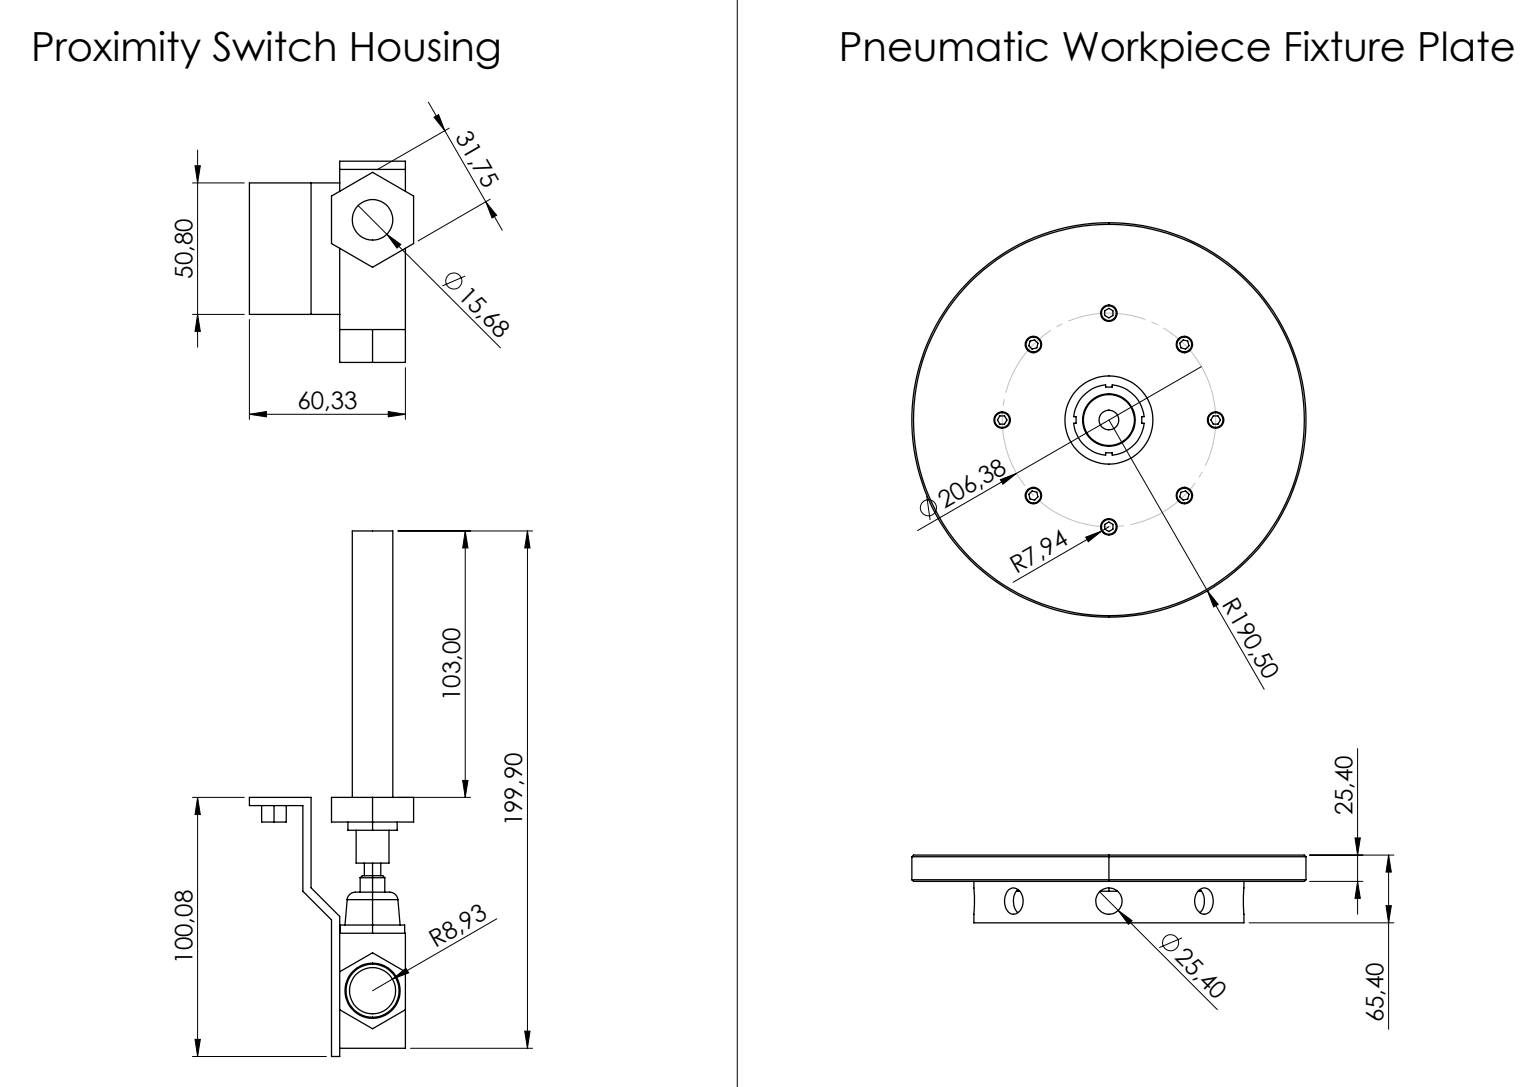
ISO-10303-21;
HEADER;
FILE_DESCRIPTION (('STEP AP214'),
    '1' );
FILE_NAME ('Pneumatic Workpiece Fixture Plate.step',
    '2026-10-07T11:37:37',
    ( '' ),
    ( '' ),
    'SwSTEP 2.0',
    'SolidWorks 2020',
    '' );
FILE_SCHEMA (( 'AUTOMOTIVE_DESIGN' ));
ENDSEC;

DATA;
#3=CARTESIAN_POINT ( 'NONE',  ( -7.205548786489490269E-13, 127.0000000000000000, 111.1250000000000000 ) ) ;
#11=CARTESIAN_POINT ( 'NONE',  ( 92.31685958143638970, 83.38015080693119785, -74.38497350661467067 ) ) ;
#32=DIRECTION ( 'NONE',  ( 0.2588190451025215166, 0.000000000000000000, -0.9659258262890680902 ) ) ;
#49=ORIENTED_EDGE ( 'NONE', *, *, #34842, .F. ) ;
#61=EDGE_LOOP ( 'NONE', ( #69387, #53740 ) ) ;
#64=ADVANCED_FACE ( 'NONE', ( #72976, #57557 ), #58012, .F. ) ;
#66=ADVANCED_FACE ( 'NONE', ( #65279 ), #44369, .F. ) ;
#91=CARTESIAN_POINT ( 'NONE',  ( -90.24991642302028083, 70.17656663518272353, 94.33976020835999066 ) ) ;
#105=CARTESIAN_POINT ( 'NONE',  ( -3.968750000000754508, 127.0000000000000000, 100.8961411191535973 ) ) ;
#110=CARTESIAN_POINT ( 'NONE',  ( -84.20430400022949868, 76.20343663217360586, -99.77245543246449699 ) ) ;
#111=CARTESIAN_POINT ( 'NONE',  ( -91.81710919847694186, 87.03046781249439334, -75.00112839233729289 ) ) ;
#127=CIRCLE ( 'NONE', #16099, 7.143750000000004263 ) ;
#165=PLANE ( 'NONE',  #8255 ) ;
#167=CARTESIAN_POINT ( 'NONE',  ( -103.1875000000000000, 127.0000000000000000, -1.080832317973422076E-12 ) ) ;
#168=DIRECTION ( 'NONE',  ( 0.000000000000000000, 1.000000000000000000, 0.000000000000000000 ) ) ;
#201=ORIENTED_EDGE ( 'NONE', *, *, #40061, .T. ) ;
#217=CARTESIAN_POINT ( 'NONE',  ( 9.720633968232110273E-16, 127.0000000000000000, -111.1250000000000000 ) ) ;
#218=FACE_OUTER_BOUND ( 'NONE', #6817, .T. ) ;
#237=VECTOR ( 'NONE', #41224, 1000.000000000000114 ) ;
#238=EDGE_CURVE ( 'NONE', #48773, #70137, #68413, .T. ) ;
#253=CARTESIAN_POINT ( 'NONE',  ( 129.9447564289581010, 80.89704698943971550, 12.61967231918858445 ) ) ;
#268=CYLINDRICAL_SURFACE ( 'NONE', #55688, 7.143750000000004263 ) ;
#316=CARTESIAN_POINT ( 'NONE',  ( 89.95943163722039060, 94.84315624882769669, 94.61941200740749025 ) ) ;
#327=AXIS2_PLACEMENT_3D ( 'NONE', #13933, #74815, #67998 ) ;
#328=VECTOR ( 'NONE', #6728, 1000.000000000000114 ) ;
#333=ORIENTED_EDGE ( 'NONE', *, *, #85560, .F. ) ;
#366=DIRECTION ( 'NONE',  ( 0.000000000000000000, 1.000000000000000000, 0.000000000000000000 ) ) ;
#370=ADVANCED_FACE ( 'NONE', ( #49293, #62029 ), #15244, .T. ) ;
#376=FACE_BOUND ( 'NONE', #32605, .T. ) ;
#387=ORIENTED_EDGE ( 'NONE', *, *, #40134, .F. ) ;
#391=CARTESIAN_POINT ( 'NONE',  ( -12.70000000000000107, 82.54999999999999716, 117.8738102209307641 ) ) ;
#428=CARTESIAN_POINT ( 'NONE',  ( -92.26493792250037984, 84.21376545118704371, 74.44936585838431142 ) ) ;
#431=ADVANCED_FACE ( 'NONE', ( #81897 ), #67340, .F. ) ;
#435=CARTESIAN_POINT ( 'NONE',  ( 85.00925061400988625, 69.93366089391891194, -82.64146475440696804 ) ) ;
#492=CARTESIAN_POINT ( 'NONE',  ( -75.10852726169378002, 77.68452076096561143, -91.72954497613109481 ) ) ;
#501=ORIENTED_EDGE ( 'NONE', *, *, #4272, .F. ) ;
#504=CARTESIAN_POINT ( 'NONE',  ( 85.31568053864954493, 74.16976894168004719, -98.82395782888116287 ) ) ;
#513=LINE ( 'NONE', #48640, #59500 ) ;
#514=CARTESIAN_POINT ( 'NONE',  ( 0.000000000000000000, 117.4749999999999943, -103.1875000000000000 ) ) ;
#520=FACE_OUTER_BOUND ( 'NONE', #29437, .T. ) ;
#547=ORIENTED_EDGE ( 'NONE', *, *, #56743, .F. ) ;
#575=CARTESIAN_POINT ( 'NONE',  ( -7.941868552260229762E-13, 127.0000000000000000, 107.7702177616926065 ) ) ;
#586=DIRECTION ( 'NONE',  ( -0.8660254037844381525, 0.000000000000000000, -0.5000000000000007772 ) ) ;
#607=CARTESIAN_POINT ( 'NONE',  ( -7.746062721843856025, 92.64813751154241572, 130.3278237768880672 ) ) ;
#621=CARTESIAN_POINT ( 'NONE',  ( 129.9528072873947053, 84.62817240485476589, 12.53569626682358695 ) ) ;
#634=CARTESIAN_POINT ( 'NONE',  ( -80.88709205069390862, 70.52090377575432001, 86.67734222162562219 ) ) ;
#657=CARTESIAN_POINT ( 'NONE',  ( -97.63858630140161665, 92.64237678566784950, -86.67213519546656642 ) ) ;
#673=ORIENTED_EDGE ( 'NONE', *, *, #65969, .T. ) ;
#678=CARTESIAN_POINT ( 'NONE',  ( 72.96458098368650269, 127.0000000000000000, 65.02708098368729850 ) ) ;
#698=ORIENTED_EDGE ( 'NONE', *, *, #71843, .F. ) ;
#711=CARTESIAN_POINT ( 'NONE',  ( 103.1875000000000000, 127.0000000000000000, -7.937499999999639400 ) ) ;
#717=CARTESIAN_POINT ( 'NONE',  ( 103.1875000000000000, 117.4749999999999943, 7.937500000000360600 ) ) ;
#740=ORIENTED_EDGE ( 'NONE', *, *, #36493, .T. ) ;
#755=ADVANCED_FACE ( 'NONE', ( #10935 ), #56167, .T. ) ;
#762=CARTESIAN_POINT ( 'NONE',  ( 85.30153658290296903, 90.93932679090998761, 98.83759631548571178 ) ) ;
#765=CYLINDRICAL_SURFACE ( 'NONE', #44229, 34.13125000000000142 ) ;
#769=EDGE_CURVE ( 'NONE', #62133, #32868, #1079, .T. ) ;
#785=ORIENTED_EDGE ( 'NONE', *, *, #8187, .F. ) ;
#789=CARTESIAN_POINT ( 'NONE',  ( 1.145694247088684285E-22, 95.25000000000000000, 118.5560000000000116 ) ) ;
#827=FACE_OUTER_BOUND ( 'NONE', #18181, .T. ) ;
#841=CARTESIAN_POINT ( 'NONE',  ( 100.8594679592200833, 82.54999999999999716, 82.89895571708400723 ) ) ;
#847=EDGE_LOOP ( 'NONE', ( #47913, #48812, #20485, #2433, #41329, #27512, #86444, #59413, #54279, #89920 ) ) ;
#871=DIRECTION ( 'NONE',  ( 0.7071067811865461294, 0.000000000000000000, 0.7071067811865489050 ) ) ;
#875=PLANE ( 'NONE',  #44348 ) ;
#880=CARTESIAN_POINT ( 'NONE',  ( -79.76397050720386517, 93.94641470820118911, 87.71185091857950056 ) ) ;
#883=ADVANCED_FACE ( 'NONE', ( #13270 ), #75941, .F. ) ;
#886=CARTESIAN_POINT ( 'NONE',  ( -118.0434137139726118, 88.91291927174616205, 11.02232302911455264 ) ) ;
#889=CARTESIAN_POINT ( 'NONE',  ( 74.70173812346097009, 79.26437155269050550, -92.06079644778149884 ) ) ;
#892=DIRECTION ( 'NONE',  ( -3.491483361109385222E-15, 0.000000000000000000, 1.000000000000000000 ) ) ;
#901=CARTESIAN_POINT ( 'NONE',  ( -3.968750000000770051, 127.0000000000000000, 105.4788588808462038 ) ) ;
#905=CARTESIAN_POINT ( 'NONE',  ( 76.80574412431069220, 90.93089219781636245, -90.31319802837579402 ) ) ;
#937=DIRECTION ( 'NONE',  ( 0.000000000000000000, 0.000000000000000000, 1.000000000000000000 ) ) ;
#945=CARTESIAN_POINT ( 'NONE',  ( -76.79083731950203173, 74.16215221268210200, -90.32738470895317562 ) ) ;
#951=CARTESIAN_POINT ( 'NONE',  ( 0.000000000000000000, 111.1250000000000000, 0.000000000000000000 ) ) ;
#954=ORIENTED_EDGE ( 'NONE', *, *, #47098, .T. ) ;
#957=CARTESIAN_POINT ( 'NONE',  ( 87.44698480207823366, 71.76234181793741129, -96.94335780202294472 ) ) ;
#968=CIRCLE ( 'NONE', #16988, 7.143750000000004263 ) ;
#972=CARTESIAN_POINT ( 'NONE',  ( 97.46300000000010755, 82.54999999999999716, -12.69999999999898144 ) ) ;
#985=CARTESIAN_POINT ( 'NONE',  ( -93.49502539975199511, 69.93364840292896645, 91.12742965731035838 ) ) ;
#996=CYLINDRICAL_SURFACE ( 'NONE', #75479, 7.143749999999999822 ) ;
#1018=B_SPLINE_CURVE_WITH_KNOTS ( 'NONE', 3,
 ( #43540, #14059, #62654, #428, #76288, #35382, #57168, #8604, #77636, #56725, #28117, #43086, #41741, #71282, #64450, #70369, #55805, #83560, #36302, #48997, #42634, #21786, #63552, #64010, #70829, #1788, #14519, #22685, #36751, #29485, #35836, #880, #2231, #56264, #29040, #21326, #84471, #50355, #29941, #1338, #42197, #69928, #8145, #84011, #77195, #22234, #69478, #78094, #57625 ),
 .UNSPECIFIED., .F., .F.,
 ( 4, 2, 2, 2, 2, 2, 2, 2, 2, 2, 2, 2, 2, 2, 2, 1, 2, 2, 2, 2, 2, 2, 2, 2, 4 ),
 ( 0.01987186023414422645, 0.02111356671950567407, 0.02235527320486711822, 0.02483868617559002040, 0.02608039266095149578, 0.02732209914631297809, 0.02980551211703592190, 0.03228892508775886572, 0.03353063157312033415, 0.03477233805848178871, 0.03725575102920469783, 0.03849745751456615239, 0.03973916399992760695, 0.04222257697065050913, 0.04346428345601198451, 0.04470598994137346682, 0.04594769642673494914, 0.04718940291209643145, 0.04967281588281940996, 0.05091452236818086452, 0.05215622885354231908, 0.05463964182426526983, 0.05588134830962676602, 0.05712305479498826222, 0.05960646776571128236 ),
 .UNSPECIFIED. ) ;
#1028=ORIENTED_EDGE ( 'NONE', *, *, #76526, .F. ) ;
#1034=ORIENTED_EDGE ( 'NONE', *, *, #40096, .F. ) ;
#1036=DIRECTION ( 'NONE',  ( 0.2588190451025180749, 0.000000000000000000, -0.9659258262890690894 ) ) ;
#1042=VECTOR ( 'NONE', #24862, 1000.000000000000000 ) ;
#1053=ORIENTED_EDGE ( 'NONE', *, *, #85400, .T. ) ;
#1056=DIRECTION ( 'NONE',  ( 0.000000000000000000, -1.000000000000000000, 0.000000000000000000 ) ) ;
#1063=CARTESIAN_POINT ( 'NONE',  ( 12.53573128184445551, 84.62794568765841063, -117.8914214560859932 ) ) ;
#1064=CARTESIAN_POINT ( 'NONE',  ( -12.70000000000000107, 82.54999999999999716, 129.9368274816650910 ) ) ;
#1065=CARTESIAN_POINT ( 'NONE',  ( -3.174999999999644995, 104.3431970271541616, -33.98325472291465132 ) ) ;
#1079=CIRCLE ( 'NONE', #5432, 7.143750000000001599 ) ;
#1082=DIRECTION ( 'NONE',  ( 0.000000000000000000, 1.000000000000000000, 0.000000000000000000 ) ) ;
#1094=CARTESIAN_POINT ( 'NONE',  ( -85.00925061400930360, 69.93366089391888352, 82.64146475440757911 ) ) ;
#1104=CARTESIAN_POINT ( 'NONE',  ( -76.20505178924449297, 127.0000000000000000, 76.20505178924310030 ) ) ;
#1118=CARTESIAN_POINT ( 'NONE',  ( -96.94208673522986430, 93.33885111288434189, -87.44839512528828607 ) ) ;
#1130=ORIENTED_EDGE ( 'NONE', *, *, #23416, .T. ) ;
#1158=LINE ( 'NONE', #36120, #6583 ) ;
#1159=PLANE ( 'NONE',  #88725 ) ;
#1165=AXIS2_PLACEMENT_3D ( 'NONE', #18310, #30611, #59188 ) ;
#1168=EDGE_CURVE ( 'NONE', #65321, #37445, #68012, .T. ) ;
#1178=DIRECTION ( 'NONE',  ( -0.000000000000000000, 1.000000000000000000, 0.000000000000000000 ) ) ;
#1181=DIRECTION ( 'NONE',  ( 0.000000000000000000, -1.000000000000000000, 0.000000000000000000 ) ) ;
#1201=EDGE_LOOP ( 'NONE', ( #30232, #45202 ) ) ;
#1213=EDGE_CURVE ( 'NONE', #59215, #59751, #18967, .T. ) ;
#1220=ORIENTED_EDGE ( 'NONE', *, *, #26232, .F. ) ;
#1222=CARTESIAN_POINT ( 'NONE',  ( 0.000000000000000000, 101.5999999999999943, 0.000000000000000000 ) ) ;
#1225=CARTESIAN_POINT ( 'NONE',  ( 97.63858630140103401, 92.64237678566784950, 86.67213519546724854 ) ) ;
#1241=VERTEX_POINT ( 'NONE', #61630 ) ;
#1245=EDGE_LOOP ( 'NONE', ( #56958, #54258, #46238, #1220 ) ) ;
#1251=ORIENTED_EDGE ( 'NONE', *, *, #68598, .T. ) ;
#1254=ORIENTED_EDGE ( 'NONE', *, *, #34297, .F. ) ;
#1326=DIRECTION ( 'NONE',  ( -0.7071067811865487940, 0.000000000000000000, 0.7071067811865463515 ) ) ;
#1327=EDGE_CURVE ( 'NONE', #9843, #1981, #60064, .T. ) ;
#1332=FACE_BOUND ( 'NONE', #25903, .T. ) ;
#1335=AXIS2_PLACEMENT_3D ( 'NONE', #83746, #42825, #63746 ) ;
#1338=CARTESIAN_POINT ( 'NONE',  ( -76.20774946062844890, 89.94786999841842601, 90.81826664112044512 ) ) ;
#1341=CARTESIAN_POINT ( 'NONE',  ( -117.8827734314469069, 84.21498941703525531, 12.61757617297219802 ) ) ;
#1344=CARTESIAN_POINT ( 'NONE',  ( 81.46681417397508085, 70.27900073646854651, -86.13269706310863683 ) ) ;
#1381=EDGE_LOOP ( 'NONE', ( #14389, #45601, #45690, #35665 ) ) ;
#1414=EDGE_CURVE ( 'NONE', #50785, #8401, #18401, .T. ) ;
#1416=CARTESIAN_POINT ( 'NONE',  ( 93.49502539975264881, 69.93364840292898066, -91.12742965730970468 ) ) ;
#1417=CARTESIAN_POINT ( 'NONE',  ( 0.000000000000000000, 61.59999999999999432, 130.5560000000000116 ) ) ;
#1434=ORIENTED_EDGE ( 'NONE', *, *, #81091, .F. ) ;
#1452=CARTESIAN_POINT ( 'NONE',  ( 3.175000000000355094, 111.1250000000000000, -33.98325472291460159 ) ) ;
#1466=CARTESIAN_POINT ( 'NONE',  ( -83.54193218351851158, 95.25015226514365452, -84.12159398442685188 ) ) ;
#1488=ORIENTED_EDGE ( 'NONE', *, *, #52165, .T. ) ;
#1494=EDGE_CURVE ( 'NONE', #29444, #6827, #10263, .T. ) ;
#1499=CARTESIAN_POINT ( 'NONE',  ( -12.70000000000000107, 82.54999999999999716, 129.9368274816650910 ) ) ;
#1501=ORIENTED_EDGE ( 'NONE', *, *, #74747, .T. ) ;
#1519=CARTESIAN_POINT ( 'NONE',  ( 69.72411017813010403, 120.6499999999999915, -69.72411017812979139 ) ) ;
#1525=DIRECTION ( 'NONE',  ( -1.047445008332813989E-14, 0.000000000000000000, 1.000000000000000000 ) ) ;
#1566=CARTESIAN_POINT ( 'NONE',  ( -100.8961411191535973, 127.0000000000000000, 3.968749999998880451 ) ) ;
#1592=LINE ( 'NONE', #8403, #57970 ) ;
#1606=VECTOR ( 'NONE', #41005, 1000.000000000000114 ) ;
#1610=ADVANCED_FACE ( 'NONE', ( #39738 ), #81397, .T. ) ;
#1621=EDGE_CURVE ( 'NONE', #77970, #1241, #49387, .T. ) ;
#1635=CYLINDRICAL_SURFACE ( 'NONE', #36468, 12.70000000000000107 ) ;
#1657=DIRECTION ( 'NONE',  ( -0.7071067811865510144, 0.000000000000000000, 0.7071067811865441310 ) ) ;
#1659=ORIENTED_EDGE ( 'NONE', *, *, #58078, .F. ) ;
#1670=VERTEX_POINT ( 'NONE', #2002 ) ;
#1676=CARTESIAN_POINT ( 'NONE',  ( 98.60478223830740774, 127.0000000000000000, 3.859079674607175002E-13 ) ) ;
#1677=CARTESIAN_POINT ( 'NONE',  ( 82.89895571708159139, 82.96445444011520465, 100.8594679592221155 ) ) ;
#1683=LINE ( 'NONE', #15759, #75101 ) ;
#1685=CARTESIAN_POINT ( 'NONE',  ( 76.20505178924339873, 120.6499999999999915, 76.20505178924419454 ) ) ;
#1691=ORIENTED_EDGE ( 'NONE', *, *, #2750, .F. ) ;
#1702=ORIENTED_EDGE ( 'NONE', *, *, #76963, .T. ) ;
#1704=VERTEX_POINT ( 'NONE', #84243 ) ;
#1724=ORIENTED_EDGE ( 'NONE', *, *, #1621, .T. ) ;
#1725=DIRECTION ( 'NONE',  ( -3.491483361109380094E-15, 0.000000000000000000, 1.000000000000000000 ) ) ;
#1734=FACE_BOUND ( 'NONE', #62684, .T. ) ;
#1751=CARTESIAN_POINT ( 'NONE',  ( -7.205548786489490269E-13, 101.5999999999999943, 103.1875000000000000 ) ) ;
#1764=CARTESIAN_POINT ( 'NONE',  ( 90.65754775987920766, 74.81620433377381119, 76.39898589339244950 ) ) ;
#1765=PLANE ( 'NONE',  #84930 ) ;
#1766=ADVANCED_FACE ( 'NONE', ( #83332 ), #76511, .F. ) ;
#1782=ORIENTED_EDGE ( 'NONE', *, *, #57519, .F. ) ;
#1786=ORIENTED_EDGE ( 'NONE', *, *, #238, .F. ) ;
#1788=CARTESIAN_POINT ( 'NONE',  ( -83.24211534968669923, 95.24969287062863543, 84.42134122279109931 ) ) ;
#1794=VERTEX_POINT ( 'NONE', #76962 ) ;
#1813=CARTESIAN_POINT ( 'NONE',  ( 72.96458098368701428, 101.5999999999999943, -78.00648098368678518 ) ) ;
#1817=ORIENTED_EDGE ( 'NONE', *, *, #32049, .F. ) ;
#1828=AXIS2_PLACEMENT_3D ( 'NONE', #54145, #81016, #19216 ) ;
#1850=CARTESIAN_POINT ( 'NONE',  ( 72.96458098368701428, 117.4749999999999943, -65.02708098368670164 ) ) ;
#1856=CARTESIAN_POINT ( 'NONE',  ( -103.1875000000000000, 127.0000000000000000, -1.080832317973422076E-12 ) ) ;
#1872=FACE_BOUND ( 'NONE', #82136, .T. ) ;
#1887=ORIENTED_EDGE ( 'NONE', *, *, #8187, .T. ) ;
#1895=AXIS2_PLACEMENT_3D ( 'NONE', #16774, #79005, #44455 ) ;
#1915=ORIENTED_EDGE ( 'NONE', *, *, #61465, .T. ) ;
#1945=ORIENTED_EDGE ( 'NONE', *, *, #81206, .T. ) ;
#1946=EDGE_CURVE ( 'NONE', #1794, #35668, #24234, .T. ) ;
#1954=FACE_BOUND ( 'NONE', #72816, .T. ) ;
#1967=CARTESIAN_POINT ( 'NONE',  ( -10.78734560828563360, 89.26522093196130925, 130.1097824653510315 ) ) ;
#1981=VERTEX_POINT ( 'NONE', #16527 ) ;
#2002=CARTESIAN_POINT ( 'NONE',  ( 4.665904304751420031E-15, 92.07499999999998863, -38.10000000000000142 ) ) ;
#2015=CARTESIAN_POINT ( 'NONE',  ( 1.668880554893940493, 69.93234144696143062, 130.5479136978233896 ) ) ;
#2023=CIRCLE ( 'NONE', #41097, 38.10000000000000142 ) ;
#2033=CARTESIAN_POINT ( 'NONE',  ( -103.1875000000000000, 117.4749999999999943, -1.080832317973422076E-12 ) ) ;
#2043=EDGE_LOOP ( 'NONE', ( #68408, #37115, #73877, #16147 ) ) ;
#2059=CARTESIAN_POINT ( 'NONE',  ( -130.4793906290846621, 70.66229531820916065, -4.488385961153167791 ) ) ;
#2062=VERTEX_POINT ( 'NONE', #26903 ) ;
#2090=PLANE ( 'NONE',  #6152 ) ;
#2098=DIRECTION ( 'NONE',  ( 0.000000000000000000, 1.000000000000000000, 0.000000000000000000 ) ) ;
#2102=LINE ( 'NONE', #28917, #67367 ) ;
#2124=EDGE_CURVE ( 'NONE', #47880, #64107, #46324, .T. ) ;
#2161=FACE_BOUND ( 'NONE', #29161, .T. ) ;
#2166=ORIENTED_EDGE ( 'NONE', *, *, #69271, .T. ) ;
#2184=VECTOR ( 'NONE', #82406, 1000.000000000000114 ) ;
#2192=LINE ( 'NONE', #83973, #66848 ) ;
#2221=EDGE_CURVE ( 'NONE', #55274, #46818, #44913, .T. ) ;
#2231=CARTESIAN_POINT ( 'NONE',  ( -79.21949419058834962, 93.55466788070657458, 88.20392011030202184 ) ) ;
#2249=VECTOR ( 'NONE', #61719, 1000.000000000000000 ) ;
#2290=FACE_OUTER_BOUND ( 'NONE', #53030, .T. ) ;
#2305=CARTESIAN_POINT ( 'NONE',  ( 0.000000000000000000, 127.0000000000000000, 0.000000000000000000 ) ) ;
#2315=CARTESIAN_POINT ( 'NONE',  ( 0.000000000000000000, 117.4749999999999943, -98.14560000000000173 ) ) ;
#2330=LINE ( 'NONE', #23675, #16717 ) ;
#2338=ADVANCED_FACE ( 'NONE', ( #56834 ), #996, .T. ) ;
#2352=EDGE_CURVE ( 'NONE', #18286, #38056, #51216, .T. ) ;
#2354=DIRECTION ( 'NONE',  ( 0.000000000000000000, 1.000000000000000000, 0.000000000000000000 ) ) ;
#2365=ORIENTED_EDGE ( 'NONE', *, *, #71733, .T. ) ;
#2387=CARTESIAN_POINT ( 'NONE',  ( 76.20505178924389611, 120.6499999999999915, -76.20505178924359768 ) ) ;
#2389=ADVANCED_FACE ( 'NONE', ( #87244 ), #10927, .F. ) ;
#2396=VERTEX_POINT ( 'NONE', #53574 ) ;
#2424=CARTESIAN_POINT ( 'NONE',  ( 0.000000000000000000, 127.0000000000000000, 0.000000000000000000 ) ) ;
#2431=VERTEX_POINT ( 'NONE', #19529 ) ;
#2432=LINE ( 'NONE', #50105, #73729 ) ;
#2433=ORIENTED_EDGE ( 'NONE', *, *, #81943, .F. ) ;
#2442=EDGE_CURVE ( 'NONE', #6249, #50785, #59903, .T. ) ;
#2444=CARTESIAN_POINT ( 'NONE',  ( -7.199374239792870816E-13, 101.5999999999999943, 98.14560000000000173 ) ) ;
#2453=DIRECTION ( 'NONE',  ( 0.000000000000000000, 1.000000000000000000, 0.000000000000000000 ) ) ;
#2455=DIRECTION ( 'NONE',  ( 0.000000000000000000, -1.000000000000000000, 0.000000000000000000 ) ) ;
#2456=CARTESIAN_POINT ( 'NONE',  ( -72.96458098368600531, 127.0000000000000000, -67.92268098368781182 ) ) ;
#2486=ORIENTED_EDGE ( 'NONE', *, *, #31297, .F. ) ;
#2487=AXIS2_PLACEMENT_3D ( 'NONE', #78848, #86101, #15719 ) ;
#2507=CARTESIAN_POINT ( 'NONE',  ( -130.2871811975775813, 72.98383416765817344, 8.394281761909056172 ) ) ;
#2514=EDGE_CURVE ( 'NONE', #12810, #44525, #54917, .T. ) ;
#2544=VERTEX_POINT ( 'NONE', #49909 ) ;
#2552=CARTESIAN_POINT ( 'NONE',  ( -12.70000000000000107, 82.54999999999999716, -129.9368274816650910 ) ) ;
#2564=AXIS2_PLACEMENT_3D ( 'NONE', #83197, #46395, #47297 ) ;
#2589=CARTESIAN_POINT ( 'NONE',  ( -72.96458098368600531, 117.4749999999999943, -72.96458098368781009 ) ) ;
#2596=VECTOR ( 'NONE', #70871, 1000.000000000000114 ) ;
#2609=FACE_BOUND ( 'NONE', #21078, .T. ) ;
#2611=DIRECTION ( 'NONE',  ( 1.000000000000000000, 0.000000000000000000, 0.000000000000000000 ) ) ;
#2615=CARTESIAN_POINT ( 'NONE',  ( -7.205548786489490269E-13, 127.0000000000000000, 103.1875000000000000 ) ) ;
#2616=VERTEX_POINT ( 'NONE', #86241 ) ;
#2623=ADVANCED_FACE ( 'NONE', ( #24020 ), #36754, .T. ) ;
#2631=CARTESIAN_POINT ( 'NONE',  ( 74.15067561874209900, 120.6499999999999915, 68.53801554307469246 ) ) ;
#2664=CARTESIAN_POINT ( 'NONE',  ( 75.68572508987453773, 76.20320268897035021, 91.25368348339081592 ) ) ;
#2679=ADVANCED_FACE ( 'NONE', ( #53006 ), #52128, .F. ) ;
#2684=DIRECTION ( 'NONE',  ( 0.000000000000000000, 0.000000000000000000, -1.000000000000000000 ) ) ;
#2698=EDGE_CURVE ( 'NONE', #82109, #43994, #17645, .T. ) ;
#2725=LINE ( 'NONE', #42681, #24433 ) ;
#2743=ORIENTED_EDGE ( 'NONE', *, *, #61260, .F. ) ;
#2750=EDGE_CURVE ( 'NONE', #52484, #27146, #59495, .T. ) ;
#2766=CARTESIAN_POINT ( 'NONE',  ( 99.76704648670056486, 88.91113633199481114, -84.21071524772746386 ) ) ;
#2768=VECTOR ( 'NONE', #53000, 1000.000000000000000 ) ;
#2788=EDGE_LOOP ( 'NONE', ( #36538, #22888, #1028, #17291 ) ) ;
#2794=CARTESIAN_POINT ( 'NONE',  ( -96.94152442043684914, 93.33921197991993779, 87.44900557253197348 ) ) ;
#2798=DIRECTION ( 'NONE',  ( 0.000000000000000000, 1.000000000000000000, 0.000000000000000000 ) ) ;
#2812=ORIENTED_EDGE ( 'NONE', *, *, #86456, .T. ) ;
#2816=VERTEX_POINT ( 'NONE', #13071 ) ;
#2831=LINE ( 'NONE', #35997, #27075 ) ;
#2841=CARTESIAN_POINT ( 'NONE',  ( -2.883802008152356322, 70.17481864577712258, 130.5247784292598112 ) ) ;
#2846=ORIENTED_EDGE ( 'NONE', *, *, #21323, .F. ) ;
#2849=DIRECTION ( 'NONE',  ( 0.000000000000000000, 1.000000000000000000, 0.000000000000000000 ) ) ;
#2902=CARTESIAN_POINT ( 'NONE',  ( 118.1268077877470830, 74.81620433377382540, -10.08232578576091854 ) ) ;
#2905=DIRECTION ( 'NONE',  ( 0.000000000000000000, -0.7071067811865280328, -0.7071067811865670016 ) ) ;
#2948=CARTESIAN_POINT ( 'NONE',  ( -130.3273007233323142, 72.45841406287408404, 7.755409066832052112 ) ) ;
#2970=ORIENTED_EDGE ( 'NONE', *, *, #89696, .F. ) ;
#2988=CARTESIAN_POINT ( 'NONE',  ( -11.89044713366393680, 87.03112570152840988, -130.0135071244502853 ) ) ;
#2992=AXIS2_PLACEMENT_3D ( 'NONE', #72250, #50897, #44516 ) ;
#2999=EDGE_LOOP ( 'NONE', ( #63002, #56856, #5047, #17409, #54291, #77223, #34139, #34652, #30607, #29751, #12971, #71726, #7525, #26455, #29483, #22789 ) ) ;
#3002=CARTESIAN_POINT ( 'NONE',  ( 0.000000000000000000, 101.5999999999999943, -103.1875000000000000 ) ) ;
#3009=CARTESIAN_POINT ( 'NONE',  ( 74.38497350661437224, 83.38015080693121206, 92.31685958143667392 ) ) ;
#3012=CARTESIAN_POINT ( 'NONE',  ( 7.752238106858494682, 92.64409645872694909, 130.3274943305225122 ) ) ;
#3016=ADVANCED_FACE ( 'NONE', ( #3796, #52787 ), #80554, .F. ) ;
#3019=VECTOR ( 'NONE', #47360, 1000.000000000000000 ) ;
#3025=VECTOR ( 'NONE', #19725, 1000.000000000000000 ) ;
#3027=EDGE_LOOP ( 'NONE', ( #48707, #4492, #67828, #78131, #34277, #73610 ) ) ;
#3056=VERTEX_POINT ( 'NONE', #66910 ) ;
#3072=CIRCLE ( 'NONE', #33470, 42.54500000000000171 ) ;
#3098=CARTESIAN_POINT ( 'NONE',  ( -69.72411017813060141, 120.6499999999999915, 69.72411017812929401 ) ) ;
#3101=CARTESIAN_POINT ( 'NONE',  ( 89.13771950014249512, 72.45860812971086773, 78.16952835488777396 ) ) ;
#3118=ORIENTED_EDGE ( 'NONE', *, *, #26315, .F. ) ;
#3119=LINE ( 'NONE', #37644, #65548 ) ;
#3149=ORIENTED_EDGE ( 'NONE', *, *, #11965, .F. ) ;
#3183=ORIENTED_EDGE ( 'NONE', *, *, #68690, .F. ) ;
#3189=EDGE_LOOP ( 'NONE', ( #71067, #73722, #49504, #27268 ) ) ;
#3208=CARTESIAN_POINT ( 'NONE',  ( 100.8465607796070742, 83.38002811471481834, -82.91466710319141953 ) ) ;
#3212=VECTOR ( 'NONE', #50264, 1000.000000000000000 ) ;
#3215=DIRECTION ( 'NONE',  ( 0.000000000000000000, 1.000000000000000000, 0.000000000000000000 ) ) ;
#3226=ORIENTED_EDGE ( 'NONE', *, *, #41674, .F. ) ;
#3236=CARTESIAN_POINT ( 'NONE',  ( -95.16331303980125256, 94.60320878023493663, 89.38347482486680917 ) ) ;
#3242=LINE ( 'NONE', #37310, #40634 ) ;
#3254=CARTESIAN_POINT ( 'NONE',  ( 0.000000000000000000, 124.5870000000000033, 0.000000000000000000 ) ) ;
#3286=CARTESIAN_POINT ( 'NONE',  ( -11.39831192919941927, 76.93384533283848725, 130.0576265831481635 ) ) ;
#3295=DIRECTION ( 'NONE',  ( -0.000000000000000000, 1.000000000000000000, -0.000000000000000000 ) ) ;
#3296=ORIENTED_EDGE ( 'NONE', *, *, #51682, .F. ) ;
#3325=CARTESIAN_POINT ( 'NONE',  ( 1.598849875094818280E-14, 101.5999999999999943, -130.5560000000000116 ) ) ;
#3327=CARTESIAN_POINT ( 'NONE',  ( 107.7702177616926065, 120.6499999999999915, 4.179089330879380409E-13 ) ) ;
#3345=CARTESIAN_POINT ( 'NONE',  ( 117.8738102209308920, 82.54999999999999716, -12.69999999999876827 ) ) ;
#3350=DIRECTION ( 'NONE',  ( -0.000000000000000000, 1.000000000000000000, 0.000000000000000000 ) ) ;
#3352=EDGE_CURVE ( 'NONE', #66793, #76220, #23706, .T. ) ;
#3355=ADVANCED_FACE ( 'NONE', ( #71408 ), #38206, .T. ) ;
#3360=VECTOR ( 'NONE', #83469, 1000.000000000000000 ) ;
#3366=VERTEX_POINT ( 'NONE', #59074 ) ;
#3390=CARTESIAN_POINT ( 'NONE',  ( -129.9778716492873230, 79.25971567868511158, -12.27341459163442039 ) ) ;
#3435=DIRECTION ( 'NONE',  ( 0.000000000000000000, 0.000000000000000000, 1.000000000000000000 ) ) ;
#3457=CARTESIAN_POINT ( 'NONE',  ( 1.653891986036727157, 95.16955141394545592, 130.5480982590283929 ) ) ;
#3469=ORIENTED_EDGE ( 'NONE', *, *, #88264, .F. ) ;
#3475=CARTESIAN_POINT ( 'NONE',  ( 68.53801554307449351, 120.6499999999999915, -74.15067561874229796 ) ) ;
#3532=DIRECTION ( 'NONE',  ( 0.000000000000000000, 1.000000000000000000, 0.000000000000000000 ) ) ;
#3549=CARTESIAN_POINT ( 'NONE',  ( 118.2605848834651425, 92.12496802699139664, 8.385272115322319308 ) ) ;
#3563=ORIENTED_EDGE ( 'NONE', *, *, #4315, .F. ) ;
#3565=EDGE_CURVE ( 'NONE', #43245, #5020, #52687, .T. ) ;
#3582=CARTESIAN_POINT ( 'NONE',  ( -3.174999999999644995, 124.5870000000000033, -33.98325472291465132 ) ) ;
#3584=ORIENTED_EDGE ( 'NONE', *, *, #49359, .F. ) ;
#3592=DIRECTION ( 'NONE',  ( 0.000000000000000000, -1.000000000000000000, 0.000000000000000000 ) ) ;
#3615=ORIENTED_EDGE ( 'NONE', *, *, #62505, .F. ) ;
#3617=ORIENTED_EDGE ( 'NONE', *, *, #17476, .F. ) ;
#3633=DIRECTION ( 'NONE',  ( 1.000000000000000000, 0.000000000000000000, 0.000000000000000000 ) ) ;
#3664=EDGE_CURVE ( 'NONE', #76633, #10599, #23030, .T. ) ;
#3673=CARTESIAN_POINT ( 'NONE',  ( -100.0213216842699779, 88.17609398443094904, 83.90854149456468747 ) ) ;
#3678=CARTESIAN_POINT ( 'NONE',  ( -74.15067561874160162, 120.6499999999999915, -68.53801554307528932 ) ) ;
#3680=EDGE_LOOP ( 'NONE', ( #75447, #6355, #76872, #82445 ) ) ;
#3688=CARTESIAN_POINT ( 'NONE',  ( 77.39114642429960611, 127.0000000000000000, -71.77848634863110533 ) ) ;
#3693=ORIENTED_EDGE ( 'NONE', *, *, #61802, .F. ) ;
#3715=DIRECTION ( 'NONE',  ( 0.000000000000000000, 1.000000000000000000, 0.000000000000000000 ) ) ;
#3726=ORIENTED_EDGE ( 'NONE', *, *, #57993, .F. ) ;
#3745=EDGE_CURVE ( 'NONE', #37737, #2431, #35401, .T. ) ;
#3758=ORIENTED_EDGE ( 'NONE', *, *, #77992, .T. ) ;
#3785=DIRECTION ( 'NONE',  ( 0.000000000000000000, 1.000000000000000000, 0.000000000000000000 ) ) ;
#3787=CARTESIAN_POINT ( 'NONE',  ( 117.9189190431816172, 79.26437155269050550, -12.27470785613960835 ) ) ;
#3796=FACE_BOUND ( 'NONE', #78200, .T. ) ;
#3804=FACE_OUTER_BOUND ( 'NONE', #54938, .T. ) ;
#3809=DIRECTION ( 'NONE',  ( 0.000000000000000000, 0.000000000000000000, -1.000000000000000000 ) ) ;
#3815=CARTESIAN_POINT ( 'NONE',  ( -74.15067561874160162, 120.6499999999999915, -68.53801554307528932 ) ) ;
#3876=CARTESIAN_POINT ( 'NONE',  ( -3.174999999999664979, 111.1250000000000000, -31.75000000000000000 ) ) ;
#3894=CARTESIAN_POINT ( 'NONE',  ( 0.000000000000000000, 117.4749999999999943, -110.3312500000000114 ) ) ;
#3898=CARTESIAN_POINT ( 'NONE',  ( 3.291704278000434414, 94.82304653311919651, 130.5151038487541939 ) ) ;
#3907=EDGE_CURVE ( 'NONE', #66196, #3366, #89475, .T. ) ;
#3920=PLANE ( 'NONE',  #88005 ) ;
#3921=VERTEX_POINT ( 'NONE', #72181 ) ;
#3934=ORIENTED_EDGE ( 'NONE', *, *, #14312, .F. ) ;
#3964=EDGE_CURVE ( 'NONE', #57201, #18286, #79002, .T. ) ;
#3968=VECTOR ( 'NONE', #26272, 1000.000000000000000 ) ;
#3985=LINE ( 'NONE', #85345, #68695 ) ;
#3990=VERTEX_POINT ( 'NONE', #30841 ) ;
#3997=CARTESIAN_POINT ( 'NONE',  ( 118.5451175586561874, 95.14807216649714405, 1.659552426424649729 ) ) ;
#4026=ORIENTED_EDGE ( 'NONE', *, *, #41664, .F. ) ;
#4032=CARTESIAN_POINT ( 'NONE',  ( -118.1268077877469977, 74.81620433377381119, 10.08232578576174099 ) ) ;
#4066=DIRECTION ( 'NONE',  ( 0.8660254037844379305, 0.000000000000000000, -0.5000000000000011102 ) ) ;
#4083=EDGE_CURVE ( 'NONE', #64107, #47880, #968, .T. ) ;
#4091=CARTESIAN_POINT ( 'NONE',  ( 0.000000000000000000, 127.0000000000000000, 42.54500000000000171 ) ) ;
#4095=ORIENTED_EDGE ( 'NONE', *, *, #9873, .F. ) ;
#4115=CARTESIAN_POINT ( 'NONE',  ( -85.52787878288653189, 91.23859726994542996, 98.64044413063014360 ) ) ;
#4125=DIRECTION ( 'NONE',  ( -0.7071067811865495711, 0.000000000000000000, 0.7071067811865455743 ) ) ;
#4126=EDGE_LOOP ( 'NONE', ( #54924, #32505 ) ) ;
#4150=DIRECTION ( 'NONE',  ( 0.000000000000000000, 0.000000000000000000, 1.000000000000000000 ) ) ;
#4172=CARTESIAN_POINT ( 'NONE',  ( -88.20503424218274802, 71.54629894495528220, -79.21825297796436871 ) ) ;
#4173=EDGE_CURVE ( 'NONE', #40480, #68811, #82455, .T. ) ;
#4205=ORIENTED_EDGE ( 'NONE', *, *, #88673, .F. ) ;
#4210=VERTEX_POINT ( 'NONE', #34406 ) ;
#4219=CARTESIAN_POINT ( 'NONE',  ( -84.91200770515607132, 74.81660785136577374, 99.17101862044627580 ) ) ;
#4230=CARTESIAN_POINT ( 'NONE',  ( 118.1704280561596931, 74.16215221268205937, 9.571784452934572585 ) ) ;
#4252=ORIENTED_EDGE ( 'NONE', *, *, #64976, .T. ) ;
#4255=CARTESIAN_POINT ( 'NONE',  ( -11.00664350276215941, 76.20047485311516766, 118.0441341279204721 ) ) ;
#4262=LINE ( 'NONE', #61007, #47994 ) ;
#4272=EDGE_CURVE ( 'NONE', #60191, #24962, #85893, .T. ) ;
#4279=CARTESIAN_POINT ( 'NONE',  ( -3.968750000000770051, 120.6499999999999915, 105.4788588808462038 ) ) ;
#4281=EDGE_LOOP ( 'NONE', ( #13317, #49329 ) ) ;
#4299=DIRECTION ( 'NONE',  ( 0.000000000000000000, 1.000000000000000000, 0.000000000000000000 ) ) ;
#4305=CARTESIAN_POINT ( 'NONE',  ( -72.96458098368751166, 127.0000000000000000, 65.82083098368619289 ) ) ;
#4315=EDGE_CURVE ( 'NONE', #32905, #16980, #30289, .T. ) ;
#4322=AXIS2_PLACEMENT_3D ( 'NONE', #59666, #74660, #20151 ) ;
#4324=ORIENTED_EDGE ( 'NONE', *, *, #66591, .T. ) ;
#4347=AXIS2_PLACEMENT_3D ( 'NONE', #81002, #52775, #26462 ) ;
#4363=ORIENTED_EDGE ( 'NONE', *, *, #78833, .F. ) ;
#4370=DIRECTION ( 'NONE',  ( -0.000000000000000000, 1.000000000000000000, -0.000000000000000000 ) ) ;
#4380=VERTEX_POINT ( 'NONE', #86599 ) ;
#4387=DIRECTION ( 'NONE',  ( 0.000000000000000000, 1.000000000000000000, 0.000000000000000000 ) ) ;
#4390=DIRECTION ( 'NONE',  ( 0.000000000000000000, 0.000000000000000000, 1.000000000000000000 ) ) ;
#4418=CARTESIAN_POINT ( 'NONE',  ( -74.15067561874160162, 127.0000000000000000, -68.53801554307528932 ) ) ;
#4426=CARTESIAN_POINT ( 'NONE',  ( 11.00078833628932173, 88.90974477516434149, -130.0918550420129236 ) ) ;
#4451=CARTESIAN_POINT ( 'NONE',  ( 118.0074504647926688, 88.17653575778740560, 11.39323553397083444 ) ) ;
#4492=ORIENTED_EDGE ( 'NONE', *, *, #62549, .T. ) ;
#4501=DIRECTION ( 'NONE',  ( 0.000000000000000000, -1.000000000000000000, 0.000000000000000000 ) ) ;
#4506=DIRECTION ( 'NONE',  ( 0.000000000000000000, -1.000000000000000000, 0.000000000000000000 ) ) ;
#4527=CARTESIAN_POINT ( 'NONE',  ( -129.9368274816650626, 82.96445444011519044, -12.70000000000045404 ) ) ;
#4534=EDGE_CURVE ( 'NONE', #66251, #28958, #10722, .T. ) ;
#4543=CARTESIAN_POINT ( 'NONE',  ( -7.205548786489490269E-13, 117.4749999999999943, 103.1875000000000000 ) ) ;
#4546=CARTESIAN_POINT ( 'NONE',  ( -9.275582543403935176, 73.86526018886296185, -118.1929554227103267 ) ) ;
#4559=AXIS2_PLACEMENT_3D ( 'NONE', #7540, #41585, #77475 ) ;
#4564=ORIENTED_EDGE ( 'NONE', *, *, #88178, .F. ) ;
#4569=CARTESIAN_POINT ( 'NONE',  ( -82.89895571708294142, 83.38918798244689867, 100.8594679592209502 ) ) ;
#4586=CONICAL_SURFACE ( 'NONE', #43737, 188.9759999999999991, 0.7853981633974758125 ) ;
#4597=CARTESIAN_POINT ( 'NONE',  ( -68.53801554307339927, 120.6499999999999915, -74.15067561874339219 ) ) ;
#4621=CARTESIAN_POINT ( 'NONE',  ( -92.32962665258507684, 82.54999999999999716, -74.36911441044765070 ) ) ;
#4623=EDGE_LOOP ( 'NONE', ( #58418, #31773 ) ) ;
#4638=CARTESIAN_POINT ( 'NONE',  ( -3.968750000000754508, 120.6499999999999915, 100.8961411191535973 ) ) ;
#4640=CARTESIAN_POINT ( 'NONE',  ( 72.96458098368701428, 117.4749999999999943, -72.96458098368670164 ) ) ;
#4650=EDGE_CURVE ( 'NONE', #68005, #70474, #37848, .T. ) ;
#4655=EDGE_CURVE ( 'NONE', #9197, #63483, #24655, .T. ) ;
#4666=DIRECTION ( 'NONE',  ( 0.000000000000000000, -1.000000000000000000, 0.000000000000000000 ) ) ;
#4682=CARTESIAN_POINT ( 'NONE',  ( 118.2371168503541838, 73.28361289573329884, 8.694557611693589649 ) ) ;
#4687=ORIENTED_EDGE ( 'NONE', *, *, #4920, .F. ) ;
#4691=CARTESIAN_POINT ( 'NONE',  ( -97.63922045723913357, 72.45841406287408404, -86.67141577317428869 ) ) ;
#4694=DIRECTION ( 'NONE',  ( 0.000000000000000000, 1.000000000000000000, 0.000000000000000000 ) ) ;
#4700=ORIENTED_EDGE ( 'NONE', *, *, #62567, .T. ) ;
#4701=VERTEX_POINT ( 'NONE', #59600 ) ;
#4722=CYLINDRICAL_SURFACE ( 'NONE', #51592, 7.937500000000000000 ) ;
#4748=CARTESIAN_POINT ( 'NONE',  ( 3.968750000000050182, 127.0000000000000000, -100.8961411191535973 ) ) ;
#4751=CARTESIAN_POINT ( 'NONE',  ( -12.27452259663393264, 85.83635631587365822, -117.9189384461415813 ) ) ;
#4792=CARTESIAN_POINT ( 'NONE',  ( -68.53801554307499089, 120.6499999999999915, 74.15067561874188584 ) ) ;
#4797=EDGE_CURVE ( 'NONE', #54712, #28958, #8678, .T. ) ;
#4832=DIRECTION ( 'NONE',  ( 0.000000000000000000, 1.000000000000000000, 0.000000000000000000 ) ) ;
#4864=CARTESIAN_POINT ( 'NONE',  ( 12.67977336836082891, 83.37982733273462088, -129.9388093972407603 ) ) ;
#4887=EDGE_CURVE ( 'NONE', #61102, #77844, #81944, .T. ) ;
#4897=VECTOR ( 'NONE', #26224, 1000.000000000000114 ) ;
#4920=EDGE_CURVE ( 'NONE', #40277, #9193, #18341, .T. ) ;
#4928=CARTESIAN_POINT ( 'NONE',  ( -117.9189190431815462, 79.26437155269051971, 12.27470785614043436 ) ) ;
#4949=DIRECTION ( 'NONE',  ( -0.8660254037844390407, 0.000000000000000000, -0.4999999999999995004 ) ) ;
#4964=DIRECTION ( 'NONE',  ( 0.000000000000000000, 1.000000000000000000, 0.000000000000000000 ) ) ;
#4970=CARTESIAN_POINT ( 'NONE',  ( -130.4924867222203773, 94.58014758961631685, 4.091264198876692681 ) ) ;
#4983=CARTESIAN_POINT ( 'NONE',  ( 94.61941200740719182, 94.84315624882772511, -89.95943163722073166 ) ) ;
#4985=CARTESIAN_POINT ( 'NONE',  ( 3.174999999999889688, 124.5870000000000033, 31.75000000000000000 ) ) ;
#5020=VERTEX_POINT ( 'NONE', #64068 ) ;
#5023=VERTEX_POINT ( 'NONE', #49513 ) ;
#5046=CARTESIAN_POINT ( 'NONE',  ( 103.1875000000000000, 117.4749999999999943, 3.602774393244745134E-13 ) ) ;
#5047=ORIENTED_EDGE ( 'NONE', *, *, #43636, .F. ) ;
#5048=CARTESIAN_POINT ( 'NONE',  ( 129.9368274816652331, 83.38918798244689867, -12.69999999999863505 ) ) ;
#5078=( LENGTH_UNIT ( ) NAMED_UNIT ( * ) SI_UNIT ( .MILLI., .METRE. ) );
#5100=CARTESIAN_POINT ( 'NONE',  ( 72.96458098368701428, 127.0000000000000000, -72.96458098368670164 ) ) ;
#5103=EDGE_CURVE ( 'NONE', #58908, #41468, #74447, .T. ) ;
#5123=CARTESIAN_POINT ( 'NONE',  ( 3.968749999999229949, 120.6499999999999915, 100.8961411191535973 ) ) ;
#5131=CARTESIAN_POINT ( 'NONE',  ( -88.24354053934787601, 71.14122173980733521, -96.22129751242513862 ) ) ;
#5145=ORIENTED_EDGE ( 'NONE', *, *, #29847, .T. ) ;
#5152=AXIS2_PLACEMENT_3D ( 'NONE', #84294, #43363, #15236 ) ;
#5164=DIRECTION ( 'NONE',  ( 0.000000000000000000, 1.000000000000000000, 0.000000000000000000 ) ) ;
#5210=AXIS2_PLACEMENT_3D ( 'NONE', #35376, #34934, #21779 ) ;
#5219=DIRECTION ( 'NONE',  ( 0.000000000000000000, 1.000000000000000000, 0.000000000000000000 ) ) ;
#5225=CARTESIAN_POINT ( 'NONE',  ( -75.67519899969657615, 76.18740257834568297, 91.26337341211453236 ) ) ;
#5228=VECTOR ( 'NONE', #47995, 1000.000000000000114 ) ;
#5282=CARTESIAN_POINT ( 'NONE',  ( 130.0566129357926570, 76.91670260214422683, -11.41267162807792168 ) ) ;
#5283=ADVANCED_FACE ( 'NONE', ( #1734, #21732, #77140, #376, #85316, #23089, #14917, #49854, #28517, #827 ), #14467, .F. ) ;
#5297=EDGE_CURVE ( 'NONE', #11982, #19831, #35333, .T. ) ;
#5321=CARTESIAN_POINT ( 'NONE',  ( 3.968749999999215294, 120.6499999999999915, 105.4788588808464027 ) ) ;
#5328=DIRECTION ( 'NONE',  ( 0.000000000000000000, 1.000000000000000000, 0.000000000000000000 ) ) ;
#5341=CARTESIAN_POINT ( 'NONE',  ( 74.15067561874269586, 120.6499999999999915, -68.53801554307419508 ) ) ;
#5343=LINE ( 'NONE', #47550, #70965 ) ;
#5347=CARTESIAN_POINT ( 'NONE',  ( 118.5559670995753407, 95.24969287062864964, -0.8338386114217244405 ) ) ;
#5357=DIRECTION ( 'NONE',  ( -0.7071067811865512365, 0.000000000000000000, 0.7071067811865436870 ) ) ;
#5376=CARTESIAN_POINT ( 'NONE',  ( -118.1931971052175783, 73.86197090048098346, 9.272510012971169502 ) ) ;
#5390=EDGE_LOOP ( 'NONE', ( #42426, #41819, #67161, #56127 ) ) ;
#5393=VECTOR ( 'NONE', #68884, 1000.000000000000000 ) ;
#5396=EDGE_LOOP ( 'NONE', ( #15482, #17028, #56494, #54162 ) ) ;
#5400=VECTOR ( 'NONE', #8620, 1000.000000000000000 ) ;
#5407=ADVANCED_FACE ( 'NONE', ( #30332 ), #17590, .F. ) ;
#5415=VERTEX_POINT ( 'NONE', #85760 ) ;
#5427=CARTESIAN_POINT ( 'NONE',  ( -130.2872239869710143, 92.11674985319542941, 8.393624206580916791 ) ) ;
#5432=AXIS2_PLACEMENT_3D ( 'NONE', #64573, #2354, #4125 ) ;
#5435=PLANE ( 'NONE',  #64452 ) ;
#5439=CARTESIAN_POINT ( 'NONE',  ( 84.19383299529407338, 88.91243380484084469, -99.78216974382846161 ) ) ;
#5443=CARTESIAN_POINT ( 'NONE',  ( -11.02404012120765842, 76.19011824550719325, -118.0432514857309911 ) ) ;
#5455=DIRECTION ( 'NONE',  ( 0.000000000000000000, 0.000000000000000000, 1.000000000000000000 ) ) ;
#5467=CARTESIAN_POINT ( 'NONE',  ( -118.3860192952351014, 93.55239623846829033, -6.356965277239823742 ) ) ;
#5473=CYLINDRICAL_SURFACE ( 'NONE', #89048, 34.13125000000000142 ) ;
#5490=VECTOR ( 'NONE', #88016, 1000.000000000000000 ) ;
#5507=CARTESIAN_POINT ( 'NONE',  ( 130.2064250969986006, 90.93081950567962224, -9.551273559373818500 ) ) ;
#5511=VERTEX_POINT ( 'NONE', #67072 ) ;
#5513=ORIENTED_EDGE ( 'NONE', *, *, #88264, .T. ) ;
#5519=CARTESIAN_POINT ( 'NONE',  ( -12.61757850223405519, 80.88535426119446470, -129.9449579601741505 ) ) ;
#5528=CARTESIAN_POINT ( 'NONE',  ( -92.27764637677461224, 80.88465057165898031, -74.43377912862176515 ) ) ;
#5537=FACE_OUTER_BOUND ( 'NONE', #47265, .T. ) ;
#5542=SURFACE_SIDE_STYLE ('',( #82302 ) ) ;
#5583=DIRECTION ( 'NONE',  ( -0.4999999999999990563, 0.000000000000000000, -0.8660254037844392627 ) ) ;
#5593=DIRECTION ( 'NONE',  ( 0.000000000000000000, 1.000000000000000000, 0.000000000000000000 ) ) ;
#5608=EDGE_CURVE ( 'NONE', #36627, #83684, #62582, .T. ) ;
#5617=PLANE ( 'NONE',  #42165 ) ;
#5642=DIRECTION ( 'NONE',  ( 1.000000000000000000, 0.000000000000000000, 0.000000000000000000 ) ) ;
#5653=CARTESIAN_POINT ( 'NONE',  ( -1.654053778667912145, 95.16954379564980115, -118.5472977239360830 ) ) ;
#5661=CARTESIAN_POINT ( 'NONE',  ( 68.53801554307449351, 120.6499999999999915, -74.15067561874229796 ) ) ;
#5682=DIRECTION ( 'NONE',  ( 0.000000000000000000, 0.000000000000000000, 1.000000000000000000 ) ) ;
#5695=CARTESIAN_POINT ( 'NONE',  ( 88.20392011030118340, 93.55466788070657458, 79.21949419058924491 ) ) ;
#5703=CARTESIAN_POINT ( 'NONE',  ( -89.38347482486648232, 94.60320878023493663, -95.16331303980157941 ) ) ;
#5710=EDGE_LOOP ( 'NONE', ( #59053, #79670, #15981, #57002, #87201, #51776 ) ) ;
#5755=DIRECTION ( 'NONE',  ( 0.000000000000000000, 0.000000000000000000, 1.000000000000000000 ) ) ;
#5776=ADVANCED_FACE ( 'NONE', ( #77036 ), #76582, .F. ) ;
#5777=ORIENTED_EDGE ( 'NONE', *, *, #45261, .T. ) ;
#5814=ADVANCED_FACE ( 'NONE', ( #14814 ), #1635, .F. ) ;
#5844=CARTESIAN_POINT ( 'NONE',  ( 0.8399620612054651270, 69.85000000000003695, -118.5560000000000400 ) ) ;
#5856=FACE_OUTER_BOUND ( 'NONE', #52161, .T. ) ;
#5867=EDGE_LOOP ( 'NONE', ( #37005, #35358 ) ) ;
#5879=CARTESIAN_POINT ( 'NONE',  ( -130.0566101429361368, 88.18319050751495070, 11.41270026320447428 ) ) ;
#5885=VERTEX_POINT ( 'NONE', #15707 ) ;
#5887=EDGE_LOOP ( 'NONE', ( #80313, #60469, #21818, #23580 ) ) ;
#5888=DIRECTION ( 'NONE',  ( 0.000000000000000000, 0.000000000000000000, -1.000000000000000000 ) ) ;
#5910=ORIENTED_EDGE ( 'NONE', *, *, #85334, .T. ) ;
#5913=B_SPLINE_CURVE_WITH_KNOTS ( 'NONE', 3,
 ( #36275, #69485, #54920, #7700, #889, #77201, #34947, #77645, #48553, #62659, #69034, #55816, #89483, #34499, #83126, #20885, #76294, #14065, #14972, #63559, #1344, #41749, #83566, #76743, #29046, #435, #56734, #84478, #27243, #21333, #22241, #15427, #43093, #6354, #82682, #48112, #75847, #41303, #49005, #14525, #78103, #72170, #37202, #52132, #65779, #71725, #23585, #9944 ),
 .UNSPECIFIED., .F., .F.,
 ( 4, 2, 2, 2, 2, 2, 2, 2, 2, 1, 2, 2, 2, 2, 2, 2, 2, 2, 2, 2, 2, 1, 2, 2, 4 ),
 ( 0.05960646776571126848, 0.06208927922045071740, 0.06333068494782044533, 0.06457209067519016632, 0.06705490212992966381, 0.06829630785729939868, 0.06953771358466911967, 0.07202052503940853390, 0.07326193076677825489, 0.07450333649414797588, 0.07574474222151769687, 0.07698614794888740398, 0.07946895940362684596, 0.08195177085836627406, 0.08319317658573600893, 0.08443458231310574380, 0.08691739376784522741, 0.08815879949521496228, 0.08940020522258468327, 0.09188301667732418077, 0.09312442240469391563, 0.09436582813206365050, 0.09560723385943339925, 0.09684863958680312024, 0.09933145104154256222 ),
 .UNSPECIFIED. ) ;
#5920=DIRECTION ( 'NONE',  ( 0.000000000000000000, 1.000000000000000000, 0.000000000000000000 ) ) ;
#5936=LINE ( 'NONE', #80446, #21491 ) ;
#5947=VERTEX_POINT ( 'NONE', #65182 ) ;
#5961=CARTESIAN_POINT ( 'NONE',  ( 130.0566101429361936, 88.18319050751496491, -11.41270026320357189 ) ) ;
#5966=ORIENTED_EDGE ( 'NONE', *, *, #15096, .F. ) ;
#5967=AXIS2_PLACEMENT_3D ( 'NONE', #54604, #28727, #82365 ) ;
#5978=CARTESIAN_POINT ( 'NONE',  ( -77.69145367648802392, 73.00424585431358082, -89.55259891852590215 ) ) ;
#6005=DIRECTION ( 'NONE',  ( 0.000000000000000000, 0.000000000000000000, 1.000000000000000000 ) ) ;
#6009=EDGE_CURVE ( 'NONE', #78871, #26653, #17480, .T. ) ;
#6010=DIRECTION ( 'NONE',  ( 0.000000000000000000, 1.000000000000000000, 0.000000000000000000 ) ) ;
#6025=CARTESIAN_POINT ( 'NONE',  ( -98.26026929335812099, 73.28356282573676594, 85.96437953530717380 ) ) ;
#6038=FACE_OUTER_BOUND ( 'NONE', #60661, .T. ) ;
#6059=LINE ( 'NONE', #33747, #39093 ) ;
#6070=CARTESIAN_POINT ( 'NONE',  ( 3.292096649336123892, 94.82294024675948663, 118.5109520256350208 ) ) ;
#6073=DIRECTION ( 'NONE',  ( 0.8660254037844390407, 0.000000000000000000, -0.4999999999999995004 ) ) ;
#6094=DIRECTION ( 'NONE',  ( -0.000000000000000000, 1.000000000000000000, 0.000000000000000000 ) ) ;
#6122=ORIENTED_EDGE ( 'NONE', *, *, #8150, .T. ) ;
#6144=CARTESIAN_POINT ( 'NONE',  ( 92.32962665258456525, 82.54999999999999716, 74.36911441044829019 ) ) ;
#6151=CARTESIAN_POINT ( 'NONE',  ( -92.02731164704657374, 95.25015599858943460, -92.60677566276801542 ) ) ;
#6152=AXIS2_PLACEMENT_3D ( 'NONE', #57490, #49768, #42502 ) ;
#6159=VERTEX_POINT ( 'NONE', #19270 ) ;
#6171=VERTEX_POINT ( 'NONE', #34673 ) ;
#6187=CARTESIAN_POINT ( 'NONE',  ( -129.9368274816651194, 81.71102547120852932, 12.69999999999954809 ) ) ;
#6207=CARTESIAN_POINT ( 'NONE',  ( -3.968750000000770051, 120.6499999999999915, 105.4788588808462038 ) ) ;
#6212=CARTESIAN_POINT ( 'NONE',  ( -3.174999999999664979, 111.1250000000000000, -31.75000000000000000 ) ) ;
#6221=ORIENTED_EDGE ( 'NONE', *, *, #60158, .T. ) ;
#6249=VERTEX_POINT ( 'NONE', #8328 ) ;
#6266=AXIS2_PLACEMENT_3D ( 'NONE', #40173, #80645, #5682 ) ;
#6268=ORIENTED_EDGE ( 'NONE', *, *, #25378, .T. ) ;
#6286=CIRCLE ( 'NONE', #41096, 7.143749999999999822 ) ;
#6287=DIRECTION ( 'NONE',  ( 0.000000000000000000, -1.000000000000000000, 0.000000000000000000 ) ) ;
#6312=CARTESIAN_POINT ( 'NONE',  ( -130.1664033068596495, 90.28418055714726620, 10.08203418473845936 ) ) ;
#6320=ORIENTED_EDGE ( 'NONE', *, *, #66389, .F. ) ;
#6323=DIRECTION ( 'NONE',  ( 0.000000000000000000, 0.000000000000000000, -1.000000000000000000 ) ) ;
#6336=DIRECTION ( 'NONE',  ( 0.5000000000000003331, 0.000000000000000000, 0.8660254037844383745 ) ) ;
#6354=CARTESIAN_POINT ( 'NONE',  ( 89.12695577293594340, 72.47328848629024378, -78.17938156622481927 ) ) ;
#6355=ORIENTED_EDGE ( 'NONE', *, *, #42854, .F. ) ;
#6357=DIRECTION ( 'NONE',  ( 0.000000000000000000, -1.000000000000000000, 0.000000000000000000 ) ) ;
#6369=CARTESIAN_POINT ( 'NONE',  ( 92.26493792250094828, 84.21376545118702950, -74.44936585838367193 ) ) ;
#6389=CARTESIAN_POINT ( 'NONE',  ( 129.9761744276714523, 85.85000629251470627, 12.29186252049211880 ) ) ;
#6407=CARTESIAN_POINT ( 'NONE',  ( -72.96458098368600531, 117.4749999999999943, -72.96458098368781009 ) ) ;
#6411=FACE_OUTER_BOUND ( 'NONE', #27480, .T. ) ;
#6431=CARTESIAN_POINT ( 'NONE',  ( 6.802569982901797644E-16, 69.84999999999999432, 118.5560000000000116 ) ) ;
#6435=DIRECTION ( 'NONE',  ( 1.000000000000000000, 0.000000000000000000, 3.491483361109385222E-15 ) ) ;
#6450=FACE_BOUND ( 'NONE', #21334, .T. ) ;
#6452=ADVANCED_FACE ( 'NONE', ( #26864 ), #18258, .F. ) ;
#6454=CARTESIAN_POINT ( 'NONE',  ( -99.63271100832207594, 75.84295037288958952, 84.36969927706194028 ) ) ;
#6457=EDGE_LOOP ( 'NONE', ( #63258, #10362, #21308, #58387, #67657, #6886 ) ) ;
#6472=CARTESIAN_POINT ( 'NONE',  ( -86.93292302958607820, 72.22361908171431821, -97.40459591070893453 ) ) ;
#6479=DIRECTION ( 'NONE',  ( 0.000000000000000000, 1.000000000000000000, 0.000000000000000000 ) ) ;
#6485=CARTESIAN_POINT ( 'NONE',  ( -105.4788588808464027, 120.6499999999999915, 3.968749999998844924 ) ) ;
#6489=ORIENTED_EDGE ( 'NONE', *, *, #13107, .F. ) ;
#6497=CARTESIAN_POINT ( 'NONE',  ( 11.02155491792549924, 88.91427639974089914, 118.0434862571550099 ) ) ;
#6499=ORIENTED_EDGE ( 'NONE', *, *, #69170, .F. ) ;
#6532=CARTESIAN_POINT ( 'NONE',  ( 8.387180980836969724, 92.12328101316224149, -118.2604483546762282 ) ) ;
#6537=CARTESIAN_POINT ( 'NONE',  ( -72.96458098368751166, 127.0000000000000000, 72.96458098368620426 ) ) ;
#6538=ORIENTED_EDGE ( 'NONE', *, *, #28055, .F. ) ;
#6556=DIRECTION ( 'NONE',  ( -0.7071067811865495711, 0.000000000000000000, 0.7071067811865455743 ) ) ;
#6560=CARTESIAN_POINT ( 'NONE',  ( -91.50401754987770175, 76.93600387762164416, 75.38287938185037262 ) ) ;
#6564=VERTEX_POINT ( 'NONE', #39590 ) ;
#6573=DIRECTION ( 'NONE',  ( 0.000000000000000000, 1.000000000000000000, 0.000000000000000000 ) ) ;
#6580=ORIENTED_EDGE ( 'NONE', *, *, #1414, .T. ) ;
#6583=VECTOR ( 'NONE', #50177, 1000.000000000000114 ) ;
#6597=DIRECTION ( 'NONE',  ( 0.000000000000000000, 1.000000000000000000, 0.000000000000000000 ) ) ;
#6606=ORIENTED_EDGE ( 'NONE', *, *, #42189, .F. ) ;
#6623=CARTESIAN_POINT ( 'NONE',  ( 130.3463096697861943, 72.22361908171431821, 7.404590904609912982 ) ) ;
#6625=EDGE_CURVE ( 'NONE', #3921, #12790, #63631, .T. ) ;
#6633=VECTOR ( 'NONE', #15534, 1000.000000000000000 ) ;
#6634=DIRECTION ( 'NONE',  ( 0.4999999999999998890, 0.000000000000000000, -0.8660254037844387076 ) ) ;
#6686=CARTESIAN_POINT ( 'NONE',  ( -68.53801554307339927, 120.6499999999999915, -74.15067561874339219 ) ) ;
#6691=AXIS2_PLACEMENT_3D ( 'NONE', #23368, #3350, #52343 ) ;
#6695=AXIS2_PLACEMENT_3D ( 'NONE', #26465, #54583, #39192 ) ;
#6703=CARTESIAN_POINT ( 'NONE',  ( 5.041900000000000048, 117.4749999999999943, -103.1875000000000000 ) ) ;
#6710=ORIENTED_EDGE ( 'NONE', *, *, #81812, .F. ) ;
#6711=CARTESIAN_POINT ( 'NONE',  ( -117.9083433361413285, 79.66725693986899159, -12.37555662352200336 ) ) ;
#6728=DIRECTION ( 'NONE',  ( 0.000000000000000000, -0.7071067811865315855, -0.7071067811865634489 ) ) ;
#6738=DIRECTION ( 'NONE',  ( 0.000000000000000000, 1.000000000000000000, 0.000000000000000000 ) ) ;
#6749=EDGE_CURVE ( 'NONE', #12034, #72171, #35917, .T. ) ;
#6752=CYLINDRICAL_SURFACE ( 'NONE', #25901, 5.041900000000000048 ) ;
#6755=CARTESIAN_POINT ( 'NONE',  ( 72.96458098368701428, 117.4749999999999943, -72.96458098368670164 ) ) ;
#6758=CARTESIAN_POINT ( 'NONE',  ( 85.96437953530612219, 73.28356282573676594, 98.26026929335903048 ) ) ;
#6759=CARTESIAN_POINT ( 'NONE',  ( -105.4788588808464027, 127.0000000000000000, 3.968749999998844924 ) ) ;
#6765=VERTEX_POINT ( 'NONE', #22307 ) ;
#6773=CARTESIAN_POINT ( 'NONE',  ( 0.000000000000000000, 127.0000000000000000, -103.1875000000000000 ) ) ;
#6793=VECTOR ( 'NONE', #21750, 1000.000000000000000 ) ;
#6816=CARTESIAN_POINT ( 'NONE',  ( 91.11128979799246963, 89.26692529358288652, -75.85717701425140547 ) ) ;
#6817=EDGE_LOOP ( 'NONE', ( #76793, #58348, #12878, #82892 ) ) ;
#6827=VERTEX_POINT ( 'NONE', #2315 ) ;
#6831=CARTESIAN_POINT ( 'NONE',  ( 3.968750000000000000, 120.6499999999999915, -105.4788588808464027 ) ) ;
#6842=ORIENTED_EDGE ( 'NONE', *, *, #73835, .F. ) ;
#6864=VECTOR ( 'NONE', #86102, 1000.000000000000000 ) ;
#6865=DIRECTION ( 'NONE',  ( -0.2588190451025206285, 0.000000000000000000, 0.9659258262890683122 ) ) ;
#6866=ORIENTED_EDGE ( 'NONE', *, *, #29322, .F. ) ;
#6869=CARTESIAN_POINT ( 'NONE',  ( 82.89895571708365196, 82.54999999999999716, -100.8594679592203818 ) ) ;
#6871=LINE ( 'NONE', #76814, #22376 ) ;
#6884=VECTOR ( 'NONE', #81579, 1000.000000000000000 ) ;
#6886=ORIENTED_EDGE ( 'NONE', *, *, #62105, .F. ) ;
#6888=DIRECTION ( 'NONE',  ( -0.4999999999999990008, 0.000000000000000000, 0.8660254037844392627 ) ) ;
#6893=FACE_OUTER_BOUND ( 'NONE', #5867, .T. ) ;
#6908=CARTESIAN_POINT ( 'NONE',  ( -103.1875000000000000, 127.0000000000000000, -1.080832317973422076E-12 ) ) ;
#6920=EDGE_CURVE ( 'NONE', #77431, #38484, #16830, .T. ) ;
#6921=CARTESIAN_POINT ( 'NONE',  ( -83.41622542100893156, 78.46444036551650925, -100.4321520267697707 ) ) ;
#6922=CARTESIAN_POINT ( 'NONE',  ( -84.42134122279082931, 95.24969287062862122, -83.24211534968698345 ) ) ;
#6933=ORIENTED_EDGE ( 'NONE', *, *, #83123, .T. ) ;
#6949=CARTESIAN_POINT ( 'NONE',  ( 4.868064396069526900, 94.30179516618007085, 118.4578665249601102 ) ) ;
#6976=CARTESIAN_POINT ( 'NONE',  ( 72.96458098368650269, 127.0000000000000000, 67.92268098368730023 ) ) ;
#6981=CARTESIAN_POINT ( 'NONE',  ( 0.8301440424157503495, 95.22976080284070122, -118.5538265829301565 ) ) ;
#6987=ORIENTED_EDGE ( 'NONE', *, *, #54071, .T. ) ;
#6995=CARTESIAN_POINT ( 'NONE',  ( 0.000000000000000000, 117.4749999999999943, -103.1875000000000000 ) ) ;
#7014=EDGE_LOOP ( 'NONE', ( #70795, #75809 ) ) ;
#7026=AXIS2_PLACEMENT_3D ( 'NONE', #40544, #5593, #33288 ) ;
#7047=ORIENTED_EDGE ( 'NONE', *, *, #70922, .F. ) ;
#7076=CARTESIAN_POINT ( 'NONE',  ( 130.4023353925299489, 71.53177522571071734, 6.370020420676822503 ) ) ;
#7088=CARTESIAN_POINT ( 'NONE',  ( 3.968749999999229949, 120.6499999999999915, 100.8961411191535973 ) ) ;
#7096=DIRECTION ( 'NONE',  ( 0.000000000000000000, 0.000000000000000000, -1.000000000000000000 ) ) ;
#7102=EDGE_CURVE ( 'NONE', #76987, #81147, #71142, .T. ) ;
#7105=CYLINDRICAL_SURFACE ( 'NONE', #65491, 5.041900000000001825 ) ;
#7116=EDGE_LOOP ( 'NONE', ( #68504, #70383 ) ) ;
#7133=EDGE_LOOP ( 'NONE', ( #59269, #52202, #83808, #54745 ) ) ;
#7137=CARTESIAN_POINT ( 'NONE',  ( 94.33669211993637305, 94.92443974548203300, 90.25311968877711877 ) ) ;
#7141=DIRECTION ( 'NONE',  ( 0.000000000000000000, 1.000000000000000000, 0.000000000000000000 ) ) ;
#7152=CIRCLE ( 'NONE', #76784, 7.143750000000001599 ) ;
#7166=DIRECTION ( 'NONE',  ( 0.000000000000000000, -1.000000000000000000, 0.000000000000000000 ) ) ;
#7172=VERTEX_POINT ( 'NONE', #59700 ) ;
#7173=CARTESIAN_POINT ( 'NONE',  ( -118.3034456680046702, 72.47328848629024378, -7.741103959107750399 ) ) ;
#7174=VERTEX_POINT ( 'NONE', #18378 ) ;
#7186=DIRECTION ( 'NONE',  ( 0.000000000000000000, 1.000000000000000000, 0.000000000000000000 ) ) ;
#7194=CARTESIAN_POINT ( 'NONE',  ( 72.96458098368650269, 127.0000000000000000, 72.96458098368729850 ) ) ;
#7205=AXIS2_PLACEMENT_3D ( 'NONE', #34611, #55477, #20554 ) ;
#7206=LINE ( 'NONE', #76237, #21831 ) ;
#7215=CARTESIAN_POINT ( 'NONE',  ( 98.06260288352331145, 72.98383416765820186, 86.19129576945198323 ) ) ;
#7228=CARTESIAN_POINT ( 'NONE',  ( 72.96458098368650269, 117.4749999999999943, 72.96458098368729850 ) ) ;
#7230=MECHANICAL_DESIGN_GEOMETRIC_PRESENTATION_REPRESENTATION('',(#50720),#63772);
#7251=EDGE_CURVE ( 'NONE', #79223, #55335, #11116, .T. ) ;
#7254=LINE ( 'NONE', #76737, #64077 ) ;
#7257=CARTESIAN_POINT ( 'NONE',  ( -117.9438598201574990, 86.63388195152280957, 12.03269986015488868 ) ) ;
#7277=CARTESIAN_POINT ( 'NONE',  ( 77.01901799881285626, 91.23868085022587593, -90.13147184857885463 ) ) ;
#7281=ORIENTED_EDGE ( 'NONE', *, *, #49359, .T. ) ;
#7293=CARTESIAN_POINT ( 'NONE',  ( 3.174999999999879918, 124.5870000000000033, 33.98325472291465132 ) ) ;
#7297=ORIENTED_EDGE ( 'NONE', *, *, #46817, .F. ) ;
#7307=DIRECTION ( 'NONE',  ( 0.000000000000000000, 1.000000000000000000, 0.000000000000000000 ) ) ;
#7315=CARTESIAN_POINT ( 'NONE',  ( -74.36911441044667015, 81.72118090664557144, -92.32962665258587265 ) ) ;
#7320=DIRECTION ( 'NONE',  ( -1.046082768126375896E-16, 0.000000000000000000, -1.000000000000000000 ) ) ;
#7334=LINE ( 'NONE', #69112, #28369 ) ;
#7337=EDGE_LOOP ( 'NONE', ( #10568, #6933 ) ) ;
#7346=ORIENTED_EDGE ( 'NONE', *, *, #52721, .T. ) ;
#7352=LINE ( 'NONE', #62302, #21037 ) ;
#7354=CARTESIAN_POINT ( 'NONE',  ( -88.25674559704555122, 71.15434825076368952, 96.20681132576139305 ) ) ;
#7356=EDGE_LOOP ( 'NONE', ( #11026, #89700, #66603, #77445, #33510, #74262 ) ) ;
#7365=CARTESIAN_POINT ( 'NONE',  ( 68.53801554307449351, 127.0000000000000000, -74.15067561874229796 ) ) ;
#7367=CARTESIAN_POINT ( 'NONE',  ( 1.166476076187854022E-15, 95.25000000000000000, -9.525000000000000355 ) ) ;
#7379=B_SPLINE_CURVE_WITH_KNOTS ( 'NONE', 3,
 ( #52273, #67731, #5519, #60913, #88641, #26397, #54070, #19578, #48602, #34091, #69081, #40471, #89078, #40911, #28174, #68188, #56318, #49508, #20039, #28633, #48161, #61795, #26836, #14116, #84065 ),
 .UNSPECIFIED., .F., .F.,
 ( 4, 2, 2, 2, 2, 2, 2, 2, 2, 1, 2, 2, 4 ),
 ( 0.05959919981814688211, 0.06208050401323544909, 0.06332115611077974993, 0.06456180820832406464, 0.06704311240341262468, 0.06828376450095689776, 0.06952441659850118472, 0.07200572079358977251, 0.07324637289113407335, 0.07448702498867838806, 0.07572767708622268890, 0.07696832918376700361, 0.07944963337885561916 ),
 .UNSPECIFIED. ) ;
#7386=FACE_BOUND ( 'NONE', #7494, .T. ) ;
#7411=DIRECTION ( 'NONE',  ( 0.000000000000000000, 1.000000000000000000, 0.000000000000000000 ) ) ;
#7419=CARTESIAN_POINT ( 'NONE',  ( -72.96458098368600531, 127.0000000000000000, -65.82083098368781293 ) ) ;
#7426=CARTESIAN_POINT ( 'NONE',  ( 6.715083999775234069, 93.33742752469728998, -118.3661748111209420 ) ) ;
#7429=CARTESIAN_POINT ( 'NONE',  ( -10.09777173618929602, 90.29655250510948861, 130.1657284840295006 ) ) ;
#7442=DIRECTION ( 'NONE',  ( -0.4999999999999998890, 0.000000000000000000, 0.8660254037844387076 ) ) ;
#7450=EDGE_LOOP ( 'NONE', ( #3584, #60194, #67290, #34318, #22309, #33034 ) ) ;
#7460=AXIS2_PLACEMENT_3D ( 'NONE', #80213, #88814, #19761 ) ;
#7479=EDGE_CURVE ( 'NONE', #75690, #32614, #68333, .T. ) ;
#7487=CARTESIAN_POINT ( 'NONE',  ( -100.8961411191535973, 120.6499999999999915, 3.968749999998880451 ) ) ;
#7490=DIRECTION ( 'NONE',  ( 0.000000000000000000, -1.000000000000000000, 0.000000000000000000 ) ) ;
#7494=EDGE_LOOP ( 'NONE', ( #6606, #75462 ) ) ;
#7496=ORIENTED_EDGE ( 'NONE', *, *, #29183, .T. ) ;
#7516=CARTESIAN_POINT ( 'NONE',  ( 8.748570571408901218E-16, 117.4749999999999943, -96.04375000000000284 ) ) ;
#7520=CARTESIAN_POINT ( 'NONE',  ( -98.60478223830740774, 127.0000000000000000, -1.074461880482445986E-12 ) ) ;
#7524=VECTOR ( 'NONE', #52776, 1000.000000000000000 ) ;
#7525=ORIENTED_EDGE ( 'NONE', *, *, #77993, .F. ) ;
#7529=AXIS2_PLACEMENT_3D ( 'NONE', #73060, #10835, #87158 ) ;
#7540=CARTESIAN_POINT ( 'NONE',  ( 0.000000000000000000, 92.07499999999998863, 0.000000000000000000 ) ) ;
#7541=CARTESIAN_POINT ( 'NONE',  ( -77.39114642430010349, 120.6499999999999915, 71.77848634863050847 ) ) ;
#7547=CARTESIAN_POINT ( 'NONE',  ( -7.199374239792870816E-13, 117.4749999999999943, 98.14560000000000173 ) ) ;
#7560=DIRECTION ( 'NONE',  ( 0.000000000000000000, 1.000000000000000000, 0.000000000000000000 ) ) ;
#7570=ORIENTED_EDGE ( 'NONE', *, *, #13107, .T. ) ;
#7576=AXIS2_PLACEMENT_3D ( 'NONE', #86311, #24088, #66746 ) ;
#7587=CARTESIAN_POINT ( 'NONE',  ( 100.8594679592200691, 83.38918798244691288, 82.89895571708403565 ) ) ;
#7596=DIRECTION ( 'NONE',  ( 0.000000000000000000, -1.000000000000000000, 0.000000000000000000 ) ) ;
#7601=DIRECTION ( 'NONE',  ( 0.000000000000000000, 1.000000000000000000, 0.000000000000000000 ) ) ;
#7623=CARTESIAN_POINT ( 'NONE',  ( 11.00664350276215941, 76.20047485311516766, -118.0441341279204721 ) ) ;
#7624=DIRECTION ( 'NONE',  ( 0.7071067811865460184, 0.000000000000000000, -0.7071067811865489050 ) ) ;
#7665=ORIENTED_EDGE ( 'NONE', *, *, #37483, .T. ) ;
#7675=CARTESIAN_POINT ( 'NONE',  ( -12.70000000000000107, 82.54999999999999716, 129.9368274816650910 ) ) ;
#7700=CARTESIAN_POINT ( 'NONE',  ( 74.62312585591649849, 79.66685870724424490, -92.12448541806578817 ) ) ;
#7704=ORIENTED_EDGE ( 'NONE', *, *, #53723, .T. ) ;
#7728=EDGE_LOOP ( 'NONE', ( #45921, #35994 ) ) ;
#7730=CARTESIAN_POINT ( 'NONE',  ( -31.75000000000000000, 111.1250000000000000, 3.174999999999779998 ) ) ;
#7755=VERTEX_POINT ( 'NONE', #12360 ) ;
#7760=CYLINDRICAL_SURFACE ( 'NONE', #66410, 34.13125000000000142 ) ;
#7765=DIRECTION ( 'NONE',  ( 0.000000000000000000, 0.000000000000000000, 1.000000000000000000 ) ) ;
#7784=VECTOR ( 'NONE', #72011, 1000.000000000000000 ) ;
#7818=CARTESIAN_POINT ( 'NONE',  ( -75.69222284415457125, 88.91144712388911842, -91.24829632406229507 ) ) ;
#7825=CARTESIAN_POINT ( 'NONE',  ( 72.96458098368701428, 127.0000000000000000, -72.96458098368670164 ) ) ;
#7827=ORIENTED_EDGE ( 'NONE', *, *, #14724, .F. ) ;
#7830=FACE_OUTER_BOUND ( 'NONE', #40384, .T. ) ;
#7863=AXIS2_PLACEMENT_3D ( 'NONE', #22880, #56008, #35582 ) ;
#7881=CARTESIAN_POINT ( 'NONE',  ( -3.968749999999935163, 120.6499999999999915, -100.8961411191535973 ) ) ;
#7892=CARTESIAN_POINT ( 'NONE',  ( -3.968750000000770051, 120.6499999999999915, 105.4788588808462038 ) ) ;
#7901=CARTESIAN_POINT ( 'NONE',  ( 105.4788588808464027, 120.6499999999999915, 3.968750000000405009 ) ) ;
#7902=CARTESIAN_POINT ( 'NONE',  ( -92.12462914090755817, 79.66725693986894896, 74.62294912200682973 ) ) ;
#7924=ORIENTED_EDGE ( 'NONE', *, *, #29692, .T. ) ;
#7931=AXIS2_PLACEMENT_3D ( 'NONE', #12359, #54551, #60947 ) ;
#7936=EDGE_LOOP ( 'NONE', ( #35636, #71289 ) ) ;
#7941=DIRECTION ( 'NONE',  ( 0.2588190451025189631, 0.000000000000000000, 0.9659258262890688673 ) ) ;
#7993=ORIENTED_EDGE ( 'NONE', *, *, #82925, .F. ) ;
#8030=CARTESIAN_POINT ( 'NONE',  ( 88.53717826876548713, 94.12569442554141119, 95.94886839522675359 ) ) ;
#8037=CARTESIAN_POINT ( 'NONE',  ( 103.1875000000000000, 127.0000000000000000, 7.937500000000360600 ) ) ;
#8046=ORIENTED_EDGE ( 'NONE', *, *, #70831, .T. ) ;
#8052=ADVANCED_FACE ( 'NONE', ( #1872, #55900 ), #48642, .T. ) ;
#8055=CARTESIAN_POINT ( 'NONE',  ( -12.70000000000000462, 82.96441223327236969, 117.8738102209307641 ) ) ;
#8071=CARTESIAN_POINT ( 'NONE',  ( 12.70000000000000284, 81.72078997525719046, -117.8738102209307641 ) ) ;
#8076=VERTEX_POINT ( 'NONE', #20530 ) ;
#8079=ORIENTED_EDGE ( 'NONE', *, *, #32049, .T. ) ;
#8087=AXIS2_PLACEMENT_3D ( 'NONE', #88225, #12353, #40044 ) ;
#8088=DIRECTION ( 'NONE',  ( 0.000000000000000000, 0.000000000000000000, 1.000000000000000000 ) ) ;
#8093=CARTESIAN_POINT ( 'NONE',  ( -72.96458098368751166, 127.0000000000000000, 80.90208098368620426 ) ) ;
#8097=EDGE_CURVE ( 'NONE', #78413, #69399, #75927, .T. ) ;
#8110=CARTESIAN_POINT ( 'NONE',  ( 94.33976020835903853, 70.17656663518266669, 90.24991642302124717 ) ) ;
#8121=FACE_OUTER_BOUND ( 'NONE', #86008, .T. ) ;
#8129=AXIS2_PLACEMENT_3D ( 'NONE', #24557, #79537, #58177 ) ;
#8142=VERTEX_POINT ( 'NONE', #31347 ) ;
#8145=CARTESIAN_POINT ( 'NONE',  ( -75.00112839233693762, 87.03046781249436492, 91.81710919847719765 ) ) ;
#8150=EDGE_CURVE ( 'NONE', #86064, #29444, #34973, .T. ) ;
#8167=CARTESIAN_POINT ( 'NONE',  ( -7.205548786489490269E-13, 127.0000000000000000, 103.1875000000000000 ) ) ;
#8170=CARTESIAN_POINT ( 'NONE',  ( 79.21949419058893227, 93.55466788070661721, -88.20392011030149604 ) ) ;
#8187=EDGE_CURVE ( 'NONE', #53265, #24560, #86328, .T. ) ;
#8237=CARTESIAN_POINT ( 'NONE',  ( 72.96458098368650269, 127.0000000000000000, 72.96458098368729850 ) ) ;
#8248=FACE_OUTER_BOUND ( 'NONE', #41714, .T. ) ;
#8255=AXIS2_PLACEMENT_3D ( 'NONE', #1065, #70560, #1525 ) ;
#8266=EDGE_CURVE ( 'NONE', #52316, #46913, #38608, .T. ) ;
#8271=ORIENTED_EDGE ( 'NONE', *, *, #37995, .T. ) ;
#8274=CARTESIAN_POINT ( 'NONE',  ( -80.89343850130802593, 94.60304557064716846, -86.67392531623340801 ) ) ;
#8309=VERTEX_POINT ( 'NONE', #32688 ) ;
#8312=AXIS2_PLACEMENT_3D ( 'NONE', #79989, #17741, #5455 ) ;
#8328=CARTESIAN_POINT ( 'NONE',  ( -117.8738102209307215, 82.54999999999999716, -12.70000000000041318 ) ) ;
#8331=CARTESIAN_POINT ( 'NONE',  ( -11.39408073823492806, 88.17482193101731980, 130.0579986637597187 ) ) ;
#8344=CARTESIAN_POINT ( 'NONE',  ( 100.8961411191535973, 120.6499999999999915, -3.968749999999580336 ) ) ;
#8365=ORIENTED_EDGE ( 'NONE', *, *, #83144, .T. ) ;
#8385=CARTESIAN_POINT ( 'NONE',  ( 12.61757850223405519, 80.88535426119446470, 129.9449579601741505 ) ) ;
#8386=CARTESIAN_POINT ( 'NONE',  ( -100.8594679592206802, 82.54999999999999716, -82.89895571708333932 ) ) ;
#8393=LINE ( 'NONE', #62887, #46515 ) ;
#8401=VERTEX_POINT ( 'NONE', #11810 ) ;
#8403=CARTESIAN_POINT ( 'NONE',  ( 4.163101094985349692E-14, 120.6499999999999915, -98.60478223830740774 ) ) ;
#8407=FACE_OUTER_BOUND ( 'NONE', #12138, .T. ) ;
#8427=CARTESIAN_POINT ( 'NONE',  ( -130.5477899301573927, 69.93364840292896645, -1.674143004589110140 ) ) ;
#8464=AXIS2_PLACEMENT_3D ( 'NONE', #28531, #82642, #49418 ) ;
#8465=EDGE_CURVE ( 'NONE', #8076, #83603, #69457, .T. ) ;
#8477=CIRCLE ( 'NONE', #38859, 190.5000000000000000 ) ;
#8488=CARTESIAN_POINT ( 'NONE',  ( 87.44900557253099294, 93.33921197991990937, 96.94152442043777285 ) ) ;
#8504=EDGE_LOOP ( 'NONE', ( #15770, #26334, #71639, #3615 ) ) ;
#8515=VECTOR ( 'NONE', #15056, 999.9999999999998863 ) ;
#8561=CARTESIAN_POINT ( 'NONE',  ( 97.63922045723853671, 72.45841406287408404, 86.67141577317495660 ) ) ;
#8585=CIRCLE ( 'NONE', #82644, 5.041900000000001825 ) ;
#8599=DIRECTION ( 'NONE',  ( 0.000000000000000000, 1.000000000000000000, 0.000000000000000000 ) ) ;
#8604=CARTESIAN_POINT ( 'NONE',  ( -91.61507027739536113, 87.79588542099537563, 75.24778849303649508 ) ) ;
#8608=CIRCLE ( 'NONE', #57875, 7.937500000000000000 ) ;
#8620=DIRECTION ( 'NONE',  ( 0.000000000000000000, 1.000000000000000000, 0.000000000000000000 ) ) ;
#8629=CARTESIAN_POINT ( 'NONE',  ( 85.28591416242399248, 95.08639429146514033, -82.35292268805471849 ) ) ;
#8635=ORIENTED_EDGE ( 'NONE', *, *, #50292, .F. ) ;
#8673=VECTOR ( 'NONE', #62687, 1000.000000000000000 ) ;
#8678=CIRCLE ( 'NONE', #4322, 5.041900000000000048 ) ;
#8685=AXIS2_PLACEMENT_3D ( 'NONE', #9429, #37140, #8088 ) ;
#8716=ADVANCED_FACE ( 'NONE', ( #36280 ), #1765, .F. ) ;
#8731=EDGE_CURVE ( 'NONE', #11327, #70447, #71262, .T. ) ;
#8733=CARTESIAN_POINT ( 'NONE',  ( -88.44471653959766400, 93.33860577356858812, -78.95047879920376488 ) ) ;
#8736=CARTESIAN_POINT ( 'NONE',  ( 103.1875000000000000, 117.4749999999999943, 3.602774393244745134E-13 ) ) ;
#8766=CARTESIAN_POINT ( 'NONE',  ( -7.399926448127667200, 72.22026871922481916, 130.3465752436562468 ) ) ;
#8773=EDGE_CURVE ( 'NONE', #4701, #24255, #13884, .T. ) ;
#8776=CARTESIAN_POINT ( 'NONE',  ( -103.1875000000000000, 127.0000000000000000, -1.080832317973422076E-12 ) ) ;
#8778=UNCERTAINTY_MEASURE_WITH_UNIT (LENGTH_MEASURE( 1.000000000000000082E-05 ), #5078, 'distance_accuracy_value', 'NONE');
#8787=EDGE_CURVE ( 'NONE', #64021, #49178, #15291, .T. ) ;
#8810=EDGE_CURVE ( 'NONE', #32576, #20813, #1158, .T. ) ;
#8814=VECTOR ( 'NONE', #9792, 1000.000000000000000 ) ;
#8815=CARTESIAN_POINT ( 'NONE',  ( 72.96458098368701428, 127.0000000000000000, -72.96458098368670164 ) ) ;
#8817=DIRECTION ( 'NONE',  ( 0.000000000000000000, -1.000000000000000000, 0.000000000000000000 ) ) ;
#8835=LINE ( 'NONE', #51038, #44903 ) ;
#8849=AXIS2_PLACEMENT_3D ( 'NONE', #6755, #48503, #55328 ) ;
#8856=AXIS2_PLACEMENT_3D ( 'NONE', #58442, #24828, #80256 ) ;
#8862=VECTOR ( 'NONE', #20825, 1000.000000000000000 ) ;
#8871=EDGE_CURVE ( 'NONE', #12810, #31262, #83835, .T. ) ;
#8885=CARTESIAN_POINT ( 'NONE',  ( -130.5560612649026666, 69.84937019662270075, 0.8297548318613829910 ) ) ;
#8904=CARTESIAN_POINT ( 'NONE',  ( 3.175000000000334666, 111.1250000000000000, -31.75000000000000000 ) ) ;
#8910=VERTEX_POINT ( 'NONE', #85635 ) ;
#8912=CARTESIAN_POINT ( 'NONE',  ( -103.1875000000000000, 127.0000000000000000, -7.143750000001079847 ) ) ;
#8921=LINE ( 'NONE', #83416, #33493 ) ;
#8957=DIRECTION ( 'NONE',  ( 0.000000000000000000, 1.000000000000000000, 0.000000000000000000 ) ) ;
#8971=ADVANCED_FACE ( 'NONE', ( #71989 ), #52385, .F. ) ;
#8986=FACE_BOUND ( 'NONE', #61, .T. ) ;
#8988=EDGE_LOOP ( 'NONE', ( #78923, #43522, #2486, #39731 ) ) ;
#8992=PLANE ( 'NONE',  #76544 ) ;
#9005=CARTESIAN_POINT ( 'NONE',  ( 8.748570571408911079E-16, 127.0000000000000000, -96.04375000000000284 ) ) ;
#9023=ORIENTED_EDGE ( 'NONE', *, *, #46375, .T. ) ;
#9024=ADVANCED_FACE ( 'NONE', ( #20648 ), #40171, .T. ) ;
#9031=CIRCLE ( 'NONE', #46727, 190.5000000000000000 ) ;
#9033=CARTESIAN_POINT ( 'NONE',  ( 86.13269706310835261, 70.27900073646853230, 81.46681417397539349 ) ) ;
#9052=FACE_OUTER_BOUND ( 'NONE', #86603, .T. ) ;
#9079=ORIENTED_EDGE ( 'NONE', *, *, #38806, .F. ) ;
#9080=ORIENTED_EDGE ( 'NONE', *, *, #79136, .T. ) ;
#9091=EDGE_LOOP ( 'NONE', ( #36094, #41540 ) ) ;
#9097=AXIS2_PLACEMENT_3D ( 'NONE', #41460, #14683, #70081 ) ;
#9102=CARTESIAN_POINT ( 'NONE',  ( -103.1875000000000000, 101.5999999999999943, 5.041899999998910253 ) ) ;
#9106=DIRECTION ( 'NONE',  ( 0.000000000000000000, 1.000000000000000000, 0.000000000000000000 ) ) ;
#9157=CARTESIAN_POINT ( 'NONE',  ( -94.61941200740652391, 94.84315624882771090, 89.95943163722139957 ) ) ;
#9158=AXIS2_PLACEMENT_3D ( 'NONE', #2387, #1036, #63260 ) ;
#9162=FACE_OUTER_BOUND ( 'NONE', #49253, .T. ) ;
#9173=DIRECTION ( 'NONE',  ( 0.000000000000000000, 1.000000000000000000, 0.000000000000000000 ) ) ;
#9183=EDGE_LOOP ( 'NONE', ( #68958, #35707, #79608, #71525 ) ) ;
#9193=VERTEX_POINT ( 'NONE', #41955 ) ;
#9197=VERTEX_POINT ( 'NONE', #7901 ) ;
#9240=VECTOR ( 'NONE', #71291, 1000.000000000000000 ) ;
#9275=DIRECTION ( 'NONE',  ( 0.5000000000000061062, 0.000000000000000000, -0.8660254037844351549 ) ) ;
#9290=LINE ( 'NONE', #28375, #11431 ) ;
#9291=ORIENTED_EDGE ( 'NONE', *, *, #74697, .T. ) ;
#9302=ORIENTED_EDGE ( 'NONE', *, *, #66389, .T. ) ;
#9317=CARTESIAN_POINT ( 'NONE',  ( -130.0004344034682617, 78.46444036551649504, -12.03207709110584211 ) ) ;
#9318=VERTEX_POINT ( 'NONE', #17841 ) ;
#9320=VERTEX_POINT ( 'NONE', #44192 ) ;
#9356=CARTESIAN_POINT ( 'NONE',  ( -7.752238106858478695, 92.64409645872694909, -130.3274943305225406 ) ) ;
#9359=FACE_OUTER_BOUND ( 'NONE', #17449, .T. ) ;
#9377=VECTOR ( 'NONE', #39588, 1000.000000000000000 ) ;
#9378=CARTESIAN_POINT ( 'NONE',  ( 77.39114642429899504, 120.6499999999999915, 71.77848634863160271 ) ) ;
#9380=CARTESIAN_POINT ( 'NONE',  ( 76.38857008572915674, 90.29828471680515634, 90.66710916952514765 ) ) ;
#9387=CARTESIAN_POINT ( 'NONE',  ( -72.96458098368751166, 117.4749999999999943, 72.96458098368620426 ) ) ;
#9423=CIRCLE ( 'NONE', #63098, 5.041900000000000048 ) ;
#9429=CARTESIAN_POINT ( 'NONE',  ( 0.000000000000000000, 92.07499999999998863, 0.000000000000000000 ) ) ;
#9434=DIRECTION ( 'NONE',  ( -0.000000000000000000, 1.000000000000000000, 0.000000000000000000 ) ) ;
#9436=VERTEX_POINT ( 'NONE', #40063 ) ;
#9440=DIRECTION ( 'NONE',  ( 0.000000000000000000, -1.000000000000000000, 0.000000000000000000 ) ) ;
#9484=AXIS2_PLACEMENT_3D ( 'NONE', #21438, #34602, #48660 ) ;
#9496=B_SPLINE_CURVE_WITH_KNOTS ( 'NONE', 3,
 ( #4621, #67281, #5528, #33221, #60460, #54080, #19585, #47277, #11433, #75003, #65934, #59115, #10975, #38677, #31868, #32306, #4172, #34555, #62714, #76347, #47726, #13671, #62262, #20046, #48609, #41803, #69539, #89087, #35447, #56329, #63163, #75463, #54972, #82739, #5978, #14583, #945, #68643, #54526, #14125, #20503, #492, #42258, #21391, #83623, #13232, #7315, #28182 ),
 .UNSPECIFIED., .F., .F.,
 ( 4, 2, 2, 2, 2, 2, 2, 2, 2, 1, 2, 2, 2, 2, 2, 2, 2, 2, 2, 2, 2, 1, 2, 2, 4 ),
 ( 0.05960646776571127542, 0.06208927922045080761, 0.06333068494782057023, 0.06457209067519034673, 0.06705490212992989973, 0.06829630785729966236, 0.06953771358466942498, 0.07202052503940886696, 0.07326193076677858795, 0.07450333649414830894, 0.07574474222151801606, 0.07698614794888773705, 0.07946895940362716515, 0.08195177085836659325, 0.08319317658573632812, 0.08443458231310606299, 0.08691739376784554660, 0.08815879949521529535, 0.08940020522258504410, 0.09188301667732448608, 0.09312442240469417931, 0.09436582813206385867, 0.09560723385943355190, 0.09684863958680324514, 0.09933145104154257610 ),
 .UNSPECIFIED. ) ;
#9512=ORIENTED_EDGE ( 'NONE', *, *, #5608, .F. ) ;
#9540=VECTOR ( 'NONE', #35415, 1000.000000000000000 ) ;
#9559=EDGE_CURVE ( 'NONE', #28103, #62184, #7352, .T. ) ;
#9571=CARTESIAN_POINT ( 'NONE',  ( 100.8961411191535973, 127.0000000000000000, -3.968749999999580336 ) ) ;
#9597=CARTESIAN_POINT ( 'NONE',  ( -89.37916159652597514, 94.58014758961630264, 95.16508291382922380 ) ) ;
#9601=DIRECTION ( 'NONE',  ( 0.000000000000000000, 1.000000000000000000, 0.000000000000000000 ) ) ;
#9615=AXIS2_PLACEMENT_3D ( 'NONE', #41148, #62942, #42047 ) ;
#9633=VERTEX_POINT ( 'NONE', #21434 ) ;
#9680=EDGE_CURVE ( 'NONE', #37237, #3921, #64113, .T. ) ;
#9694=EDGE_CURVE ( 'NONE', #19831, #72752, #38404, .T. ) ;
#9701=ADVANCED_FACE ( 'NONE', ( #8248 ), #35487, .T. ) ;
#9703=EDGE_CURVE ( 'NONE', #67094, #28641, #42295, .T. ) ;
#9714=DIRECTION ( 'NONE',  ( 0.000000000000000000, -1.000000000000000000, 0.000000000000000000 ) ) ;
#9719=VERTEX_POINT ( 'NONE', #73135 ) ;
#9749=CIRCLE ( 'NONE', #21355, 7.143750000000001599 ) ;
#9764=CIRCLE ( 'NONE', #44557, 42.54500000000000171 ) ;
#9792=DIRECTION ( 'NONE',  ( -0.4999999999999998890, 0.000000000000000000, 0.8660254037844387076 ) ) ;
#9803=CARTESIAN_POINT ( 'NONE',  ( -6.710386649963790084, 93.34051461951032991, -130.3838978039176482 ) ) ;
#9817=AXIS2_PLACEMENT_3D ( 'NONE', #42171, #43512, #77612 ) ;
#9818=VECTOR ( 'NONE', #47734, 1000.000000000000000 ) ;
#9821=DIRECTION ( 'NONE',  ( 0.000000000000000000, 1.000000000000000000, 0.000000000000000000 ) ) ;
#9833=CARTESIAN_POINT ( 'NONE',  ( 2.883471595053340053, 94.92538689125287021, 130.5247975405367811 ) ) ;
#9843=VERTEX_POINT ( 'NONE', #67675 ) ;
#9873=EDGE_CURVE ( 'NONE', #12790, #87834, #54010, .T. ) ;
#9895=ORIENTED_EDGE ( 'NONE', *, *, #22033, .F. ) ;
#9899=CARTESIAN_POINT ( 'NONE',  ( 0.000000000000000000, 61.59999999999999432, 130.5560000000000116 ) ) ;
#9913=DIRECTION ( 'NONE',  ( 0.000000000000000000, 0.000000000000000000, 1.000000000000000000 ) ) ;
#9919=CARTESIAN_POINT ( 'NONE',  ( 91.90737012895596081, 78.46643079253878739, 74.89042153202969132 ) ) ;
#9929=DIRECTION ( 'NONE',  ( 0.7071067811865398012, 0.000000000000000000, 0.7071067811865552333 ) ) ;
#9931=ADVANCED_FACE ( 'NONE', ( #18629 ), #26775, .F. ) ;
#9944=CARTESIAN_POINT ( 'NONE',  ( 92.32962665258612844, 82.54999999999999716, -74.36911441044637172 ) ) ;
#9964=CARTESIAN_POINT ( 'NONE',  ( -31.75000000000000000, 111.1250000000000000, 3.174999999999779998 ) ) ;
#9967=DIRECTION ( 'NONE',  ( 0.7071067811865460184, 0.000000000000000000, -0.7071067811865489050 ) ) ;
#9974=DIRECTION ( 'NONE',  ( 0.000000000000000000, 1.000000000000000000, 0.000000000000000000 ) ) ;
#9991=FACE_OUTER_BOUND ( 'NONE', #10922, .T. ) ;
#10047=CARTESIAN_POINT ( 'NONE',  ( 4.163101094985349692E-14, 120.6499999999999915, -98.60478223830740774 ) ) ;
#10052=ORIENTED_EDGE ( 'NONE', *, *, #47098, .F. ) ;
#10067=CARTESIAN_POINT ( 'NONE',  ( 103.1875000000000000, 127.0000000000000000, 7.143750000000359535 ) ) ;
#10084=CIRCLE ( 'NONE', #1335, 38.10000000000000142 ) ;
#10097=CARTESIAN_POINT ( 'NONE',  ( -4.084841600441663445, 70.51762400537137410, 130.4926920574403937 ) ) ;
#10105=AXIS2_PLACEMENT_3D ( 'NONE', #87358, #12851, #67336 ) ;
#10127=CIRCLE ( 'NONE', #31832, 5.041900000000001825 ) ;
#10133=ADVANCED_FACE ( 'NONE', ( #42530 ), #765, .T. ) ;
#10141=ORIENTED_EDGE ( 'NONE', *, *, #25552, .F. ) ;
#10157=CARTESIAN_POINT ( 'NONE',  ( 118.1931971052176777, 73.86197090048099767, -9.272510012970347049 ) ) ;
#10168=VECTOR ( 'NONE', #2798, 1000.000000000000000 ) ;
#10171=EDGE_CURVE ( 'NONE', #78871, #2616, #23025, .T. ) ;
#10188=VECTOR ( 'NONE', #47495, 999.9999999999998863 ) ;
#10190=ADVANCED_FACE ( 'NONE', ( #57960 ), #15308, .T. ) ;
#10199=DIRECTION ( 'NONE',  ( 0.000000000000000000, 1.000000000000000000, 0.000000000000000000 ) ) ;
#10202=CARTESIAN_POINT ( 'NONE',  ( -130.3836616406706526, 71.76234181793739708, 6.714949744938381038 ) ) ;
#10225=CARTESIAN_POINT ( 'NONE',  ( 72.96458098368701428, 101.5999999999999943, -72.96458098368670164 ) ) ;
#10227=EDGE_LOOP ( 'NONE', ( #53256, #34294 ) ) ;
#10243=EDGE_CURVE ( 'NONE', #2816, #67094, #73826, .T. ) ;
#10253=EDGE_CURVE ( 'NONE', #64446, #83766, #52015, .T. ) ;
#10263=LINE ( 'NONE', #37963, #52280 ) ;
#10286=CIRCLE ( 'NONE', #78531, 7.143750000000004263 ) ;
#10291=VECTOR ( 'NONE', #47250, 1000.000000000000000 ) ;
#10357=CARTESIAN_POINT ( 'NONE',  ( 74.43211355457049194, 80.89685143461890959, 92.27899210470947367 ) ) ;
#10362=ORIENTED_EDGE ( 'NONE', *, *, #51847, .F. ) ;
#10367=CARTESIAN_POINT ( 'NONE',  ( -72.96458098368600531, 127.0000000000000000, -72.96458098368781009 ) ) ;
#10385=DIRECTION ( 'NONE',  ( 0.000000000000000000, 1.000000000000000000, 0.000000000000000000 ) ) ;
#10394=CYLINDRICAL_SURFACE ( 'NONE', #37512, 7.143750000000004263 ) ;
#10456=CARTESIAN_POINT ( 'NONE',  ( -2.077912807000512618, 95.08573034283286063, 130.5400978111108259 ) ) ;
#10464=DIRECTION ( 'NONE',  ( 0.000000000000000000, 1.000000000000000000, 0.000000000000000000 ) ) ;
#10468=EDGE_CURVE ( 'NONE', #29480, #89346, #9764, .T. ) ;
#10488=CARTESIAN_POINT ( 'NONE',  ( -100.8594679592212344, 82.54999999999999716, 82.89895571708261457 ) ) ;
#10489=CARTESIAN_POINT ( 'NONE',  ( 72.96458098368701428, 127.0000000000000000, -72.96458098368670164 ) ) ;
#10528=ORIENTED_EDGE ( 'NONE', *, *, #37995, .F. ) ;
#10537=CARTESIAN_POINT ( 'NONE',  ( -12.70000000000000462, 81.72090770373000623, 129.9368274816651194 ) ) ;
#10567=CYLINDRICAL_SURFACE ( 'NONE', #14289, 7.937500000000000000 ) ;
#10568=ORIENTED_EDGE ( 'NONE', *, *, #78704, .T. ) ;
#10573=FACE_OUTER_BOUND ( 'NONE', #30474, .T. ) ;
#10575=DIRECTION ( 'NONE',  ( 0.8660254037844384856, 0.000000000000000000, -0.5000000000000003331 ) ) ;
#10592=CARTESIAN_POINT ( 'NONE',  ( 118.0058494126929816, 76.91656954603718077, -11.41259371393238098 ) ) ;
#10594=AXIS2_PLACEMENT_3D ( 'NONE', #30255, #85680, #65651 ) ;
#10599=VERTEX_POINT ( 'NONE', #77410 ) ;
#10607=ORIENTED_EDGE ( 'NONE', *, *, #13627, .F. ) ;
#10611=CARTESIAN_POINT ( 'NONE',  ( -4.481911866145203760, 70.65984535152513502, 118.4718773200152384 ) ) ;
#10627=EDGE_LOOP ( 'NONE', ( #85791, #64927, #18024, #74144 ) ) ;
#10630=CIRCLE ( 'NONE', #80298, 5.041900000000001825 ) ;
#10654=CARTESIAN_POINT ( 'NONE',  ( -97.46299999999992281, 82.54999999999999716, -12.70000000000034035 ) ) ;
#10704=CARTESIAN_POINT ( 'NONE',  ( 9.549815870737170087, 90.93248498521381862, 130.2065322450557119 ) ) ;
#10710=EDGE_CURVE ( 'NONE', #64009, #56554, #36964, .T. ) ;
#10713=ORIENTED_EDGE ( 'NONE', *, *, #42100, .F. ) ;
#10722=LINE ( 'NONE', #12079, #60272 ) ;
#10738=EDGE_LOOP ( 'NONE', ( #44986, #19954, #54006, #64514 ) ) ;
#10746=AXIS2_PLACEMENT_3D ( 'NONE', #25629, #18818, #53305 ) ;
#10755=CARTESIAN_POINT ( 'NONE',  ( 33.98325472291465132, 111.1250000000000000, -3.174999999999999822 ) ) ;
#10769=CARTESIAN_POINT ( 'NONE',  ( 84.20430400022883077, 76.20343663217362007, 99.77245543246509385 ) ) ;
#10775=CONICAL_SURFACE ( 'NONE', #77518, 24.63800000000000168, 0.7853981633974710386 ) ;
#10790=CARTESIAN_POINT ( 'NONE',  ( 77.69145367648738443, 73.00424585431355240, 89.55259891852641374 ) ) ;
#10799=EDGE_CURVE ( 'NONE', #81090, #79139, #89250, .T. ) ;
#10801=CARTESIAN_POINT ( 'NONE',  ( 117.8827734314469637, 84.21498941703524110, -12.61757617297137024 ) ) ;
#10809=ORIENTED_EDGE ( 'NONE', *, *, #43096, .F. ) ;
#10815=DIRECTION ( 'NONE',  ( 0.000000000000000000, -1.000000000000000000, 0.000000000000000000 ) ) ;
#10823=EDGE_CURVE ( 'NONE', #73627, #67094, #54581, .T. ) ;
#10828=ADVANCED_FACE ( 'NONE', ( #26464 ), #40079, .F. ) ;
#10835=DIRECTION ( 'NONE',  ( 1.000000000000000000, 0.000000000000000000, -3.406823656978775284E-15 ) ) ;
#10849=VECTOR ( 'NONE', #56822, 1000.000000000000000 ) ;
#10878=CARTESIAN_POINT ( 'NONE',  ( 4.163101094985349692E-14, 120.6499999999999915, -107.7702177616926065 ) ) ;
#10879=LINE ( 'NONE', #66276, #24662 ) ;
#10920=EDGE_LOOP ( 'NONE', ( #86351, #45913 ) ) ;
#10922=EDGE_LOOP ( 'NONE', ( #27485, #15450 ) ) ;
#10927=PLANE ( 'NONE',  #66769 ) ;
#10935=FACE_OUTER_BOUND ( 'NONE', #80727, .T. ) ;
#10965=VECTOR ( 'NONE', #17412, 1000.000000000000000 ) ;
#10974=VERTEX_POINT ( 'NONE', #42752 ) ;
#10975=CARTESIAN_POINT ( 'NONE',  ( -90.13186587200952715, 73.86197090048101188, -77.01855645442566356 ) ) ;
#11002=DIRECTION ( 'NONE',  ( 0.000000000000000000, 0.000000000000000000, 1.000000000000000000 ) ) ;
#11006=EDGE_LOOP ( 'NONE', ( #34465, #44985 ) ) ;
#11023=CARTESIAN_POINT ( 'NONE',  ( -83.15068351451286333, 79.66695435136418268, 100.6520717229721527 ) ) ;
#11026=ORIENTED_EDGE ( 'NONE', *, *, #63567, .F. ) ;
#11033=AXIS2_PLACEMENT_3D ( 'NONE', #48667, #83225, #89591 ) ;
#11040=CARTESIAN_POINT ( 'NONE',  ( 118.5214188546241161, 70.17671898886891313, 2.891923471344727492 ) ) ;
#11059=CARTESIAN_POINT ( 'NONE',  ( -10.79070278320184073, 75.83992121942911524, 118.0641357957730264 ) ) ;
#11073=FACE_OUTER_BOUND ( 'NONE', #82463, .T. ) ;
#11092=DIRECTION ( 'NONE',  ( 0.000000000000000000, -1.000000000000000000, 0.000000000000000000 ) ) ;
#11099=CARTESIAN_POINT ( 'NONE',  ( 77.39114642429899504, 120.6499999999999915, 71.77848634863160271 ) ) ;
#11103=LINE ( 'NONE', #4305, #16946 ) ;
#11105=CARTESIAN_POINT ( 'NONE',  ( 1.451892247740217613E-14, 95.25000000000000000, -118.5560000000000116 ) ) ;
#11116=LINE ( 'NONE', #65640, #8814 ) ;
#11118=CARTESIAN_POINT ( 'NONE',  ( 76.20505178924389611, 127.0000000000000000, -76.20505178924359768 ) ) ;
#11121=ORIENTED_EDGE ( 'NONE', *, *, #64702, .T. ) ;
#11146=CARTESIAN_POINT ( 'NONE',  ( 79.76258624986769519, 93.94553785444269067, 87.71311422381614875 ) ) ;
#11153=VECTOR ( 'NONE', #16238, 1000.000000000000000 ) ;
#11157=AXIS2_PLACEMENT_3D ( 'NONE', #75968, #60072, #27363 ) ;
#11175=ORIENTED_EDGE ( 'NONE', *, *, #50407, .F. ) ;
#11187=CARTESIAN_POINT ( 'NONE',  ( -72.96458098368751166, 127.0000000000000000, 72.96458098368620426 ) ) ;
#11196=B_SPLINE_CURVE_WITH_KNOTS ( 'NONE', 3,
 ( #58504, #45314, #81222, #52560, #67115, #24452, #38506, #74387, #4451, #65762, #52116, #66207, #53454, #3549, #81668, #74835, #46198, #38955, #60735, #60288, #45747, #26228, #3997, #53906, #31244, #5347, #58943, #86681, #24894, #19418, #18970, #59393, #47099, #12160, #79881, #59838, #73934, #38074, #25328, #18065, #11715, #80319, #17634, #73030, #87568, #39408, #10801, #39847, #31697 ),
 .UNSPECIFIED., .F., .F.,
 ( 4, 2, 2, 2, 2, 2, 2, 2, 2, 2, 2, 2, 2, 2, 2, 1, 2, 2, 2, 2, 2, 2, 2, 2, 4 ),
 ( 0.01987186023414422298, 0.02111356671950568101, 0.02235527320486713557, 0.02483868617559004816, 0.02608039266095152353, 0.02732209914631299891, 0.02980551211703595313, 0.03228892508775890735, 0.03353063157312036885, 0.03477233805848183035, 0.03725575102920476722, 0.03849745751456623566, 0.03973916399992770410, 0.04222257697065064097, 0.04346428345601210247, 0.04470598994137356397, 0.04594769642673503240, 0.04718940291209650084, 0.04967281588281945159, 0.05091452236818090615, 0.05215622885354237459, 0.05463964182426532534, 0.05588134830962680072, 0.05712305479498827609, 0.05960646776571126848 ),
 .UNSPECIFIED. ) ;
#11199=ADVANCED_FACE ( 'NONE', ( #31815, #59510 ), #87245, .T. ) ;
#11205=DIRECTION ( 'NONE',  ( 0.000000000000000000, -1.000000000000000000, 0.000000000000000000 ) ) ;
#11207=CARTESIAN_POINT ( 'NONE',  ( -3.968749999999935163, 127.0000000000000000, -100.8961411191535973 ) ) ;
#11232=VERTEX_POINT ( 'NONE', #11381 ) ;
#11236=DIRECTION ( 'NONE',  ( 0.000000000000000000, 1.000000000000000000, 0.000000000000000000 ) ) ;
#11241=LINE ( 'NONE', #38943, #77270 ) ;
#11274=ORIENTED_EDGE ( 'NONE', *, *, #34069, .T. ) ;
#11284=CIRCLE ( 'NONE', #54777, 88.90000000000000568 ) ;
#11286=CIRCLE ( 'NONE', #62065, 34.13125000000000142 ) ;
#11287=CARTESIAN_POINT ( 'NONE',  ( -118.5108917117887444, 70.27763793881261734, -3.294392537550126843 ) ) ;
#11291=VECTOR ( 'NONE', #54812, 1000.000000000000000 ) ;
#11321=ORIENTED_EDGE ( 'NONE', *, *, #89703, .T. ) ;
#11327=VERTEX_POINT ( 'NONE', #74950 ) ;
#11330=DIRECTION ( 'NONE',  ( -1.000000000000000000, 0.000000000000000000, -3.491483361109379305E-15 ) ) ;
#11334=CARTESIAN_POINT ( 'NONE',  ( -130.0420937742006515, 87.79544278253749212, -11.57361518220400676 ) ) ;
#11336=CIRCLE ( 'NONE', #15763, 5.041900000000001825 ) ;
#11353=CARTESIAN_POINT ( 'NONE',  ( -4.101352651117800896, 70.52330563318118095, -118.4857037620892726 ) ) ;
#11361=ADVANCED_FACE ( 'NONE', ( #32257 ), #19531, .F. ) ;
#11381=CARTESIAN_POINT ( 'NONE',  ( -72.96458098368751166, 101.5999999999999943, 78.00648098368618832 ) ) ;
#11413=ORIENTED_EDGE ( 'NONE', *, *, #27843, .T. ) ;
#11414=AXIS2_PLACEMENT_3D ( 'NONE', #56568, #62932, #83395 ) ;
#11431=VECTOR ( 'NONE', #56063, 1000.000000000000000 ) ;
#11432=ADVANCED_FACE ( 'NONE', ( #22689 ), #64015, .F. ) ;
#11433=CARTESIAN_POINT ( 'NONE',  ( -91.26337341211424814, 76.18740257834565455, -75.67519899969691721 ) ) ;
#11438=LINE ( 'NONE', #45478, #21441 ) ;
#11449=( NAMED_UNIT ( * ) PLANE_ANGLE_UNIT ( ) SI_UNIT ( $, .RADIAN. ) );
#11470=FACE_BOUND ( 'NONE', #76767, .T. ) ;
#11484=EDGE_CURVE ( 'NONE', #24458, #5511, #8477, .T. ) ;
#11504=CARTESIAN_POINT ( 'NONE',  ( -98.60478223830740774, 120.6499999999999915, -1.074461880482445986E-12 ) ) ;
#11508=CARTESIAN_POINT ( 'NONE',  ( -72.96458098368600531, 127.0000000000000000, -72.96458098368781009 ) ) ;
#11514=VECTOR ( 'NONE', #39679, 1000.000000000000000 ) ;
#11574=CARTESIAN_POINT ( 'NONE',  ( -10.08084112162953616, 90.28574336371696063, -118.1269349842563088 ) ) ;
#11613=CARTESIAN_POINT ( 'NONE',  ( 92.27768215249926698, 84.21498941703525531, 74.43373480440783396 ) ) ;
#11652=FACE_OUTER_BOUND ( 'NONE', #86235, .T. ) ;
#11661=ORIENTED_EDGE ( 'NONE', *, *, #40449, .F. ) ;
#11688=CARTESIAN_POINT ( 'NONE',  ( 6.714856022345344400, 93.33757043186105307, -130.3836582748265869 ) ) ;
#11711=DIRECTION ( 'NONE',  ( 0.2588190451025269012, 0.000000000000000000, -0.9659258262890665359 ) ) ;
#11715=CARTESIAN_POINT ( 'NONE',  ( 118.0434137139726829, 88.91291927174619047, -11.02232302911373196 ) ) ;
#11755=CYLINDRICAL_SURFACE ( 'NONE', #44711, 42.54500000000000171 ) ;
#11784=CARTESIAN_POINT ( 'NONE',  ( 103.1875000000000000, 117.4749999999999943, 3.602774393244745134E-13 ) ) ;
#11790=CARTESIAN_POINT ( 'NONE',  ( -130.3837941446097375, 93.33921197991992358, -6.712224447894871382 ) ) ;
#11809=CARTESIAN_POINT ( 'NONE',  ( -12.69999999999999929, 81.71107837960109066, -117.8738102209307499 ) ) ;
#11810=CARTESIAN_POINT ( 'NONE',  ( -129.9368274816651478, 82.54999999999999716, 12.69999999999954809 ) ) ;
#11817=EDGE_LOOP ( 'NONE', ( #27174, #2365, #77163, #58800 ) ) ;
#11831=DIRECTION ( 'NONE',  ( -0.5000000000000061062, 0.000000000000000000, 0.8660254037844351549 ) ) ;
#11837=ORIENTED_EDGE ( 'NONE', *, *, #65372, .F. ) ;
#11862=DIRECTION ( 'NONE',  ( 0.000000000000000000, 1.000000000000000000, 0.000000000000000000 ) ) ;
#11870=CARTESIAN_POINT ( 'NONE',  ( 130.5540562089606738, 95.23006786499114185, 0.8254869398584661067 ) ) ;
#11887=ADVANCED_FACE ( 'NONE', ( #56627 ), #76184, .F. ) ;
#11903=LINE ( 'NONE', #80960, #35481 ) ;
#11929=VECTOR ( 'NONE', #47454, 1000.000000000000000 ) ;
#11944=ADVANCED_FACE ( 'NONE', ( #62554 ), #20339, .F. ) ;
#11952=DIRECTION ( 'NONE',  ( -3.386875084296745512E-15, 0.000000000000000000, 1.000000000000000000 ) ) ;
#11957=CARTESIAN_POINT ( 'NONE',  ( -95.16685018566032284, 70.52074417248462623, -89.37727808479068869 ) ) ;
#11963=EDGE_LOOP ( 'NONE', ( #25263, #37882, #61119, #52904 ) ) ;
#11965=EDGE_CURVE ( 'NONE', #20160, #8910, #21231, .T. ) ;
#11982=VERTEX_POINT ( 'NONE', #43890 ) ;
#12018=CARTESIAN_POINT ( 'NONE',  ( -12.37521547983011416, 85.43365698736769787, -117.9083787315452412 ) ) ;
#12034=VERTEX_POINT ( 'NONE', #16212 ) ;
#12051=CARTESIAN_POINT ( 'NONE',  ( 7.399926448127667200, 72.22026871922481916, -130.3465752436562468 ) ) ;
#12052=EDGE_CURVE ( 'NONE', #18138, #10974, #65881, .T. ) ;
#12055=CARTESIAN_POINT ( 'NONE',  ( 83.54193218351797157, 95.25015226514366873, 84.12159398442744873 ) ) ;
#12074=ORIENTED_EDGE ( 'NONE', *, *, #67423, .F. ) ;
#12075=EDGE_LOOP ( 'NONE', ( #50675, #40179 ) ) ;
#12079=CARTESIAN_POINT ( 'NONE',  ( 103.1875000000000000, 127.0000000000000000, 5.041900000000359761 ) ) ;
#12097=CARTESIAN_POINT ( 'NONE',  ( 130.0003553321328411, 78.46683822717001533, -12.03293382262373612 ) ) ;
#12104=CARTESIAN_POINT ( 'NONE',  ( 0.000000000000000000, 82.54999999999999716, -97.46299999999996544 ) ) ;
#12122=ORIENTED_EDGE ( 'NONE', *, *, #88683, .F. ) ;
#12127=CARTESIAN_POINT ( 'NONE',  ( 2.077912807000529050, 95.08573034283288905, -130.5400978111108543 ) ) ;
#12135=APPLICATION_CONTEXT ( 'automotive_design' ) ;
#12138=EDGE_LOOP ( 'NONE', ( #53444, #41076, #47228, #65655 ) ) ;
#12140=DIRECTION ( 'NONE',  ( 0.000000000000000000, 0.000000000000000000, -1.000000000000000000 ) ) ;
#12160=CARTESIAN_POINT ( 'NONE',  ( 118.3662777621133131, 93.33860577356861654, -6.713439888429178382 ) ) ;
#12192=ORIENTED_EDGE ( 'NONE', *, *, #51682, .T. ) ;
#12205=VERTEX_POINT ( 'NONE', #67348 ) ;
#12236=CARTESIAN_POINT ( 'NONE',  ( -130.4354318373311514, 93.94566094357735153, -5.621620364686718219 ) ) ;
#12246=CARTESIAN_POINT ( 'NONE',  ( 72.96458098368701428, 127.0000000000000000, -67.92268098368680285 ) ) ;
#12261=ADVANCED_FACE ( 'NONE', ( #60992 ), #88720, .F. ) ;
#12265=CARTESIAN_POINT ( 'NONE',  ( -77.39114642430010349, 120.6499999999999915, 71.77848634863050847 ) ) ;
#12276=CARTESIAN_POINT ( 'NONE',  ( -118.2605848834651709, 92.12496802699141085, -8.385272115321491526 ) ) ;
#12282=VERTEX_POINT ( 'NONE', #77770 ) ;
#12317=ORIENTED_EDGE ( 'NONE', *, *, #13689, .F. ) ;
#12323=AXIS2_PLACEMENT_3D ( 'NONE', #6207, #33895, #35686 ) ;
#12338=LINE ( 'NONE', #38248, #66885 ) ;
#12346=( NAMED_UNIT ( * ) PLANE_ANGLE_UNIT ( ) SI_UNIT ( $, .RADIAN. ) );
#12353=DIRECTION ( 'NONE',  ( 0.000000000000000000, 1.000000000000000000, 0.000000000000000000 ) ) ;
#12359=CARTESIAN_POINT ( 'NONE',  ( 0.000000000000000000, 198.8420489685532004, 0.000000000000000000 ) ) ;
#12360=CARTESIAN_POINT ( 'NONE',  ( -105.4788588808462038, 120.6499999999999915, -3.968750000001139977 ) ) ;
#12362=AXIS2_PLACEMENT_3D ( 'NONE', #17378, #43278, #31437 ) ;
#12394=VERTEX_POINT ( 'NONE', #28251 ) ;
#12399=AXIS2_PLACEMENT_3D ( 'NONE', #70366, #8599, #36296 ) ;
#12421=VERTEX_POINT ( 'NONE', #84597 ) ;
#12422=VERTEX_POINT ( 'NONE', #69609 ) ;
#12456=EDGE_CURVE ( 'NONE', #59338, #79094, #65470, .T. ) ;
#12460=CARTESIAN_POINT ( 'NONE',  ( -71.77848634863190114, 127.0000000000000000, 77.39114642429879609 ) ) ;
#12469=DIRECTION ( 'NONE',  ( -0.9659258262890677571, 0.000000000000000000, 0.2588190451025230154 ) ) ;
#12480=ORIENTED_EDGE ( 'NONE', *, *, #88901, .F. ) ;
#12488=EDGE_CURVE ( 'NONE', #41468, #89588, #44111, .T. ) ;
#12490=DIRECTION ( 'NONE',  ( 0.000000000000000000, 1.000000000000000000, 0.000000000000000000 ) ) ;
#12494=VERTEX_POINT ( 'NONE', #10067 ) ;
#12501=CARTESIAN_POINT ( 'NONE',  ( 0.000000000000000000, 103.1240000000000236, 0.000000000000000000 ) ) ;
#12513=PLANE ( 'NONE',  #66401 ) ;
#12547=CARTESIAN_POINT ( 'NONE',  ( 130.2063869749195248, 74.16976894168006140, -9.551794474070780083 ) ) ;
#12555=CARTESIAN_POINT ( 'NONE',  ( 3.968750000000000000, 127.0000000000000000, -105.4788588808464027 ) ) ;
#12570=CARTESIAN_POINT ( 'NONE',  ( -3.175000000000120171, 104.3431970271541900, 33.98325472291460159 ) ) ;
#12581=CARTESIAN_POINT ( 'NONE',  ( 0.000000000000000000, 101.5999999999999943, 0.000000000000000000 ) ) ;
#12597=DIRECTION ( 'NONE',  ( -1.047445008332813989E-14, 0.000000000000000000, 1.000000000000000000 ) ) ;
#12601=ORIENTED_EDGE ( 'NONE', *, *, #4887, .T. ) ;
#12650=CARTESIAN_POINT ( 'NONE',  ( 3.286821707691937711, 70.27560252132435892, -118.5111027017741776 ) ) ;
#12655=VECTOR ( 'NONE', #37496, 1000.000000000000000 ) ;
#12679=EDGE_CURVE ( 'NONE', #75690, #9436, #48809, .T. ) ;
#12706=DIRECTION ( 'NONE',  ( 0.000000000000000000, 1.000000000000000000, 0.000000000000000000 ) ) ;
#12731=CARTESIAN_POINT ( 'NONE',  ( -118.4880192609368947, 94.60304557064718267, -4.087421425392933294 ) ) ;
#12737=CARTESIAN_POINT ( 'NONE',  ( 4.665904304751420031E-15, 95.25000000000000000, -38.10000000000000142 ) ) ;
#12749=AXIS2_PLACEMENT_3D ( 'NONE', #12104, #40242, #54747 ) ;
#12752=CARTESIAN_POINT ( 'NONE',  ( 92.32962665258611423, 82.96450994655477018, -74.36911441044638593 ) ) ;
#12753=VECTOR ( 'NONE', #82566, 1000.000000000000000 ) ;
#12769=CARTESIAN_POINT ( 'NONE',  ( 130.5169520046878802, 94.84315624882771090, 3.295103719955264410 ) ) ;
#12790=VERTEX_POINT ( 'NONE', #84788 ) ;
#12810=VERTEX_POINT ( 'NONE', #15738 ) ;
#12814=VECTOR ( 'NONE', #41519, 1000.000000000000000 ) ;
#12817=ORIENTED_EDGE ( 'NONE', *, *, #54071, .F. ) ;
#12829=ORIENTED_EDGE ( 'NONE', *, *, #28589, .T. ) ;
#12836=CARTESIAN_POINT ( 'NONE',  ( -100.4321520267694723, 78.46444036551649504, 83.41622542100928683 ) ) ;
#12849=DIRECTION ( 'NONE',  ( 0.000000000000000000, -1.000000000000000000, 0.000000000000000000 ) ) ;
#12851=DIRECTION ( 'NONE',  ( 0.000000000000000000, -1.000000000000000000, 0.000000000000000000 ) ) ;
#12865=ORIENTED_EDGE ( 'NONE', *, *, #57036, .T. ) ;
#12871=FACE_OUTER_BOUND ( 'NONE', #84976, .T. ) ;
#12878=ORIENTED_EDGE ( 'NONE', *, *, #10171, .F. ) ;
#12879=LINE ( 'NONE', #42338, #1606 ) ;
#12886=DIRECTION ( 'NONE',  ( 0.000000000000000000, -1.000000000000000000, 0.000000000000000000 ) ) ;
#12894=EDGE_CURVE ( 'NONE', #8142, #5023, #2102, .T. ) ;
#12907=LINE ( 'NONE', #89211, #2184 ) ;
#12929=AXIS2_PLACEMENT_3D ( 'NONE', #80757, #46195, #39841 ) ;
#12931=ORIENTED_EDGE ( 'NONE', *, *, #61487, .T. ) ;
#12957=CARTESIAN_POINT ( 'NONE',  ( 82.65057572782268380, 95.14807216649717247, 84.99753727674189463 ) ) ;
#12964=CARTESIAN_POINT ( 'NONE',  ( -83.76986456925402535, 87.79544278253753475, -100.1374281256143774 ) ) ;
#12971=ORIENTED_EDGE ( 'NONE', *, *, #41562, .F. ) ;
#12993=CIRCLE ( 'NONE', #24592, 188.9759999999999991 ) ;
#13029=CARTESIAN_POINT ( 'NONE',  ( -33.98325472291460159, 104.3431970271541900, -3.175000000000234746 ) ) ;
#13064=DIRECTION ( 'NONE',  ( 0.000000000000000000, 0.000000000000000000, -1.000000000000000000 ) ) ;
#13071=CARTESIAN_POINT ( 'NONE',  ( -100.8961411191535973, 120.6499999999999915, -3.968750000001104894 ) ) ;
#13092=CARTESIAN_POINT ( 'NONE',  ( 0.000000000000000000, 92.07499999999998863, 38.10000000000000142 ) ) ;
#13093=ORIENTED_EDGE ( 'NONE', *, *, #16668, .F. ) ;
#13094=CARTESIAN_POINT ( 'NONE',  ( -118.0068565116053492, 76.93600387762168680, -11.39936611905761765 ) ) ;
#13098=EDGE_CURVE ( 'NONE', #36775, #1670, #54379, .T. ) ;
#13107=EDGE_CURVE ( 'NONE', #41269, #52484, #16961, .T. ) ;
#13111=CIRCLE ( 'NONE', #34875, 7.937500000000000000 ) ;
#13150=CARTESIAN_POINT ( 'NONE',  ( 88.25806911646408537, 93.94653598907717651, -96.20559720633534084 ) ) ;
#13154=CARTESIAN_POINT ( 'NONE',  ( -12.37563412544579045, 79.66819247178165142, -117.9083347083516173 ) ) ;
#13164=AXIS2_PLACEMENT_3D ( 'NONE', #12501, #46545, #40183 ) ;
#13183=ADVANCED_FACE ( 'NONE', ( #88695, #46863, #31461, #74155 ), #26007, .T. ) ;
#13202=ORIENTED_EDGE ( 'NONE', *, *, #7479, .T. ) ;
#13210=VECTOR ( 'NONE', #62515, 1000.000000000000000 ) ;
#13215=VERTEX_POINT ( 'NONE', #80992 ) ;
#13232=CARTESIAN_POINT ( 'NONE',  ( -74.43211355457115985, 80.89685143461889538, -92.27899210470897629 ) ) ;
#13233=ORIENTED_EDGE ( 'NONE', *, *, #32084, .F. ) ;
#13242=DIRECTION ( 'NONE',  ( -0.9659258262890683122, 0.000000000000000000, -0.2588190451025206285 ) ) ;
#13266=EDGE_LOOP ( 'NONE', ( #57137, #5513, #77517, #65801 ) ) ;
#13270=FACE_OUTER_BOUND ( 'NONE', #11963, .T. ) ;
#13293=DIRECTION ( 'NONE',  ( 1.000000000000000000, 0.000000000000000000, 3.386875084296745512E-15 ) ) ;
#13297=EDGE_CURVE ( 'NONE', #38056, #18286, #41263, .T. ) ;
#13298=CARTESIAN_POINT ( 'NONE',  ( -89.95878776288222411, 70.27756284692561906, -94.61736061587636470 ) ) ;
#13302=VECTOR ( 'NONE', #41048, 1000.000000000000114 ) ;
#13317=ORIENTED_EDGE ( 'NONE', *, *, #23098, .F. ) ;
#13320=EDGE_LOOP ( 'NONE', ( #89844, #38638, #7047, #74510 ) ) ;
#13338=ADVANCED_FACE ( 'NONE', ( #20984 ), #35489, .F. ) ;
#13343=ORIENTED_EDGE ( 'NONE', *, *, #80925, .F. ) ;
#13361=CARTESIAN_POINT ( 'NONE',  ( -74.15067561874160162, 120.6499999999999915, -68.53801554307528932 ) ) ;
#13384=CARTESIAN_POINT ( 'NONE',  ( -91.90683392111071726, 78.46407912418315789, 74.89107914305792235 ) ) ;
#13420=ORIENTED_EDGE ( 'NONE', *, *, #74747, .F. ) ;
#13442=CARTESIAN_POINT ( 'NONE',  ( 130.4667014434020587, 70.80031561532533146, -4.873084245995139341 ) ) ;
#13467=CARTESIAN_POINT ( 'NONE',  ( 0.000000000000000000, 127.0000000000000000, -103.1875000000000000 ) ) ;
#13501=CARTESIAN_POINT ( 'NONE',  ( -68.53801554307499089, 127.0000000000000000, 74.15067561874188584 ) ) ;
#13536=FACE_OUTER_BOUND ( 'NONE', #56481, .T. ) ;
#13547=ORIENTED_EDGE ( 'NONE', *, *, #62194, .T. ) ;
#13571=CARTESIAN_POINT ( 'NONE',  ( 95.16685018565972598, 70.52074417248462623, 89.37727808479131397 ) ) ;
#13585=CARTESIAN_POINT ( 'NONE',  ( 89.37916159652658621, 94.58014758961626001, -95.16508291382855589 ) ) ;
#13587=ADVANCED_FACE ( 'NONE', ( #60399 ), #29853, .T. ) ;
#13590=CARTESIAN_POINT ( 'NONE',  ( 92.32962665258456525, 82.54999999999999716, 74.36911441044829019 ) ) ;
#13594=VECTOR ( 'NONE', #56979, 1000.000000000000000 ) ;
#13613=CIRCLE ( 'NONE', #51331, 7.143750000000004263 ) ;
#13617=FACE_OUTER_BOUND ( 'NONE', #16548, .T. ) ;
#13627=EDGE_CURVE ( 'NONE', #44525, #64446, #65876, .T. ) ;
#13628=CARTESIAN_POINT ( 'NONE',  ( -117.8738102209307925, 82.54999999999999716, 12.69999999999959073 ) ) ;
#13633=EDGE_CURVE ( 'NONE', #84986, #66271, #66077, .T. ) ;
#13644=ORIENTED_EDGE ( 'NONE', *, *, #8097, .T. ) ;
#13646=ORIENTED_EDGE ( 'NONE', *, *, #50507, .F. ) ;
#13671=CARTESIAN_POINT ( 'NONE',  ( -85.85227416678151258, 70.17658267799284033, -81.76234319299396702 ) ) ;
#13673=DIRECTION ( 'NONE',  ( 0.000000000000000000, 0.000000000000000000, -1.000000000000000000 ) ) ;
#13678=CYLINDRICAL_SURFACE ( 'NONE', #14713, 12.70000000000000107 ) ;
#13684=CARTESIAN_POINT ( 'NONE',  ( 98.83784439188674753, 74.16222525595216553, -85.30119219530038777 ) ) ;
#13689=EDGE_CURVE ( 'NONE', #77431, #13215, #47213, .T. ) ;
#13692=CARTESIAN_POINT ( 'NONE',  ( 5.627926923415666138, 71.15750911566317427, 118.4229113093306438 ) ) ;
#13698=CARTESIAN_POINT ( 'NONE',  ( 103.1875000000000000, 127.0000000000000000, 7.937500000000360600 ) ) ;
#13719=CARTESIAN_POINT ( 'NONE',  ( -98.83784439188610804, 74.16222525595216553, 85.30119219530108410 ) ) ;
#13735=EDGE_LOOP ( 'NONE', ( #88204, #30000 ) ) ;
#13738=CARTESIAN_POINT ( 'NONE',  ( -99.78212687779739554, 76.18750001922978754, -84.19388261208001722 ) ) ;
#13739=CARTESIAN_POINT ( 'NONE',  ( -74.49778344313841671, 84.62843115047675724, -92.22587532767836649 ) ) ;
#13746=DIRECTION ( 'NONE',  ( 0.000000000000000000, 0.000000000000000000, 1.000000000000000000 ) ) ;
#13776=DIRECTION ( 'NONE',  ( 1.000000000000000000, 0.000000000000000000, 0.000000000000000000 ) ) ;
#13809=DIRECTION ( 'NONE',  ( 0.000000000000000000, 0.000000000000000000, -1.000000000000000000 ) ) ;
#13811=VECTOR ( 'NONE', #87286, 1000.000000000000000 ) ;
#13825=CARTESIAN_POINT ( 'NONE',  ( -89.12695577293538918, 72.47328848629025799, 78.17938156622544454 ) ) ;
#13841=DIRECTION ( 'NONE',  ( 0.000000000000000000, 1.000000000000000000, 0.000000000000000000 ) ) ;
#13850=CARTESIAN_POINT ( 'NONE',  ( -87.71306776503853087, 93.55256755804782642, -96.70275196374447546 ) ) ;
#13856=AXIS2_PLACEMENT_3D ( 'NONE', #6537, #168, #82864 ) ;
#13859=VERTEX_POINT ( 'NONE', #3894 ) ;
#13872=EDGE_CURVE ( 'NONE', #1794, #14083, #54445, .T. ) ;
#13884=LINE ( 'NONE', #15691, #82014 ) ;
#13904=ADVANCED_FACE ( 'NONE', ( #52455 ), #43536, .F. ) ;
#13909=CARTESIAN_POINT ( 'NONE',  ( -7.205548786489490269E-13, 117.4749999999999943, 103.1875000000000000 ) ) ;
#13931=ADVANCED_FACE ( 'NONE', ( #1332, #57163 ), #875, .F. ) ;
#13933=CARTESIAN_POINT ( 'NONE',  ( 0.000000000000000000, 127.0000000000000000, -103.1875000000000000 ) ) ;
#13938=LINE ( 'NONE', #41617, #27252 ) ;
#13963=DIRECTION ( 'NONE',  ( 0.000000000000000000, 1.000000000000000000, 0.000000000000000000 ) ) ;
#13971=FACE_BOUND ( 'NONE', #43662, .T. ) ;
#13979=CARTESIAN_POINT ( 'NONE',  ( -117.8825533107840329, 80.89685143461892380, -12.61964884581497692 ) ) ;
#13995=VECTOR ( 'NONE', #50834, 1000.000000000000000 ) ;
#13997=DIRECTION ( 'NONE',  ( 0.000000000000000000, 0.000000000000000000, -1.000000000000000000 ) ) ;
#14011=DIRECTION ( 'NONE',  ( 0.000000000000000000, 0.000000000000000000, -1.000000000000000000 ) ) ;
#14014=ORIENTED_EDGE ( 'NONE', *, *, #29820, .T. ) ;
#14025=VECTOR ( 'NONE', #28705, 999.9999999999998863 ) ;
#14053=CYLINDRICAL_SURFACE ( 'NONE', #16826, 190.5000000000000000 ) ;
#14059=CARTESIAN_POINT ( 'NONE',  ( -92.32962665258561685, 82.96450994655479860, 74.36911441044702542 ) ) ;
#14065=CARTESIAN_POINT ( 'NONE',  ( 79.76251016565943530, 71.15456258041353976, -87.71317827224403629 ) ) ;
#14066=ORIENTED_EDGE ( 'NONE', *, *, #38915, .T. ) ;
#14077=DIRECTION ( 'NONE',  ( 0.000000000000000000, 0.000000000000000000, 1.000000000000000000 ) ) ;
#14082=CARTESIAN_POINT ( 'NONE',  ( 74.62309654709210349, 85.43299024555683729, -92.12450916458674044 ) ) ;
#14083=VERTEX_POINT ( 'NONE', #19316 ) ;
#14116=CARTESIAN_POINT ( 'NONE',  ( -0.8390482630167189759, 69.85000000000000853, -130.5560000000000400 ) ) ;
#14125=CARTESIAN_POINT ( 'NONE',  ( -75.68572508987513459, 76.20320268897033600, -91.25368348339026170 ) ) ;
#14127=VERTEX_POINT ( 'NONE', #25673 ) ;
#14138=CARTESIAN_POINT ( 'NONE',  ( 97.62852612868790914, 72.47310549519059464, -86.68128281353502018 ) ) ;
#14147=CARTESIAN_POINT ( 'NONE',  ( 11.41378189430731993, 76.91903266065129685, 118.0057337156638653 ) ) ;
#14158=ORIENTED_EDGE ( 'NONE', *, *, #25443, .F. ) ;
#14181=DIRECTION ( 'NONE',  ( 0.2588190451025229599, 0.000000000000000000, 0.9659258262890676461 ) ) ;
#14187=ORIENTED_EDGE ( 'NONE', *, *, #55005, .T. ) ;
#14189=CARTESIAN_POINT ( 'NONE',  ( -74.44936585838399878, 84.21376545118704371, -92.26493792250069248 ) ) ;
#14196=DIRECTION ( 'NONE',  ( 0.000000000000000000, 1.000000000000000000, 0.000000000000000000 ) ) ;
#14210=VECTOR ( 'NONE', #46712, 1000.000000000000000 ) ;
#14227=CARTESIAN_POINT ( 'NONE',  ( -68.53801554307339927, 120.6499999999999915, -74.15067561874339219 ) ) ;
#14234=LINE ( 'NONE', #69642, #75362 ) ;
#14255=EDGE_CURVE ( 'NONE', #76109, #24458, #22021, .T. ) ;
#14262=EDGE_CURVE ( 'NONE', #52873, #75590, #36536, .T. ) ;
#14282=CARTESIAN_POINT ( 'NONE',  ( -89.55259891852560372, 73.00424585431356661, 77.69145367648832234 ) ) ;
#14289=AXIS2_PLACEMENT_3D ( 'NONE', #5100, #73692, #46408 ) ;
#14306=CARTESIAN_POINT ( 'NONE',  ( 8.398107354775891764, 72.98722500879387098, 130.2869324835649536 ) ) ;
#14307=CARTESIAN_POINT ( 'NONE',  ( -98.64044413062988781, 91.23859726994547259, -85.52787878288694401 ) ) ;
#14312=EDGE_CURVE ( 'NONE', #24458, #77970, #43774, .T. ) ;
#14343=DIRECTION ( 'NONE',  ( 0.000000000000000000, 0.000000000000000000, -1.000000000000000000 ) ) ;
#14346=CARTESIAN_POINT ( 'NONE',  ( 130.5246120830809957, 70.17656663518269511, -2.891956274606212407 ) ) ;
#14380=ADVANCED_FACE ( 'NONE', ( #24678, #79666 ), #30603, .T. ) ;
#14389=ORIENTED_EDGE ( 'NONE', *, *, #12488, .T. ) ;
#14408=CARTESIAN_POINT ( 'NONE',  ( 99.17062120112595380, 90.28418055714728041, 84.91247172076124627 ) ) ;
#14416=CYLINDRICAL_SURFACE ( 'NONE', #30176, 7.143750000000004263 ) ;
#14431=EDGE_LOOP ( 'NONE', ( #80269, #20958 ) ) ;
#14440=CARTESIAN_POINT ( 'NONE',  ( -117.9723322394570886, 77.68452076096554038, -11.75283433610015393 ) ) ;
#14467=PLANE ( 'NONE',  #50913 ) ;
#14476=DIRECTION ( 'NONE',  ( 0.000000000000000000, 1.000000000000000000, 0.000000000000000000 ) ) ;
#14517=EDGE_LOOP ( 'NONE', ( #23403, #54023, #12865, #48013, #61076, #42978 ) ) ;
#14519=CARTESIAN_POINT ( 'NONE',  ( -82.65294504194682190, 95.16897323824359489, 84.99816483510906551 ) ) ;
#14525=CARTESIAN_POINT ( 'NONE',  ( 91.25368348339054592, 76.20320268897036442, -75.68572508987483616 ) ) ;
#14528=PLANE ( 'NONE',  #49871 ) ;
#14531=EDGE_LOOP ( 'NONE', ( #36126, #84180 ) ) ;
#14543=CARTESIAN_POINT ( 'NONE',  ( 76.39920031718088467, 90.28416741362499920, -90.65736737572389359 ) ) ;
#14550=VERTEX_POINT ( 'NONE', #66900 ) ;
#14557=DIRECTION ( 'NONE',  ( -0.9659258262890697555, 0.000000000000000000, 0.2588190451025154659 ) ) ;
#14583=CARTESIAN_POINT ( 'NONE',  ( -77.45828646618646474, 73.28361289573329884, -89.75424775947691103 ) ) ;
#14584=ORIENTED_EDGE ( 'NONE', *, *, #5103, .F. ) ;
#14625=CARTESIAN_POINT ( 'NONE',  ( -89.37727808479034763, 70.52074417248462623, 95.16685018566064969 ) ) ;
#14665=CIRCLE ( 'NONE', #36588, 7.937500000000000000 ) ;
#14671=AXIS2_PLACEMENT_3D ( 'NONE', #40378, #39923, #53981 ) ;
#14683=DIRECTION ( 'NONE',  ( 0.000000000000000000, 1.000000000000000000, 0.000000000000000000 ) ) ;
#14685=LINE ( 'NONE', #62809, #31897 ) ;
#14691=EDGE_LOOP ( 'NONE', ( #28356, #4205 ) ) ;
#14701=CARTESIAN_POINT ( 'NONE',  ( 2.078103260390294693, 95.08570091005915970, -118.5384849238115947 ) ) ;
#14713=AXIS2_PLACEMENT_3D ( 'NONE', #42267, #48616, #20512 ) ;
#14724=EDGE_CURVE ( 'NONE', #7172, #40430, #63224, .T. ) ;
#14735=CARTESIAN_POINT ( 'NONE',  ( -87.72765544449595154, 71.14137858619484689, 79.74945239053533896 ) ) ;
#14742=EDGE_CURVE ( 'NONE', #35450, #37737, #55935, .T. ) ;
#14801=CIRCLE ( 'NONE', #51020, 9.525000000000000355 ) ;
#14814=FACE_OUTER_BOUND ( 'NONE', #8504, .T. ) ;
#14815=PLANE ( 'NONE',  #46740 ) ;
#14817=CARTESIAN_POINT ( 'NONE',  ( 1.166476076187854022E-15, 92.07499999999998863, -9.525000000000000355 ) ) ;
#14859=CARTESIAN_POINT ( 'NONE',  ( -69.72411017812909506, 127.0000000000000000, -69.72411017813089984 ) ) ;
#14861=CARTESIAN_POINT ( 'NONE',  ( 100.8594679592200833, 82.54999999999999716, 82.89895571708400723 ) ) ;
#14862=LINE ( 'NONE', #63440, #84320 ) ;
#14878=VERTEX_POINT ( 'NONE', #72285 ) ;
#14884=CARTESIAN_POINT ( 'NONE',  ( -10.78716141056406208, 89.26551436951578467, 118.0644550036098224 ) ) ;
#14897=LINE ( 'NONE', #15344, #11153 ) ;
#14899=DIRECTION ( 'NONE',  ( 0.000000000000000000, 0.000000000000000000, 1.000000000000000000 ) ) ;
#14911=CARTESIAN_POINT ( 'NONE',  ( 117.8738102209308920, 82.54999999999999716, -12.69999999999876827 ) ) ;
#14917=FACE_BOUND ( 'NONE', #64909, .T. ) ;
#14942=CARTESIAN_POINT ( 'NONE',  ( -74.15067561874319324, 127.0000000000000000, 68.53801554307369770 ) ) ;
#14948=CYLINDRICAL_SURFACE ( 'NONE', #19597, 7.937500000000000000 ) ;
#14963=VERTEX_POINT ( 'NONE', #12737 ) ;
#14972=CARTESIAN_POINT ( 'NONE',  ( 80.31601416995117404, 70.80054593973557076, -87.20837843453648475 ) ) ;
#14988=CARTESIAN_POINT ( 'NONE',  ( 87.71311422381590717, 93.94553785444269067, -79.76258624986799362 ) ) ;
#14991=DIRECTION ( 'NONE',  ( 0.7071067811865389130, 0.000000000000000000, 0.7071067811865561215 ) ) ;
#15021=EDGE_LOOP ( 'NONE', ( #71099, #38880 ) ) ;
#15042=ADVANCED_FACE ( 'NONE', ( #26356 ), #5473, .T. ) ;
#15056=DIRECTION ( 'NONE',  ( 0.4999999999999986122, 0.000000000000000000, 0.8660254037844394848 ) ) ;
#15062=DIRECTION ( 'NONE',  ( 0.000000000000000000, 1.000000000000000000, 0.000000000000000000 ) ) ;
#15081=CARTESIAN_POINT ( 'NONE',  ( -107.7702177616926065, 127.0000000000000000, -1.170464777364108012E-12 ) ) ;
#15096=EDGE_CURVE ( 'NONE', #23774, #15841, #26665, .T. ) ;
#15130=DIRECTION ( 'NONE',  ( 1.000000000000000000, 0.000000000000000000, 0.000000000000000000 ) ) ;
#15131=AXIS2_PLACEMENT_3D ( 'NONE', #69828, #7601, #34848 ) ;
#15135=AXIS2_PLACEMENT_3D ( 'NONE', #2424, #16944, #44623 ) ;
#15140=LINE ( 'NONE', #77818, #30288 ) ;
#15144=CARTESIAN_POINT ( 'NONE',  ( 1.663885868249273425, 95.14749804389164467, -118.5450564992233780 ) ) ;
#15164=ADVANCED_FACE ( 'NONE', ( #76746 ), #14528, .F. ) ;
#15177=ORIENTED_EDGE ( 'NONE', *, *, #45132, .T. ) ;
#15178=ORIENTED_EDGE ( 'NONE', *, *, #84720, .F. ) ;
#15192=ORIENTED_EDGE ( 'NONE', *, *, #43096, .T. ) ;
#15194=CARTESIAN_POINT ( 'NONE',  ( 9.720633968232110273E-16, 117.4749999999999943, -111.1250000000000000 ) ) ;
#15208=ORIENTED_EDGE ( 'NONE', *, *, #31641, .T. ) ;
#15209=VECTOR ( 'NONE', #55992, 1000.000000000000114 ) ;
#15212=ORIENTED_EDGE ( 'NONE', *, *, #58715, .F. ) ;
#15224=DIRECTION ( 'NONE',  ( 0.8660254037844390407, 0.000000000000000000, -0.4999999999999995004 ) ) ;
#15236=DIRECTION ( 'NONE',  ( 0.000000000000000000, 0.000000000000000000, 1.000000000000000000 ) ) ;
#15244=PLANE ( 'NONE',  #54728 ) ;
#15270=PLANE ( 'NONE',  #2487 ) ;
#15276=ORIENTED_EDGE ( 'NONE', *, *, #30535, .F. ) ;
#15284=EDGE_CURVE ( 'NONE', #29629, #33210, #84731, .T. ) ;
#15291=CIRCLE ( 'NONE', #5152, 34.13125000000000142 ) ;
#15306=CARTESIAN_POINT ( 'NONE',  ( 95.69832483115182242, 94.30053025434482095, 88.80956239834469557 ) ) ;
#15308=CYLINDRICAL_SURFACE ( 'NONE', #66471, 7.143750000000004263 ) ;
#15322=CARTESIAN_POINT ( 'NONE',  ( -7.301849239715819957E-13, 127.0000000000000000, 98.60478223830740774 ) ) ;
#15336=EDGE_CURVE ( 'NONE', #79139, #29190, #36310, .T. ) ;
#15344=CARTESIAN_POINT ( 'NONE',  ( 3.968750000000000000, 120.6499999999999915, -105.4788588808464027 ) ) ;
#15388=ORIENTED_EDGE ( 'NONE', *, *, #33916, .T. ) ;
#15411=PLANE ( 'NONE',  #74801 ) ;
#15413=FACE_OUTER_BOUND ( 'NONE', #23540, .T. ) ;
#15427=CARTESIAN_POINT ( 'NONE',  ( 88.21655330423281782, 71.53193882405247450, -79.20758933349323172 ) ) ;
#15443=CARTESIAN_POINT ( 'NONE',  ( 80.88915705228910724, 94.58006533271583294, -86.67541640318093243 ) ) ;
#15450=ORIENTED_EDGE ( 'NONE', *, *, #26345, .T. ) ;
#15453=VERTEX_POINT ( 'NONE', #89383 ) ;
#15458=CARTESIAN_POINT ( 'NONE',  ( -72.96458098368751166, 117.4749999999999943, 80.10833098368618721 ) ) ;
#15470=AXIS2_PLACEMENT_3D ( 'NONE', #28187, #7320, #64851 ) ;
#15482=ORIENTED_EDGE ( 'NONE', *, *, #31641, .F. ) ;
#15492=AXIS2_PLACEMENT_3D ( 'NONE', #24273, #31509, #18788 ) ;
#15497=CARTESIAN_POINT ( 'NONE',  ( 84.19388261208037250, 76.18750001922980175, -99.78212687779711132 ) ) ;
#15504=DIRECTION ( 'NONE',  ( -0.2588190451025281225, 0.000000000000000000, 0.9659258262890663138 ) ) ;
#15518=CARTESIAN_POINT ( 'NONE',  ( -100.8961411191535973, 127.0000000000000000, -3.968750000001104894 ) ) ;
#15528=CIRCLE ( 'NONE', #11157, 7.937500000000000000 ) ;
#15534=DIRECTION ( 'NONE',  ( 3.596091637922019804E-15, 0.000000000000000000, 1.000000000000000000 ) ) ;
#15542=CARTESIAN_POINT ( 'NONE',  ( -75.24778849303618244, 87.79588542099533299, -91.61507027739561693 ) ) ;
#15545=DIRECTION ( 'NONE',  ( 0.000000000000000000, 1.000000000000000000, 0.000000000000000000 ) ) ;
#15554=EDGE_CURVE ( 'NONE', #14550, #27150, #61241, .T. ) ;
#15574=FACE_OUTER_BOUND ( 'NONE', #2043, .T. ) ;
#15584=CIRCLE ( 'NONE', #53202, 7.937500000000000000 ) ;
#15596=DIRECTION ( 'NONE',  ( 0.7071067811865415775, 0.000000000000000000, 0.7071067811865535679 ) ) ;
#15601=CARTESIAN_POINT ( 'NONE',  ( -9.572882853229330635, 90.93765695308124464, 130.2059221945669947 ) ) ;
#15612=FACE_OUTER_BOUND ( 'NONE', #63369, .T. ) ;
#15614=EDGE_CURVE ( 'NONE', #61529, #35450, #85273, .T. ) ;
#15618=ORIENTED_EDGE ( 'NONE', *, *, #58609, .T. ) ;
#15654=VECTOR ( 'NONE', #67201, 1000.000000000000000 ) ;
#15671=DIRECTION ( 'NONE',  ( -1.047445008332813989E-14, 0.000000000000000000, 1.000000000000000000 ) ) ;
#15682=ORIENTED_EDGE ( 'NONE', *, *, #57440, .F. ) ;
#15691=CARTESIAN_POINT ( 'NONE',  ( 1.088711004441995877E-14, 92.07499999999998863, -88.90000000000000568 ) ) ;
#15693=ORIENTED_EDGE ( 'NONE', *, *, #62002, .T. ) ;
#15707=CARTESIAN_POINT ( 'NONE',  ( 72.96458098368650269, 117.4749999999999943, 65.82083098368730134 ) ) ;
#15719=DIRECTION ( 'NONE',  ( 0.000000000000000000, -1.000000000000000000, 0.000000000000000000 ) ) ;
#15724=DIRECTION ( 'NONE',  ( 0.000000000000000000, 1.000000000000000000, 0.000000000000000000 ) ) ;
#15738=CARTESIAN_POINT ( 'NONE',  ( -76.20505178924449297, 120.6499999999999915, 76.20505178924310030 ) ) ;
#15748=DIRECTION ( 'NONE',  ( 0.000000000000000000, -1.000000000000000000, 0.000000000000000000 ) ) ;
#15757=ORIENTED_EDGE ( 'NONE', *, *, #50914, .T. ) ;
#15759=CARTESIAN_POINT ( 'NONE',  ( 76.20505178924389611, 120.6499999999999915, -76.20505178924359768 ) ) ;
#15763=AXIS2_PLACEMENT_3D ( 'NONE', #61072, #12490, #53786 ) ;
#15766=ORIENTED_EDGE ( 'NONE', *, *, #3352, .T. ) ;
#15770=ORIENTED_EDGE ( 'NONE', *, *, #10799, .T. ) ;
#15784=ORIENTED_EDGE ( 'NONE', *, *, #18613, .T. ) ;
#15788=CARTESIAN_POINT ( 'NONE',  ( 12.27293249669208919, 79.25788962028573792, -117.9191036749242301 ) ) ;
#15795=FACE_BOUND ( 'NONE', #58103, .T. ) ;
#15800=ORIENTED_EDGE ( 'NONE', *, *, #76985, .T. ) ;
#15801=ORIENTED_EDGE ( 'NONE', *, *, #13633, .F. ) ;
#15814=CARTESIAN_POINT ( 'NONE',  ( 71.77848634863140376, 127.0000000000000000, -77.39114642429929347 ) ) ;
#15832=CARTESIAN_POINT ( 'NONE',  ( 0.000000000000000000, 117.4749999999999943, -103.1875000000000000 ) ) ;
#15834=DIRECTION ( 'NONE',  ( 0.000000000000000000, 1.000000000000000000, 0.000000000000000000 ) ) ;
#15839=DIRECTION ( 'NONE',  ( 0.000000000000000000, -1.000000000000000000, 0.000000000000000000 ) ) ;
#15841=VERTEX_POINT ( 'NONE', #56859 ) ;
#15862=DIRECTION ( 'NONE',  ( -1.047445008332813989E-14, 0.000000000000000000, 1.000000000000000000 ) ) ;
#15891=CARTESIAN_POINT ( 'NONE',  ( 74.15067561874269586, 120.6499999999999915, -68.53801554307419508 ) ) ;
#15942=ORIENTED_EDGE ( 'NONE', *, *, #70178, .F. ) ;
#15944=LINE ( 'NONE', #62733, #48881 ) ;
#15976=CARTESIAN_POINT ( 'NONE',  ( -90.25311968877612401, 94.92443974548203300, 94.33669211993731096 ) ) ;
#15981=ORIENTED_EDGE ( 'NONE', *, *, #18249, .T. ) ;
#16019=PLANE ( 'NONE',  #9158 ) ;
#16053=DIRECTION ( 'NONE',  ( 0.000000000000000000, 1.000000000000000000, 0.000000000000000000 ) ) ;
#16099=AXIS2_PLACEMENT_3D ( 'NONE', #18493, #3532, #17616 ) ;
#16108=EDGE_LOOP ( 'NONE', ( #23608, #37814, #18155, #18883 ) ) ;
#16140=CARTESIAN_POINT ( 'NONE',  ( -130.2867309503044453, 73.00415124681445889, -8.386992461123011111 ) ) ;
#16141=ORIENTED_EDGE ( 'NONE', *, *, #23023, .T. ) ;
#16143=VECTOR ( 'NONE', #71893, 1000.000000000000000 ) ;
#16144=CIRCLE ( 'NONE', #5967, 5.041900000000001825 ) ;
#16147=ORIENTED_EDGE ( 'NONE', *, *, #69483, .T. ) ;
#16199=CARTESIAN_POINT ( 'NONE',  ( 84.37439091330263352, 89.26666702275852572, 99.62873342662707898 ) ) ;
#16212=CARTESIAN_POINT ( 'NONE',  ( 9.331435647859348646E-23, 95.25000000000000000, 130.5560000000000116 ) ) ;
#16216=DIRECTION ( 'NONE',  ( 0.000000000000000000, 0.000000000000000000, -1.000000000000000000 ) ) ;
#16238=DIRECTION ( 'NONE',  ( 0.000000000000000000, 1.000000000000000000, 0.000000000000000000 ) ) ;
#16265=CARTESIAN_POINT ( 'NONE',  ( 100.8961411191535973, 120.6499999999999915, 3.968750000000400124 ) ) ;
#16268=CARTESIAN_POINT ( 'NONE',  ( -3.174999999999664979, 124.5870000000000033, -31.75000000000000000 ) ) ;
#16293=AXIS2_PLACEMENT_3D ( 'NONE', #69858, #7186, #89867 ) ;
#16324=DIRECTION ( 'NONE',  ( 0.000000000000000000, 0.000000000000000000, 1.000000000000000000 ) ) ;
#16354=PLANE ( 'NONE',  #17956 ) ;
#16374=EDGE_CURVE ( 'NONE', #84699, #64009, #19241, .T. ) ;
#16392=CARTESIAN_POINT ( 'NONE',  ( 100.4448767513723624, 86.64186789594792515, -83.40142812120552662 ) ) ;
#16452=ORIENTED_EDGE ( 'NONE', *, *, #30625, .T. ) ;
#16453=VECTOR ( 'NONE', #82598, 1000.000000000000114 ) ;
#16463=EDGE_CURVE ( 'NONE', #80081, #57023, #78581, .T. ) ;
#16474=AXIS2_PLACEMENT_3D ( 'NONE', #30665, #44274, #44723 ) ;
#16503=CARTESIAN_POINT ( 'NONE',  ( 74.36911441044604487, 82.54999999999999716, 92.32962665258637003 ) ) ;
#16527=CARTESIAN_POINT ( 'NONE',  ( 100.8594679592200833, 82.54999999999999716, 82.89895571708400723 ) ) ;
#16533=VERTEX_POINT ( 'NONE', #37220 ) ;
#16548=EDGE_LOOP ( 'NONE', ( #2970, #46441, #85163, #86715, #18199, #74772 ) ) ;
#16559=CARTESIAN_POINT ( 'NONE',  ( 105.4788588808462038, 120.6499999999999915, -3.968749999999580336 ) ) ;
#16565=VERTEX_POINT ( 'NONE', #32173 ) ;
#16573=EDGE_CURVE ( 'NONE', #50785, #6249, #27827, .T. ) ;
#16606=DIRECTION ( 'NONE',  ( 0.000000000000000000, -1.000000000000000000, 0.000000000000000000 ) ) ;
#16616=ORIENTED_EDGE ( 'NONE', *, *, #69735, .F. ) ;
#16650=CIRCLE ( 'NONE', #26814, 5.041900000000000048 ) ;
#16668=EDGE_CURVE ( 'NONE', #57023, #65340, #83043, .T. ) ;
#16672=EDGE_CURVE ( 'NONE', #84699, #54126, #41658, .T. ) ;
#16717=VECTOR ( 'NONE', #23240, 1000.000000000000000 ) ;
#16766=EDGE_CURVE ( 'NONE', #82989, #76109, #22236, .T. ) ;
#16769=CARTESIAN_POINT ( 'NONE',  ( 0.000000000000000000, 127.0000000000000000, -103.1875000000000000 ) ) ;
#16770=CARTESIAN_POINT ( 'NONE',  ( -77.89700433585372252, 82.54999999999999716, 59.93649209371516662 ) ) ;
#16774=CARTESIAN_POINT ( 'NONE',  ( 68.91674821478504498, 82.54999999999999716, -68.91674821478385127 ) ) ;
#16781=AXIS2_PLACEMENT_3D ( 'NONE', #4640, #19170, #18262 ) ;
#16783=CARTESIAN_POINT ( 'NONE',  ( 103.1875000000000000, 127.0000000000000000, 3.602774393244745134E-13 ) ) ;
#16792=PLANE ( 'NONE',  #71172 ) ;
#16826=AXIS2_PLACEMENT_3D ( 'NONE', #41735, #29032, #28111 ) ;
#16830=LINE ( 'NONE', #44510, #75647 ) ;
#16856=VERTEX_POINT ( 'NONE', #32463 ) ;
#16862=CARTESIAN_POINT ( 'NONE',  ( -87.44839512528793080, 93.33885111288432768, 96.94208673523014852 ) ) ;
#16863=DIRECTION ( 'NONE',  ( -0.000000000000000000, 1.000000000000000000, 0.000000000000000000 ) ) ;
#16867=DIRECTION ( 'NONE',  ( 0.000000000000000000, 0.000000000000000000, 1.000000000000000000 ) ) ;
#16875=CARTESIAN_POINT ( 'NONE',  ( -74.36911441044730964, 82.54999999999999716, 92.32962665258534685 ) ) ;
#16888=AXIS2_PLACEMENT_3D ( 'NONE', #62210, #21792, #35390 ) ;
#16893=CYLINDRICAL_SURFACE ( 'NONE', #31196, 118.5560000000000116 ) ;
#16903=EDGE_LOOP ( 'NONE', ( #17615, #19858, #43502, #81109 ) ) ;
#16925=ORIENTED_EDGE ( 'NONE', *, *, #29847, .F. ) ;
#16944=DIRECTION ( 'NONE',  ( 0.000000000000000000, -1.000000000000000000, 0.000000000000000000 ) ) ;
#16946=VECTOR ( 'NONE', #66515, 1000.000000000000000 ) ;
#16950=ORIENTED_EDGE ( 'NONE', *, *, #30512, .F. ) ;
#16956=FACE_OUTER_BOUND ( 'NONE', #3189, .T. ) ;
#16961=LINE ( 'NONE', #78314, #79076 ) ;
#16970=CARTESIAN_POINT ( 'NONE',  ( 100.8961411191535973, 120.6499999999999915, 3.968750000000400124 ) ) ;
#16974=CARTESIAN_POINT ( 'NONE',  ( 118.5559323284754782, 69.85063172184841562, 0.8489616598202707198 ) ) ;
#16980=VERTEX_POINT ( 'NONE', #56029 ) ;
#16988=AXIS2_PLACEMENT_3D ( 'NONE', #53481, #18539, #31724 ) ;
#16998=CARTESIAN_POINT ( 'NONE',  ( -5.635505087355097587, 71.13841253056517644, 118.4244851085658468 ) ) ;
#17020=CARTESIAN_POINT ( 'NONE',  ( 72.96458098368701428, 117.4749999999999943, -72.96458098368670164 ) ) ;
#17024=CARTESIAN_POINT ( 'NONE',  ( -130.5246035444015718, 70.17666187254643262, -2.891673250712901044 ) ) ;
#17028=ORIENTED_EDGE ( 'NONE', *, *, #47415, .T. ) ;
#17033=EDGE_LOOP ( 'NONE', ( #77103, #1915 ) ) ;
#17043=PLANE ( 'NONE',  #16474 ) ;
#17059=ORIENTED_EDGE ( 'NONE', *, *, #80815, .F. ) ;
#17065=CARTESIAN_POINT ( 'NONE',  ( -4.087661814003488381, 94.58137602904392338, -130.4926000606902505 ) ) ;
#17068=CARTESIAN_POINT ( 'NONE',  ( 0.000000000000000000, 61.59999999999999432, 0.000000000000000000 ) ) ;
#17077=AXIS2_PLACEMENT_3D ( 'NONE', #87659, #46291, #6323 ) ;
#17137=CIRCLE ( 'NONE', #25881, 7.937500000000000000 ) ;
#17143=DIRECTION ( 'NONE',  ( 0.000000000000000000, 1.000000000000000000, 0.000000000000000000 ) ) ;
#17149=DIRECTION ( 'NONE',  ( 0.000000000000000000, 0.000000000000000000, 1.000000000000000000 ) ) ;
#17153=CARTESIAN_POINT ( 'NONE',  ( 1.451892259197136103E-14, 101.5999999999999943, -118.5560000000000116 ) ) ;
#17160=DIRECTION ( 'NONE',  ( 0.000000000000000000, 1.000000000000000000, 0.000000000000000000 ) ) ;
#17164=CARTESIAN_POINT ( 'NONE',  ( 82.89895571708156297, 82.54999999999999716, 100.8594679592221155 ) ) ;
#17167=CARTESIAN_POINT ( 'NONE',  ( 100.6522392491104938, 79.66749569656609253, -83.15048135366419046 ) ) ;
#17180=CARTESIAN_POINT ( 'NONE',  ( 79.20758933349287645, 71.53193882405246029, 88.21655330423307362 ) ) ;
#17185=ORIENTED_EDGE ( 'NONE', *, *, #89626, .F. ) ;
#17189=EDGE_CURVE ( 'NONE', #36762, #81558, #89393, .T. ) ;
#17204=DIRECTION ( 'NONE',  ( 0.000000000000000000, -1.000000000000000000, 0.000000000000000000 ) ) ;
#17205=B_SPLINE_CURVE_WITH_KNOTS ( 'NONE', 3,
 ( #66745, #4527, #81743, #46732, #74461, #68543, #47627, #11334, #18593, #73557, #47175, #53530, #39033, #68095, #74011, #11790, #81302, #12236, #39486, #39924, #67643, #40821, #75359, #33122, #19045, #67187, #59912, #19492, #53982, #4970, #32668, #60363, #53076, #25863, #54426, #5427, #74909, #88988, #6312, #32215, #40379, #5879, #34004, #88550, #33565, #26747, #82190, #61705, #24967 ),
 .UNSPECIFIED., .F., .F.,
 ( 4, 2, 2, 2, 2, 2, 2, 2, 2, 2, 2, 2, 2, 2, 2, 1, 2, 2, 2, 2, 2, 2, 2, 2, 4 ),
 ( 0.01986933033599076401, 0.02111088875730814801, 0.02235244717862553548, 0.02483556402126030349, 0.02607712244257766668, 0.02731868086389502986, 0.02980179770652975971, 0.03228491454916448955, 0.03352647297048184927, 0.03476803139179920898, 0.03725114823443394924, 0.03849270665575131589, 0.03973426507706868949, 0.04221738191970342974, 0.04345894034102079639, 0.04470049876233816999, 0.04594205718365554358, 0.04718361560497291718, 0.04966673244760767825, 0.05090829086892507960, 0.05214984929024249483, 0.05463296613287728365, 0.05587452455419468500, 0.05711608297551208635, 0.05959919981814688905 ),
 .UNSPECIFIED. ) ;
#17242=LINE ( 'NONE', #19018, #25910 ) ;
#17250=EDGE_CURVE ( 'NONE', #41991, #79223, #75759, .T. ) ;
#17268=CARTESIAN_POINT ( 'NONE',  ( 72.96458098368650269, 127.0000000000000000, 80.10833098368729566 ) ) ;
#17280=EDGE_LOOP ( 'NONE', ( #37562, #66032 ) ) ;
#17289=CARTESIAN_POINT ( 'NONE',  ( -103.1875000000000000, 101.5999999999999943, -1.080832317973422076E-12 ) ) ;
#17291=ORIENTED_EDGE ( 'NONE', *, *, #85400, .F. ) ;
#17299=FACE_OUTER_BOUND ( 'NONE', #49097, .T. ) ;
#17338=DIRECTION ( 'NONE',  ( -0.000000000000000000, 1.000000000000000000, -0.000000000000000000 ) ) ;
#17351=CARTESIAN_POINT ( 'NONE',  ( 31.75000000000000000, 104.3431970271542042, 3.174999999999999822 ) ) ;
#17357=CARTESIAN_POINT ( 'NONE',  ( -12.27300924177314911, 79.25817979229439914, 129.9779100289732696 ) ) ;
#17359=DIRECTION ( 'NONE',  ( 0.000000000000000000, 1.000000000000000000, 0.000000000000000000 ) ) ;
#17378=CARTESIAN_POINT ( 'NONE',  ( -103.1875000000000000, 127.0000000000000000, -1.080832317973422076E-12 ) ) ;
#17379=AXIS2_PLACEMENT_3D ( 'NONE', #53317, #34241, #55110 ) ;
#17397=DIRECTION ( 'NONE',  ( 0.000000000000000000, -1.000000000000000000, 0.000000000000000000 ) ) ;
#17409=ORIENTED_EDGE ( 'NONE', *, *, #5608, .T. ) ;
#17412=DIRECTION ( 'NONE',  ( 0.000000000000000000, -1.000000000000000000, 0.000000000000000000 ) ) ;
#17418=CARTESIAN_POINT ( 'NONE',  ( 117.9439354154377924, 78.46407912418312947, 12.03195559056957187 ) ) ;
#17428=DIRECTION ( 'NONE',  ( -0.4999999999999990563, 0.000000000000000000, -0.8660254037844392627 ) ) ;
#17449=EDGE_LOOP ( 'NONE', ( #71921, #3563, #15276, #18992 ) ) ;
#17476=EDGE_CURVE ( 'NONE', #44525, #88514, #33302, .T. ) ;
#17480=LINE ( 'NONE', #11099, #68492 ) ;
#17504=ADVANCED_FACE ( 'NONE', ( #7830 ), #56413, .F. ) ;
#17512=CARTESIAN_POINT ( 'NONE',  ( -7.205548786489490269E-13, 117.4749999999999943, 103.1875000000000000 ) ) ;
#17532=CARTESIAN_POINT ( 'NONE',  ( 79.21650378603776232, 93.55239623846831876, 88.20661029664658770 ) ) ;
#17538=CARTESIAN_POINT ( 'NONE',  ( 4.087661814003508809, 94.58137602904389496, 130.4926000606901937 ) ) ;
#17540=EDGE_CURVE ( 'NONE', #11232, #41269, #16144, .T. ) ;
#17541=CARTESIAN_POINT ( 'NONE',  ( 0.000000000000000000, 125.4759999999999991, 0.000000000000000000 ) ) ;
#17575=EDGE_LOOP ( 'NONE', ( #24474, #55854, #89084, #38228 ) ) ;
#17576=ORIENTED_EDGE ( 'NONE', *, *, #10799, .F. ) ;
#17588=DIRECTION ( 'NONE',  ( 0.8660254037844392627, 0.000000000000000000, 0.4999999999999990563 ) ) ;
#17590=PLANE ( 'NONE',  #68370 ) ;
#17615=ORIENTED_EDGE ( 'NONE', *, *, #40574, .F. ) ;
#17616=DIRECTION ( 'NONE',  ( 0.000000000000000000, 0.000000000000000000, -1.000000000000000000 ) ) ;
#17622=CARTESIAN_POINT ( 'NONE',  ( 90.81844170390269255, 75.15251084995274766, 76.20754074253750332 ) ) ;
#17634=CARTESIAN_POINT ( 'NONE',  ( 117.9583070260533901, 87.03046781249440755, -11.89069406032356824 ) ) ;
#17645=LINE ( 'NONE', #24463, #31949 ) ;
#17731=CARTESIAN_POINT ( 'NONE',  ( 0.000000000000000000, 61.59999999999999432, 130.5560000000000116 ) ) ;
#17741=DIRECTION ( 'NONE',  ( 0.000000000000000000, -1.000000000000000000, 0.000000000000000000 ) ) ;
#17751=CARTESIAN_POINT ( 'NONE',  ( -98.83759631548484492, 90.93932679091001603, 85.30153658290403484 ) ) ;
#17784=EDGE_LOOP ( 'NONE', ( #25929, #58481, #51569, #80238, #15178, #88658 ) ) ;
#17790=DIRECTION ( 'NONE',  ( -0.7071067811865490160, 0.000000000000000000, 0.7071067811865461294 ) ) ;
#17809=EDGE_LOOP ( 'NONE', ( #25507, #53310, #62024, #63467 ) ) ;
#17841=CARTESIAN_POINT ( 'NONE',  ( 82.89895571708365196, 82.54999999999999716, -100.8594679592203818 ) ) ;
#17858=AXIS2_PLACEMENT_3D ( 'NONE', #60612, #88355, #19742 ) ;
#17898=CARTESIAN_POINT ( 'NONE',  ( 72.96458098368650269, 127.0000000000000000, 72.96458098368729850 ) ) ;
#17921=ADVANCED_FACE ( 'NONE', ( #75878 ), #33643, .F. ) ;
#17956=AXIS2_PLACEMENT_3D ( 'NONE', #55862, #71328, #84524 ) ;
#17958=CARTESIAN_POINT ( 'NONE',  ( 12.27300924177314911, 79.25817979229439914, -129.9779100289732696 ) ) ;
#17966=CARTESIAN_POINT ( 'NONE',  ( 12.03249045273852502, 86.63451674300237926, 130.0003965276981432 ) ) ;
#17981=FACE_OUTER_BOUND ( 'NONE', #58106, .T. ) ;
#17984=EDGE_CURVE ( 'NONE', #62096, #9843, #27724, .T. ) ;
#17991=ORIENTED_EDGE ( 'NONE', *, *, #1946, .F. ) ;
#18002=CYLINDRICAL_SURFACE ( 'NONE', #71232, 5.041900000000001825 ) ;
#18006=EDGE_LOOP ( 'NONE', ( #56020, #64269, #29766, #45568 ) ) ;
#18009=ORIENTED_EDGE ( 'NONE', *, *, #72361, .T. ) ;
#18020=DIRECTION ( 'NONE',  ( 0.000000000000000000, 1.000000000000000000, 0.000000000000000000 ) ) ;
#18024=ORIENTED_EDGE ( 'NONE', *, *, #41562, .T. ) ;
#18031=DIRECTION ( 'NONE',  ( 0.000000000000000000, -1.000000000000000000, 0.000000000000000000 ) ) ;
#18046=CIRCLE ( 'NONE', #29655, 5.041900000000001825 ) ;
#18048=ORIENTED_EDGE ( 'NONE', *, *, #20287, .T. ) ;
#18065=CARTESIAN_POINT ( 'NONE',  ( 118.1052286201201724, 89.94786999841838337, -10.33119577496741925 ) ) ;
#18071=LINE ( 'NONE', #80326, #59689 ) ;
#18100=CARTESIAN_POINT ( 'NONE',  ( -118.5472164932298256, 69.93120980984942037, 1.660430599529278295 ) ) ;
#18108=ORIENTED_EDGE ( 'NONE', *, *, #32821, .F. ) ;
#18120=CARTESIAN_POINT ( 'NONE',  ( 6.174546696621020337E-16, 101.5999999999999943, -108.2293999999999983 ) ) ;
#18128=CARTESIAN_POINT ( 'NONE',  ( 0.000000000000000000, 95.25000000000000000, 0.000000000000000000 ) ) ;
#18137=DIRECTION ( 'NONE',  ( 0.000000000000000000, 0.000000000000000000, -1.000000000000000000 ) ) ;
#18138=VERTEX_POINT ( 'NONE', #15458 ) ;
#18151=AXIS2_PLACEMENT_3D ( 'NONE', #87530, #25739, #24414 ) ;
#18155=ORIENTED_EDGE ( 'NONE', *, *, #37979, .T. ) ;
#18181=EDGE_LOOP ( 'NONE', ( #86446, #60153 ) ) ;
#18193=CYLINDRICAL_SURFACE ( 'NONE', #49319, 88.90000000000000568 ) ;
#18199=ORIENTED_EDGE ( 'NONE', *, *, #83252, .F. ) ;
#18236=CARTESIAN_POINT ( 'NONE',  ( 3.175000000000334666, 124.5870000000000033, -31.75000000000000000 ) ) ;
#18237=PLANE ( 'NONE',  #50102 ) ;
#18241=ORIENTED_EDGE ( 'NONE', *, *, #34718, .T. ) ;
#18249=EDGE_CURVE ( 'NONE', #61102, #83340, #21254, .T. ) ;
#18257=CARTESIAN_POINT ( 'NONE',  ( -69.72411017813060141, 120.6499999999999915, 69.72411017812929401 ) ) ;
#18258=PLANE ( 'NONE',  #88801 ) ;
#18262=DIRECTION ( 'NONE',  ( 0.000000000000000000, 0.000000000000000000, 1.000000000000000000 ) ) ;
#18272=FACE_OUTER_BOUND ( 'NONE', #58014, .T. ) ;
#18286=VERTEX_POINT ( 'NONE', #33532 ) ;
#18294=AXIS2_PLACEMENT_3D ( 'NONE', #62319, #43208, #20556 ) ;
#18298=CARTESIAN_POINT ( 'NONE',  ( 118.3867465934798560, 71.53193882405243187, 6.370299515175424254 ) ) ;
#18310=CARTESIAN_POINT ( 'NONE',  ( 5.041899999999280624, 117.4749999999999943, 103.1875000000000000 ) ) ;
#18332=CARTESIAN_POINT ( 'NONE',  ( 1.598849875094818280E-14, 61.59999999999999432, -130.5560000000000116 ) ) ;
#18341=LINE ( 'NONE', #4279, #62336 ) ;
#18367=CARTESIAN_POINT ( 'NONE',  ( -0.8293608286808433760, 95.25000000000002842, -118.5560000000000400 ) ) ;
#18378=CARTESIAN_POINT ( 'NONE',  ( 103.1875000000000000, 117.4749999999999943, -7.937499999999639400 ) ) ;
#18381=EDGE_CURVE ( 'NONE', #35298, #73407, #39451, .T. ) ;
#18391=CARTESIAN_POINT ( 'NONE',  ( -74.70173812346030218, 79.26437155269049128, 92.06079644778199622 ) ) ;
#18401=LINE ( 'NONE', #57958, #82816 ) ;
#18405=CARTESIAN_POINT ( 'NONE',  ( 86.13037352894073706, 94.82191660594808980, 81.46927207886326983 ) ) ;
#18408=EDGE_LOOP ( 'NONE', ( #3469, #61408, #43326, #25107 ) ) ;
#18416=DIRECTION ( 'NONE',  ( 0.000000000000000000, 0.000000000000000000, 1.000000000000000000 ) ) ;
#18450=CARTESIAN_POINT ( 'NONE',  ( 129.9449656991351105, 80.88456863959032717, -12.61750076990764313 ) ) ;
#18463=LINE ( 'NONE', #87968, #55052 ) ;
#18493=CARTESIAN_POINT ( 'NONE',  ( -72.96458098368751166, 117.4749999999999943, 72.96458098368620426 ) ) ;
#18503=AXIS2_PLACEMENT_3D ( 'NONE', #43924, #366, #28062 ) ;
#18509=FACE_OUTER_BOUND ( 'NONE', #7337, .T. ) ;
#18539=DIRECTION ( 'NONE',  ( 0.000000000000000000, 1.000000000000000000, 0.000000000000000000 ) ) ;
#18551=ORIENTED_EDGE ( 'NONE', *, *, #80815, .T. ) ;
#18593=CARTESIAN_POINT ( 'NONE',  ( -130.0580535164678508, 88.17609398443093482, -11.39345613590910666 ) ) ;
#18605=EDGE_LOOP ( 'NONE', ( #21370, #89509, #4564, #14187 ) ) ;
#18607=ORIENTED_EDGE ( 'NONE', *, *, #22118, .T. ) ;
#18609=CARTESIAN_POINT ( 'NONE',  ( 82.89895571708365196, 83.38918798244688446, -100.8594679592203676 ) ) ;
#18613=EDGE_CURVE ( 'NONE', #13215, #63081, #58877, .T. ) ;
#18615=CARTESIAN_POINT ( 'NONE',  ( -3.306873253463332496, 70.28105300984509540, -118.5105382607468130 ) ) ;
#18629=FACE_OUTER_BOUND ( 'NONE', #40672, .T. ) ;
#18640=CARTESIAN_POINT ( 'NONE',  ( -117.9423201497065321, 86.64222086580515736, -12.05142355921143960 ) ) ;
#18655=DIRECTION ( 'NONE',  ( 0.000000000000000000, 1.000000000000000000, 0.000000000000000000 ) ) ;
#18708=ADVANCED_FACE ( 'NONE', ( #74323 ), #88406, .F. ) ;
#18725=DIRECTION ( 'NONE',  ( -0.000000000000000000, 1.000000000000000000, 0.000000000000000000 ) ) ;
#18734=CARTESIAN_POINT ( 'NONE',  ( 78.00648098368699834, 117.4749999999999943, -72.96458098368670164 ) ) ;
#18759=CARTESIAN_POINT ( 'NONE',  ( -100.3415888741737376, 78.07027470200928576, -83.52520760052931337 ) ) ;
#18766=DIRECTION ( 'NONE',  ( 0.000000000000000000, 0.000000000000000000, -1.000000000000000000 ) ) ;
#18788=DIRECTION ( 'NONE',  ( 1.000000000000000000, 0.000000000000000000, 0.000000000000000000 ) ) ;
#18789=ORIENTED_EDGE ( 'NONE', *, *, #44854, .F. ) ;
#18818=DIRECTION ( 'NONE',  ( 0.000000000000000000, 1.000000000000000000, 0.000000000000000000 ) ) ;
#18831=CARTESIAN_POINT ( 'NONE',  ( 3.174999999999879918, 111.1250000000000000, 33.98325472291465132 ) ) ;
#18845=CARTESIAN_POINT ( 'NONE',  ( -77.39114642430010349, 127.0000000000000000, 71.77848634863050847 ) ) ;
#18862=CARTESIAN_POINT ( 'NONE',  ( 6.364581335559162056, 71.52860519235655090, -130.4026037055029690 ) ) ;
#18865=CARTESIAN_POINT ( 'NONE',  ( 91.26325766987402233, 88.91291927174620469, 75.67533895324436344 ) ) ;
#18872=CARTESIAN_POINT ( 'NONE',  ( -85.30153658290372221, 90.93932679091004445, -98.83759631548520019 ) ) ;
#18883=ORIENTED_EDGE ( 'NONE', *, *, #32975, .T. ) ;
#18967=LINE ( 'NONE', #13501, #12753 ) ;
#18970=CARTESIAN_POINT ( 'NONE',  ( 118.4577320646419594, 94.30044247306076954, -4.871303722668521630 ) ) ;
#18975=ORIENTED_EDGE ( 'NONE', *, *, #34612, .T. ) ;
#18977=VECTOR ( 'NONE', #65349, 1000.000000000000000 ) ;
#18992=ORIENTED_EDGE ( 'NONE', *, *, #12894, .T. ) ;
#19005=CARTESIAN_POINT ( 'NONE',  ( -117.8827794761417493, 80.88465057165902294, 12.61751953376163549 ) ) ;
#19018=CARTESIAN_POINT ( 'NONE',  ( -7.941868552260229762E-13, 120.6499999999999915, 107.7702177616926065 ) ) ;
#19043=UNCERTAINTY_MEASURE_WITH_UNIT (LENGTH_MEASURE( 1.000000000000000082E-05 ), #73666, 'distance_accuracy_value', 'NONE');
#19045=CARTESIAN_POINT ( 'NONE',  ( -130.5560151749589295, 95.25015599858942039, -0.4097429349699925338 ) ) ;
#19059=CARTESIAN_POINT ( 'NONE',  ( 91.72735010416676005, 95.24968527363472504, -92.90667244829690219 ) ) ;
#19083=CARTESIAN_POINT ( 'NONE',  ( -118.0645351272586936, 89.26692529358285810, -10.78628659036711035 ) ) ;
#19096=CARTESIAN_POINT ( 'NONE',  ( 31.75000000000000000, 111.1250000000000000, -3.174999999999999822 ) ) ;
#19104=CARTESIAN_POINT ( 'NONE',  ( 89.55214429302422730, 92.12496802699136822, -77.69357874334680503 ) ) ;
#19109=EDGE_CURVE ( 'NONE', #4210, #89451, #72799, .T. ) ;
#19125=CARTESIAN_POINT ( 'NONE',  ( 130.2877996231769941, 92.12504059357186748, 8.385216644675763220 ) ) ;
#19142=CIRCLE ( 'NONE', #69918, 130.5560000000000116 ) ;
#19166=EDGE_CURVE ( 'NONE', #4210, #3366, #70429, .T. ) ;
#19170=DIRECTION ( 'NONE',  ( 0.000000000000000000, -1.000000000000000000, 0.000000000000000000 ) ) ;
#19204=AXIS2_PLACEMENT_3D ( 'NONE', #59354, #87083, #46158 ) ;
#19206=DIRECTION ( 'NONE',  ( 0.000000000000000000, 0.000000000000000000, 1.000000000000000000 ) ) ;
#19213=CARTESIAN_POINT ( 'NONE',  ( -85.96437953530681852, 73.28356282573680858, -98.26026929335846205 ) ) ;
#19216=DIRECTION ( 'NONE',  ( 0.000000000000000000, 0.000000000000000000, 1.000000000000000000 ) ) ;
#19225=EDGE_CURVE ( 'NONE', #50035, #22899, #8608, .T. ) ;
#19241=CIRCLE ( 'NONE', #61305, 5.041900000000001825 ) ;
#19265=DIRECTION ( 'NONE',  ( 0.000000000000000000, 0.000000000000000000, 1.000000000000000000 ) ) ;
#19267=LINE ( 'NONE', #6976, #35476 ) ;
#19270=CARTESIAN_POINT ( 'NONE',  ( 129.9368274816652331, 82.54999999999999716, -12.69999999999864038 ) ) ;
#19279=EDGE_LOOP ( 'NONE', ( #7297, #1817, #13644, #7665 ) ) ;
#19305=ORIENTED_EDGE ( 'NONE', *, *, #52274, .T. ) ;
#19313=CARTESIAN_POINT ( 'NONE',  ( 11.39831192919941927, 76.93384533283848725, -130.0576265831481635 ) ) ;
#19316=CARTESIAN_POINT ( 'NONE',  ( -103.1875000000000000, 117.4749999999999943, 7.937499999998919087 ) ) ;
#19321=DIRECTION ( 'NONE',  ( 1.000000000000000000, 0.000000000000000000, 0.000000000000000000 ) ) ;
#19337=VERTEX_POINT ( 'NONE', #9102 ) ;
#19361=CARTESIAN_POINT ( 'NONE',  ( 130.1663562161751884, 74.81660785136577374, -10.08264331121358381 ) ) ;
#19418=CARTESIAN_POINT ( 'NONE',  ( 118.4860461769942361, 94.58006533271583294, -4.091503224719446941 ) ) ;
#19492=CARTESIAN_POINT ( 'NONE',  ( -130.5247076678899134, 94.92443974548204721, 2.887521757540267409 ) ) ;
#19496=VERTEX_POINT ( 'NONE', #53510 ) ;
#19502=CARTESIAN_POINT ( 'NONE',  ( 1.451892259197136103E-14, 61.59999999999999432, -118.5560000000000116 ) ) ;
#19503=CARTESIAN_POINT ( 'NONE',  ( 96.94152442043744600, 93.33921197991993779, -87.44900557253130557 ) ) ;
#19508=CARTESIAN_POINT ( 'NONE',  ( -6.360060842339565923, 71.54945291875249325, -118.3858484385471286 ) ) ;
#19513=AXIS2_PLACEMENT_3D ( 'NONE', #66738, #87197, #18137 ) ;
#19520=CARTESIAN_POINT ( 'NONE',  ( 98.60478223830740774, 120.6499999999999915, 3.859079674607175002E-13 ) ) ;
#19521=DIRECTION ( 'NONE',  ( 0.000000000000000000, 1.000000000000000000, 0.000000000000000000 ) ) ;
#19529=CARTESIAN_POINT ( 'NONE',  ( -7.940696711283829426E-13, 127.0000000000000000, 107.7702177616926065 ) ) ;
#19531=PLANE ( 'NONE',  #75184 ) ;
#19555=VECTOR ( 'NONE', #77927, 999.9999999999998863 ) ;
#19568=CARTESIAN_POINT ( 'NONE',  ( 130.1658227983197662, 90.29814575435203494, 10.09656535537147803 ) ) ;
#19569=FACE_OUTER_BOUND ( 'NONE', #5390, .T. ) ;
#19572=MECHANICAL_DESIGN_GEOMETRIC_PRESENTATION_REPRESENTATION('',(#25336),#29699);
#19575=ORIENTED_EDGE ( 'NONE', *, *, #81409, .T. ) ;
#19578=CARTESIAN_POINT ( 'NONE',  ( -11.41387019979801387, 76.91918732108555901, -130.0565070412864372 ) ) ;
#19585=CARTESIAN_POINT ( 'NONE',  ( -91.81719692706842295, 78.06989712577870932, -75.00102098090771108 ) ) ;
#19589=B_SPLINE_CURVE_WITH_KNOTS ( 'NONE', 3,
 ( #86582, #52891, #3457, #9833, #3898, #17538, #37539, #59738, #58410, #65238, #3012, #72932, #31595, #10704, #67016, #24353, #46101, #73832, #80220, #17966, #45215, #38411, #59297, #30714, #45650 ),
 .UNSPECIFIED., .F., .F.,
 ( 4, 2, 2, 1, 2, 2, 2, 2, 2, 2, 2, 2, 4 ),
 ( 0.03972946622853323895, 0.04221318292723492960, 0.04345504127658578186, 0.04469689962593662719, 0.04593875797528747251, 0.04718061632463831784, 0.04966433302334004318, 0.05090619137269088851, 0.05214804972204173383, 0.05463176642074343836, 0.05587362477009429063, 0.05711548311944514289, 0.05959919981814688211 ),
 .UNSPECIFIED. ) ;
#19594=AXIS2_PLACEMENT_3D ( 'NONE', #53221, #19632, #87783 ) ;
#19597=AXIS2_PLACEMENT_3D ( 'NONE', #6773, #41722, #63531 ) ;
#19632=DIRECTION ( 'NONE',  ( -0.000000000000000000, 1.000000000000000000, -0.000000000000000000 ) ) ;
#19635=ORIENTED_EDGE ( 'NONE', *, *, #37807, .T. ) ;
#19645=DIRECTION ( 'NONE',  ( -0.000000000000000000, -1.000000000000000000, -0.000000000000000000 ) ) ;
#19653=CARTESIAN_POINT ( 'NONE',  ( -98.06260288352387988, 72.98383416765814502, -86.19129576945131532 ) ) ;
#19656=DIRECTION ( 'NONE',  ( 0.000000000000000000, 0.000000000000000000, 1.000000000000000000 ) ) ;
#19701=DIRECTION ( 'NONE',  ( 0.000000000000000000, 1.000000000000000000, 0.000000000000000000 ) ) ;
#19712=DIRECTION ( 'NONE',  ( 1.000000000000000000, 0.000000000000000000, 6.982966722218760189E-15 ) ) ;
#19722=B_SPLINE_CURVE_WITH_KNOTS ( 'NONE', 3,
 ( #68731, #82827, #27833, #54617, #6070, #61448, #6949, #61012, #34650, #76890, #54169, #42341, #47813, #68290, #55512, #48705, #6497, #21482, #82377, #70072, #81929, #75553, #69628, #49157, #34197 ),
 .UNSPECIFIED., .F., .F.,
 ( 4, 2, 2, 1, 2, 2, 2, 2, 2, 2, 2, 2, 4 ),
 ( 0.03973448063954120035, 0.04221847903031247795, 0.04346047822569811675, 0.04470247742108374861, 0.04594447661646938741, 0.04718647581185502621, 0.04967047420262627605, 0.05091247339801188709, 0.05215447259339749814, 0.05463847098416872022, 0.05588047017955435208, 0.05712246937493997700, 0.05960646776571127542 ),
 .UNSPECIFIED. ) ;
#19725=DIRECTION ( 'NONE',  ( 0.7071067811865536790, 0.000000000000000000, -0.7071067811865414665 ) ) ;
#19729=AXIS2_PLACEMENT_3D ( 'NONE', #49898, #1326, #871 ) ;
#19742=DIRECTION ( 'NONE',  ( 0.000000000000000000, 0.000000000000000000, 1.000000000000000000 ) ) ;
#19758=CIRCLE ( 'NONE', #58892, 7.143750000000001599 ) ;
#19761=DIRECTION ( 'NONE',  ( 0.000000000000000000, 0.000000000000000000, -1.000000000000000000 ) ) ;
#19763=CARTESIAN_POINT ( 'NONE',  ( 90.13147184857858463, 91.23868085022587593, 77.01901799881319732 ) ) ;
#19808=DIRECTION ( 'NONE',  ( 0.000000000000000000, -1.000000000000000000, 0.000000000000000000 ) ) ;
#19812=VECTOR ( 'NONE', #26056, 1000.000000000000000 ) ;
#19831=VERTEX_POINT ( 'NONE', #84856 ) ;
#19845=ADVANCED_FACE ( 'NONE', ( #22624 ), #36696, .F. ) ;
#19849=CARTESIAN_POINT ( 'NONE',  ( 5.210259806972410633E-15, 111.1250000000000000, -42.54500000000000171 ) ) ;
#19858=ORIENTED_EDGE ( 'NONE', *, *, #43562, .T. ) ;
#19870=DIRECTION ( 'NONE',  ( 0.7071067811865533459, 0.000000000000000000, -0.7071067811865416886 ) ) ;
#19899=CARTESIAN_POINT ( 'NONE',  ( -118.1704280561597358, 74.16215221268205937, -9.571784452933755460 ) ) ;
#19922=DIRECTION ( 'NONE',  ( 0.000000000000000000, 0.000000000000000000, 1.000000000000000000 ) ) ;
#19950=ORIENTED_EDGE ( 'NONE', *, *, #16672, .T. ) ;
#19954=ORIENTED_EDGE ( 'NONE', *, *, #41078, .F. ) ;
#19955=EDGE_CURVE ( 'NONE', #16565, #83000, #18463, .T. ) ;
#19958=ORIENTED_EDGE ( 'NONE', *, *, #46799, .T. ) ;
#19959=FACE_OUTER_BOUND ( 'NONE', #50813, .T. ) ;
#19960=CARTESIAN_POINT ( 'NONE',  ( 86.19179098795335392, 92.11674985319540099, -98.06216817836228472 ) ) ;
#19989=CARTESIAN_POINT ( 'NONE',  ( -118.4407179355509356, 94.12556101775334128, -5.241146580996161930 ) ) ;
#19993=DIRECTION ( 'NONE',  ( -0.000000000000000000, -0.000000000000000000, 1.000000000000000000 ) ) ;
#19995=CARTESIAN_POINT ( 'NONE',  ( 0.000000000000000000, 101.5999999999999943, 0.000000000000000000 ) ) ;
#20023=DIRECTION ( 'NONE',  ( 3.491483361109380094E-15, 0.000000000000000000, -1.000000000000000000 ) ) ;
#20028=CARTESIAN_POINT ( 'NONE',  ( 130.3837601098275059, 93.33885111288434189, -6.713053715882820960 ) ) ;
#20039=CARTESIAN_POINT ( 'NONE',  ( -4.879617406430184268, 70.80304812169737261, -130.4664555583633501 ) ) ;
#20046=CARTESIAN_POINT ( 'NONE',  ( -84.41866557162670404, 69.84937538953985836, -83.24493215373384203 ) ) ;
#20098=ORIENTED_EDGE ( 'NONE', *, *, #64665, .F. ) ;
#20105=CARTESIAN_POINT ( 'NONE',  ( 0.000000000000000000, 101.5999999999999943, 0.000000000000000000 ) ) ;
#20112=VECTOR ( 'NONE', #17588, 999.9999999999998863 ) ;
#20151=DIRECTION ( 'NONE',  ( 0.000000000000000000, 0.000000000000000000, 1.000000000000000000 ) ) ;
#20160=VERTEX_POINT ( 'NONE', #7088 ) ;
#20171=CARTESIAN_POINT ( 'NONE',  ( 11.00058663074870324, 88.91008943578141555, -118.0447001808843766 ) ) ;
#20188=FACE_OUTER_BOUND ( 'NONE', #75179, .T. ) ;
#20189=VECTOR ( 'NONE', #69812, 1000.000000000000227 ) ;
#20204=CARTESIAN_POINT ( 'NONE',  ( -86.94609723791337785, 70.66242608954387094, 80.59807192910960794 ) ) ;
#20210=EDGE_LOOP ( 'NONE', ( #6499, #58419, #3758, #47021 ) ) ;
#20218=CARTESIAN_POINT ( 'NONE',  ( 85.84941893669208923, 94.92435932957491218, 81.76533775135520443 ) ) ;
#20225=CARTESIAN_POINT ( 'NONE',  ( -93.48397507443814902, 95.16896684734908263, -91.13883569058478429 ) ) ;
#20228=VECTOR ( 'NONE', #68808, 1000.000000000000000 ) ;
#20240=ORIENTED_EDGE ( 'NONE', *, *, #50407, .T. ) ;
#20249=ORIENTED_EDGE ( 'NONE', *, *, #4650, .F. ) ;
#20254=EDGE_CURVE ( 'NONE', #63483, #21337, #89770, .T. ) ;
#20287=EDGE_CURVE ( 'NONE', #79701, #47173, #27589, .T. ) ;
#20288=DIRECTION ( 'NONE',  ( 0.000000000000000000, 0.000000000000000000, 1.000000000000000000 ) ) ;
#20294=DIRECTION ( 'NONE',  ( 0.000000000000000000, 1.000000000000000000, 0.000000000000000000 ) ) ;
#20310=FACE_OUTER_BOUND ( 'NONE', #22832, .T. ) ;
#20325=PLANE ( 'NONE',  #12929 ) ;
#20339=CYLINDRICAL_SURFACE ( 'NONE', #15131, 7.937500000000000000 ) ;
#20354=CARTESIAN_POINT ( 'NONE',  ( -72.96458098368600531, 127.0000000000000000, -78.00648098368779415 ) ) ;
#20356=ORIENTED_EDGE ( 'NONE', *, *, #77000, .T. ) ;
#20375=AXIS2_PLACEMENT_3D ( 'NONE', #1856, #78172, #84082 ) ;
#20401=FACE_OUTER_BOUND ( 'NONE', #52084, .T. ) ;
#20402=CARTESIAN_POINT ( 'NONE',  ( 89.37861919290365620, 70.52006616879377532, 95.16559702356724415 ) ) ;
#20411=CARTESIAN_POINT ( 'NONE',  ( -78.57724105935571401, 120.6499999999999915, 67.35192090801800191 ) ) ;
#20412=CARTESIAN_POINT ( 'NONE',  ( 93.48344774443344818, 95.14808745951977187, -91.13664476550651727 ) ) ;
#20416=FACE_OUTER_BOUND ( 'NONE', #1245, .T. ) ;
#20420=EDGE_LOOP ( 'NONE', ( #7496, #73416, #27926, #55671 ) ) ;
#20425=DIRECTION ( 'NONE',  ( -0.4999999999999998890, 0.000000000000000000, -0.8660254037844387076 ) ) ;
#20436=LINE ( 'NONE', #59177, #7524 ) ;
#20457=B_SPLINE_CURVE_WITH_KNOTS ( 'NONE', 3,
 ( #37535, #57962, #3009, #71615, #45644, #38851, #73375, #58405, #72501, #85698, #37088, #9380, #65666, #86578, #52017, #64788, #17532, #11146, #23473, #32477, #67907, #53350, #12957, #33833, #12055, #54242, #68363, #20218, #18405, #33385, #87465, #82008, #5695, #39305, #81120, #81566, #19763, #89260, #59732, #88372, #18865, #61088, #47442, #52886, #25224, #75175, #11613, #80659, #6144 ),
 .UNSPECIFIED., .F., .F.,
 ( 4, 2, 2, 2, 2, 2, 2, 2, 2, 2, 2, 2, 2, 2, 2, 1, 2, 2, 2, 2, 2, 2, 2, 2, 4 ),
 ( 0.01987186023414423339, 0.02111356671950569489, 0.02235527320486715638, 0.02483868617559007591, 0.02608039266095154782, 0.02732209914631301972, 0.02980551211703596354, 0.03228892508775890735, 0.03353063157312035497, 0.03477233805848180259, 0.03725575102920469783, 0.03849745751456616627, 0.03973916399992762083, 0.04222257697065059934, 0.04346428345601208165, 0.04470598994137357785, 0.04594769642673506016, 0.04718940291209654941, 0.04967281588281953486, 0.05091452236818098942, 0.05215622885354243010, 0.05463964182426538085, 0.05588134830962686317, 0.05712305479498833161, 0.05960646776571133787 ),
 .UNSPECIFIED. ) ;
#20473=DIRECTION ( 'NONE',  ( -0.000000000000000000, 1.000000000000000000, 0.000000000000000000 ) ) ;
#20481=CARTESIAN_POINT ( 'NONE',  ( 130.1664033068597064, 90.28418055714726620, -10.08203418473755164 ) ) ;
#20485=ORIENTED_EDGE ( 'NONE', *, *, #58303, .F. ) ;
#20490=ORIENTED_EDGE ( 'NONE', *, *, #30631, .T. ) ;
#20503=CARTESIAN_POINT ( 'NONE',  ( -75.38287938185001735, 76.93600387762164416, -91.50401754987797176 ) ) ;
#20512=DIRECTION ( 'NONE',  ( 1.000000000000000000, 0.000000000000000000, 0.000000000000000000 ) ) ;
#20517=CARTESIAN_POINT ( 'NONE',  ( 97.40459591070923295, 72.22361908171431821, -86.93292302958576556 ) ) ;
#20524=CARTESIAN_POINT ( 'NONE',  ( 8.398302923777746898, 72.98741371662136146, 118.2596197875572415 ) ) ;
#20530=CARTESIAN_POINT ( 'NONE',  ( -31.75000000000000000, 111.1250000000000000, -3.175000000000219647 ) ) ;
#20539=DIRECTION ( 'NONE',  ( 0.7071067811865490160, 0.000000000000000000, 0.7071067811865461294 ) ) ;
#20554=DIRECTION ( 'NONE',  ( 0.000000000000000000, 0.000000000000000000, 1.000000000000000000 ) ) ;
#20556=DIRECTION ( 'NONE',  ( 0.000000000000000000, 0.000000000000000000, 1.000000000000000000 ) ) ;
#20588=ORIENTED_EDGE ( 'NONE', *, *, #14255, .F. ) ;
#20593=EDGE_CURVE ( 'NONE', #81558, #83603, #76012, .T. ) ;
#20637=LINE ( 'NONE', #48303, #89704 ) ;
#20646=CARTESIAN_POINT ( 'NONE',  ( -68.53801554307339927, 127.0000000000000000, -74.15067561874339219 ) ) ;
#20648=FACE_OUTER_BOUND ( 'NONE', #11817, .T. ) ;
#20707=CARTESIAN_POINT ( 'NONE',  ( 130.5246035444014581, 70.17666187254641841, 2.891673250713812759 ) ) ;
#20726=LINE ( 'NONE', #76129, #72404 ) ;
#20743=ORIENTED_EDGE ( 'NONE', *, *, #56491, .F. ) ;
#20753=ORIENTED_EDGE ( 'NONE', *, *, #84722, .T. ) ;
#20764=CARTESIAN_POINT ( 'NONE',  ( 0.000000000000000000, 101.5999999999999943, 0.000000000000000000 ) ) ;
#20791=DIRECTION ( 'NONE',  ( 0.000000000000000000, 1.000000000000000000, 0.000000000000000000 ) ) ;
#20794=ORIENTED_EDGE ( 'NONE', *, *, #1327, .F. ) ;
#20804=CARTESIAN_POINT ( 'NONE',  ( 9.568977433314790559, 74.15890990428199814, -118.1706578929490377 ) ) ;
#20813=VERTEX_POINT ( 'NONE', #29958 ) ;
#20818=FACE_OUTER_BOUND ( 'NONE', #37628, .T. ) ;
#20825=DIRECTION ( 'NONE',  ( 0.000000000000000000, 1.000000000000000000, 0.000000000000000000 ) ) ;
#20828=EDGE_LOOP ( 'NONE', ( #82522, #34178, #62990, #21024 ) ) ;
#20832=EDGE_LOOP ( 'NONE', ( #19575, #27056, #48449, #8046 ) ) ;
#20882=CIRCLE ( 'NONE', #36836, 5.041900000000001825 ) ;
#20885=CARTESIAN_POINT ( 'NONE',  ( 78.94931995840801164, 71.76236341257997253, -88.44575049335516326 ) ) ;
#20902=CARTESIAN_POINT ( 'NONE',  ( 75.00112839233754869, 87.03046781249436492, -91.81710919847664343 ) ) ;
#20914=DIRECTION ( 'NONE',  ( 0.000000000000000000, 1.000000000000000000, 0.000000000000000000 ) ) ;
#20925=DIRECTION ( 'NONE',  ( 0.7071067811865389130, 0.000000000000000000, 0.7071067811865561215 ) ) ;
#20958=ORIENTED_EDGE ( 'NONE', *, *, #39616, .T. ) ;
#20967=AXIS2_PLACEMENT_3D ( 'NONE', #59679, #86084, #72005 ) ;
#20982=DIRECTION ( 'NONE',  ( 0.000000000000000000, -1.000000000000000000, 0.000000000000000000 ) ) ;
#20984=FACE_OUTER_BOUND ( 'NONE', #55248, .T. ) ;
#20990=CYLINDRICAL_SURFACE ( 'NONE', #11033, 7.937500000000000000 ) ;
#21004=CARTESIAN_POINT ( 'NONE',  ( -90.81826664112017511, 89.94786999841838337, -76.20774946062876154 ) ) ;
#21016=DIRECTION ( 'NONE',  ( -6.878358445406130340E-15, 0.000000000000000000, 1.000000000000000000 ) ) ;
#21024=ORIENTED_EDGE ( 'NONE', *, *, #4534, .F. ) ;
#21026=VECTOR ( 'NONE', #45008, 1000.000000000000000 ) ;
#21037=VECTOR ( 'NONE', #76836, 1000.000000000000000 ) ;
#21078=EDGE_LOOP ( 'NONE', ( #63838, #10809 ) ) ;
#21091=CARTESIAN_POINT ( 'NONE',  ( -91.11526841082567785, 75.84278307195157254, 75.85240403722379199 ) ) ;
#21125=ORIENTED_EDGE ( 'NONE', *, *, #70831, .F. ) ;
#21132=VECTOR ( 'NONE', #57382, 1000.000000000000000 ) ;
#21151=DIRECTION ( 'NONE',  ( 0.7071067811865560104, 0.000000000000000000, -0.7071067811865391350 ) ) ;
#21156=CARTESIAN_POINT ( 'NONE',  ( -130.1663562161751599, 74.81660785136578795, 10.08264331121449153 ) ) ;
#21164=VECTOR ( 'NONE', #5920, 1000.000000000000000 ) ;
#21187=CARTESIAN_POINT ( 'NONE',  ( -31.75000000000000000, 111.1250000000000000, -3.175000000000219647 ) ) ;
#21188=DIRECTION ( 'NONE',  ( 0.000000000000000000, -1.000000000000000000, 0.000000000000000000 ) ) ;
#21190=CARTESIAN_POINT ( 'NONE',  ( 77.39114642429960611, 120.6499999999999915, -71.77848634863110533 ) ) ;
#21217=CARTESIAN_POINT ( 'NONE',  ( -72.96458098368600531, 101.5999999999999943, -78.00648098368779415 ) ) ;
#21218=ADVANCED_FACE ( 'NONE', ( #87832 ), #5617, .F. ) ;
#21220=EDGE_CURVE ( 'NONE', #50419, #21337, #4262, .T. ) ;
#21231=LINE ( 'NONE', #48902, #58615 ) ;
#21251=EDGE_LOOP ( 'NONE', ( #333, #32516, #1053, #37883 ) ) ;
#21254=LINE ( 'NONE', #83480, #237 ) ;
#21261=EDGE_LOOP ( 'NONE', ( #17991, #9895, #22157, #22934 ) ) ;
#21288=CARTESIAN_POINT ( 'NONE',  ( 92.90380151374968420, 69.84937019662268654, 91.73035097708832097 ) ) ;
#21304=CARTESIAN_POINT ( 'NONE',  ( 92.06079644778121462, 79.26437155269051971, 74.70173812346128273 ) ) ;
#21308=ORIENTED_EDGE ( 'NONE', *, *, #63417, .F. ) ;
#21323=EDGE_CURVE ( 'NONE', #14083, #41448, #69625, .T. ) ;
#21326=CARTESIAN_POINT ( 'NONE',  ( -77.68727430814968216, 92.11680164986013608, 89.55756476669517951 ) ) ;
#21330=CARTESIAN_POINT ( 'NONE',  ( -118.4232890149586552, 93.94641470820113227, 5.620000134943238024 ) ) ;
#21333=CARTESIAN_POINT ( 'NONE',  ( 86.94609723791393208, 70.66242608954389937, -80.59807192910901108 ) ) ;
#21334=EDGE_LOOP ( 'NONE', ( #61897, #87495, #17185, #84543, #36399, #86501 ) ) ;
#21337=VERTEX_POINT ( 'NONE', #62349 ) ;
#21339=ORIENTED_EDGE ( 'NONE', *, *, #54480, .T. ) ;
#21349=CARTESIAN_POINT ( 'NONE',  ( 77.68727430815029322, 92.11680164986012187, -89.55756476669462529 ) ) ;
#21351=CARTESIAN_POINT ( 'NONE',  ( 77.89700433585288408, 82.54999999999999716, 59.93649209371626085 ) ) ;
#21355=AXIS2_PLACEMENT_3D ( 'NONE', #67429, #5219, #6556 ) ;
#21370=ORIENTED_EDGE ( 'NONE', *, *, #14742, .T. ) ;
#21374=CYLINDRICAL_SURFACE ( 'NONE', #40369, 12.69999999999999574 ) ;
#21391=CARTESIAN_POINT ( 'NONE',  ( -74.70281015415449133, 79.25941250729455589, -92.05992619857326531 ) ) ;
#21397=CARTESIAN_POINT ( 'NONE',  ( 3.110602869834275287E-15, 124.9679999999999893, 25.39999999999999858 ) ) ;
#21401=EDGE_CURVE ( 'NONE', #75109, #12810, #12879, .T. ) ;
#21432=DIRECTION ( 'NONE',  ( 0.000000000000000000, -1.000000000000000000, 0.000000000000000000 ) ) ;
#21434=CARTESIAN_POINT ( 'NONE',  ( -103.1875000000000000, 117.4749999999999943, 5.041899999998910253 ) ) ;
#21438=CARTESIAN_POINT ( 'NONE',  ( 74.15067561874209900, 120.6499999999999915, 68.53801554307469246 ) ) ;
#21441=VECTOR ( 'NONE', #17359, 1000.000000000000000 ) ;
#21458=CARTESIAN_POINT ( 'NONE',  ( -83.90387289223363609, 76.93632333215536789, -100.0252357601324462 ) ) ;
#21459=CARTESIAN_POINT ( 'NONE',  ( -77.69357874334708924, 92.12496802699139664, -89.55214429302399992 ) ) ;
#21463=AXIS2_PLACEMENT_3D ( 'NONE', #5661, #12469, #41937 ) ;
#21476=AXIS2_PLACEMENT_3D ( 'NONE', #27183, #6738, #83067 ) ;
#21482=CARTESIAN_POINT ( 'NONE',  ( 11.41184330286787940, 88.18497404666861428, 118.0059224074909849 ) ) ;
#21491=VECTOR ( 'NONE', #46334, 1000.000000000000114 ) ;
#21496=CIRCLE ( 'NONE', #30183, 5.041900000000001825 ) ;
#21537=DIRECTION ( 'NONE',  ( 0.000000000000000000, 1.000000000000000000, 0.000000000000000000 ) ) ;
#21557=LINE ( 'NONE', #1104, #39948 ) ;
#21572=CARTESIAN_POINT ( 'NONE',  ( 3.306647731859349904, 70.28099577563533273, 130.5147235605103617 ) ) ;
#21585=FACE_OUTER_BOUND ( 'NONE', #20832, .T. ) ;
#21610=CARTESIAN_POINT ( 'NONE',  ( -76.20505178924449297, 120.6499999999999915, 76.20505178924310030 ) ) ;
#21658=CARTESIAN_POINT ( 'NONE',  ( -7.205548786489490269E-13, 127.0000000000000000, 103.1875000000000000 ) ) ;
#21674=CARTESIAN_POINT ( 'NONE',  ( 98.06216817836198629, 92.11674985319542941, 86.19179098795370919 ) ) ;
#21679=DIRECTION ( 'NONE',  ( 0.7071067811865540120, 0.000000000000000000, -0.7071067811865410224 ) ) ;
#21698=CARTESIAN_POINT ( 'NONE',  ( -5.244287019405542871, 94.12413552026930574, 118.4405785268131410 ) ) ;
#21721=AXIS2_PLACEMENT_3D ( 'NONE', #56839, #9601, #16867 ) ;
#21732=FACE_BOUND ( 'NONE', #48592, .T. ) ;
#21749=CARTESIAN_POINT ( 'NONE',  ( 100.0338904447220898, 76.91670260214424104, 83.89393544538398828 ) ) ;
#21750=DIRECTION ( 'NONE',  ( 1.000000000000000000, 0.000000000000000000, 8.465970413060558704E-17 ) ) ;
#21779=DIRECTION ( 'NONE',  ( -3.278217592397115468E-15, 0.000000000000000000, 1.000000000000000000 ) ) ;
#21786=CARTESIAN_POINT ( 'NONE',  ( -85.28591416242345247, 95.08639429146514033, 82.35292268805530114 ) ) ;
#21792=DIRECTION ( 'NONE',  ( 0.000000000000000000, 0.000000000000000000, -1.000000000000000000 ) ) ;
#21810=CARTESIAN_POINT ( 'NONE',  ( 87.45628510944675327, 94.12556101775332706, -80.04418453221570928 ) ) ;
#21818=ORIENTED_EDGE ( 'NONE', *, *, #42477, .F. ) ;
#21826=EDGE_CURVE ( 'NONE', #26828, #26653, #82273, .T. ) ;
#21831=VECTOR ( 'NONE', #14011, 1000.000000000000000 ) ;
#21846=DIRECTION ( 'NONE',  ( 0.000000000000000000, 0.000000000000000000, 1.000000000000000000 ) ) ;
#21874=DIRECTION ( 'NONE',  ( -0.000000000000000000, 1.000000000000000000, 0.000000000000000000 ) ) ;
#21882=ORIENTED_EDGE ( 'NONE', *, *, #2698, .T. ) ;
#21886=CARTESIAN_POINT ( 'NONE',  ( -68.53801554307499089, 127.0000000000000000, 74.15067561874188584 ) ) ;
#21894=CARTESIAN_POINT ( 'NONE',  ( -3.175000000000120171, 111.1250000000000000, 33.98325472291465132 ) ) ;
#21895=ADVANCED_FACE ( 'NONE', ( #19569 ), #21374, .F. ) ;
#21914=CARTESIAN_POINT ( 'NONE',  ( -75.85717701425170389, 89.26692529358290074, -91.11128979799221383 ) ) ;
#21917=AXIS2_PLACEMENT_3D ( 'NONE', #22396, #56445, #50078 ) ;
#21948=EDGE_CURVE ( 'NONE', #78870, #9320, #2725, .T. ) ;
#21975=CARTESIAN_POINT ( 'NONE',  ( -12.70000000000000462, 82.96435431876527389, 129.9368274816651478 ) ) ;
#22002=CARTESIAN_POINT ( 'NONE',  ( -90.32738470895290561, 74.16215221268205937, 76.79083731950235858 ) ) ;
#22021=LINE ( 'NONE', #65121, #34245 ) ;
#22029=CARTESIAN_POINT ( 'NONE',  ( -99.33304294513271770, 89.94765885072627043, -84.72230615113613794 ) ) ;
#22033=EDGE_CURVE ( 'NONE', #14083, #1794, #43274, .T. ) ;
#22068=CARTESIAN_POINT ( 'NONE',  ( 130.5559380315087878, 69.85063703626886422, 0.8489233174145797145 ) ) ;
#22093=ORIENTED_EDGE ( 'NONE', *, *, #88459, .F. ) ;
#22118=EDGE_CURVE ( 'NONE', #9193, #2431, #17242, .T. ) ;
#22128=EDGE_CURVE ( 'NONE', #27158, #10599, #30867, .T. ) ;
#22146=CARTESIAN_POINT ( 'NONE',  ( -98.60478223830740774, 120.6499999999999915, -1.074461880482445986E-12 ) ) ;
#22153=CARTESIAN_POINT ( 'NONE',  ( -12.05172457139580011, 86.64129263485729382, 117.9422889837464510 ) ) ;
#22157=ORIENTED_EDGE ( 'NONE', *, *, #21323, .T. ) ;
#22179=CARTESIAN_POINT ( 'NONE',  ( -33.98325472291465132, 111.1250000000000000, 3.174999999999764899 ) ) ;
#22191=ORIENTED_EDGE ( 'NONE', *, *, #64421, .F. ) ;
#22192=FACE_OUTER_BOUND ( 'NONE', #37721, .T. ) ;
#22199=CARTESIAN_POINT ( 'NONE',  ( 103.1875000000000000, 127.0000000000000000, -5.041899999999640336 ) ) ;
#22205=ORIENTED_EDGE ( 'NONE', *, *, #8773, .T. ) ;
#22234=CARTESIAN_POINT ( 'NONE',  ( -74.62309654709146400, 85.43299024555680887, 92.12450916458723782 ) ) ;
#22236=CIRCLE ( 'NONE', #6266, 188.9759999999999991 ) ;
#22241=CARTESIAN_POINT ( 'NONE',  ( 87.72765544449647734, 71.14137858619483268, -79.74945239053471369 ) ) ;
#22265=ORIENTED_EDGE ( 'NONE', *, *, #13098, .F. ) ;
#22286=PLANE ( 'NONE',  #67845 ) ;
#22299=VECTOR ( 'NONE', #20791, 1000.000000000000000 ) ;
#22300=FACE_OUTER_BOUND ( 'NONE', #46687, .T. ) ;
#22307=CARTESIAN_POINT ( 'NONE',  ( 3.175000000000355094, 124.5870000000000033, -33.98325472291460159 ) ) ;
#22309=ORIENTED_EDGE ( 'NONE', *, *, #49782, .F. ) ;
#22315=DIRECTION ( 'NONE',  ( 0.000000000000000000, -1.000000000000000000, 0.000000000000000000 ) ) ;
#22356=CARTESIAN_POINT ( 'NONE',  ( -74.36911441044665594, 82.96450994655475597, -92.32962665258584423 ) ) ;
#22376=VECTOR ( 'NONE', #48628, 1000.000000000000000 ) ;
#22396=CARTESIAN_POINT ( 'NONE',  ( 103.1875000000000000, 127.0000000000000000, 3.602774393244745134E-13 ) ) ;
#22413=AXIS2_PLACEMENT_3D ( 'NONE', #61508, #47874, #67889 ) ;
#22419=ORIENTED_EDGE ( 'NONE', *, *, #1327, .T. ) ;
#22465=LINE ( 'NONE', #217, #62124 ) ;
#22482=ORIENTED_EDGE ( 'NONE', *, *, #6625, .F. ) ;
#22513=CIRCLE ( 'NONE', #44202, 5.041900000000001825 ) ;
#22529=ORIENTED_EDGE ( 'NONE', *, *, #67648, .F. ) ;
#22535=DIRECTION ( 'NONE',  ( 0.000000000000000000, 0.000000000000000000, -1.000000000000000000 ) ) ;
#22541=ORIENTED_EDGE ( 'NONE', *, *, #68053, .T. ) ;
#22543=CARTESIAN_POINT ( 'NONE',  ( -74.15067561874319324, 120.6499999999999915, 68.53801554307369770 ) ) ;
#22544=AXIS2_PLACEMENT_3D ( 'NONE', #30694, #23892, #71049 ) ;
#22549=VERTEX_POINT ( 'NONE', #72097 ) ;
#22570=CARTESIAN_POINT ( 'NONE',  ( 95.16508291382824325, 94.58014758961630264, 89.37916159652695569 ) ) ;
#22571=CARTESIAN_POINT ( 'NONE',  ( 2.684158038187649039E-15, 69.84999999999999432, -130.5560000000000116 ) ) ;
#22598=VECTOR ( 'NONE', #30856, 1000.000000000000114 ) ;
#22607=LINE ( 'NONE', #83943, #50317 ) ;
#22624=FACE_OUTER_BOUND ( 'NONE', #80029, .T. ) ;
#22647=LINE ( 'NONE', #23545, #73579 ) ;
#22659=DIRECTION ( 'NONE',  ( 0.9659258262890679791, 0.000000000000000000, -0.2588190451025220162 ) ) ;
#22664=CARTESIAN_POINT ( 'NONE',  ( -103.1875000000000000, 120.6499999999999915, -7.937500000001089795 ) ) ;
#22675=CARTESIAN_POINT ( 'NONE',  ( -103.1875000000000000, 117.4749999999999943, -1.080832317973422076E-12 ) ) ;
#22679=CARTESIAN_POINT ( 'NONE',  ( 78.57724105935530190, 120.6499999999999915, -67.35192090801849929 ) ) ;
#22685=CARTESIAN_POINT ( 'NONE',  ( -81.76533775135438020, 94.92435932957494060, 85.84941893669298452 ) ) ;
#22689=FACE_OUTER_BOUND ( 'NONE', #5396, .T. ) ;
#22703=CYLINDRICAL_SURFACE ( 'NONE', #78236, 7.143750000000004263 ) ;
#22731=VECTOR ( 'NONE', #17428, 999.9999999999998863 ) ;
#22740=CYLINDRICAL_SURFACE ( 'NONE', #31594, 5.041900000000001825 ) ;
#22765=ORIENTED_EDGE ( 'NONE', *, *, #44642, .F. ) ;
#22789=ORIENTED_EDGE ( 'NONE', *, *, #32084, .T. ) ;
#22793=FACE_OUTER_BOUND ( 'NONE', #41621, .T. ) ;
#22797=CARTESIAN_POINT ( 'NONE',  ( -93.48344774443276606, 95.14808745951972924, 91.13664476550712834 ) ) ;
#22809=CARTESIAN_POINT ( 'NONE',  ( -85.84941893669265767, 94.92435932957486955, -81.76533775135462179 ) ) ;
#22812=FACE_OUTER_BOUND ( 'NONE', #42758, .T. ) ;
#22832=EDGE_LOOP ( 'NONE', ( #29513, #23053, #87922, #5145 ) ) ;
#22836=CARTESIAN_POINT ( 'NONE',  ( 3.968749999999229949, 127.0000000000000000, 100.8961411191535973 ) ) ;
#22843=EDGE_CURVE ( 'NONE', #71309, #54367, #76444, .T. ) ;
#22853=DIRECTION ( 'NONE',  ( -0.000000000000000000, 1.000000000000000000, 0.000000000000000000 ) ) ;
#22867=CARTESIAN_POINT ( 'NONE',  ( 9.331435647859348646E-23, 95.25000000000000000, 130.5560000000000116 ) ) ;
#22880=CARTESIAN_POINT ( 'NONE',  ( 0.000000000000000000, 124.5870000000000033, 0.000000000000000000 ) ) ;
#22888=ORIENTED_EDGE ( 'NONE', *, *, #85560, .T. ) ;
#22899=VERTEX_POINT ( 'NONE', #29203 ) ;
#22907=CARTESIAN_POINT ( 'NONE',  ( 3.968750000000000000, 127.0000000000000000, -105.4788588808464027 ) ) ;
#22917=CARTESIAN_POINT ( 'NONE',  ( -103.1875000000000000, 127.0000000000000000, 7.143749999998919797 ) ) ;
#22934=ORIENTED_EDGE ( 'NONE', *, *, #31247, .T. ) ;
#22963=CARTESIAN_POINT ( 'NONE',  ( -130.4667021054748943, 70.80031572943160256, 4.873084223276297422 ) ) ;
#22968=ORIENTED_EDGE ( 'NONE', *, *, #59308, .F. ) ;
#22976=DIRECTION ( 'NONE',  ( 1.092739197465705130E-14, 0.000000000000000000, -1.000000000000000000 ) ) ;
#22977=FACE_OUTER_BOUND ( 'NONE', #39309, .T. ) ;
#22990=FACE_OUTER_BOUND ( 'NONE', #45919, .T. ) ;
#23012=CIRCLE ( 'NONE', #78122, 7.937500000000000000 ) ;
#23015=ORIENTED_EDGE ( 'NONE', *, *, #8266, .F. ) ;
#23018=DIRECTION ( 'NONE',  ( 0.000000000000000000, 0.000000000000000000, 1.000000000000000000 ) ) ;
#23021=CARTESIAN_POINT ( 'NONE',  ( 84.21071524772710859, 88.91113633199482535, 99.76704648670086328 ) ) ;
#23023=EDGE_CURVE ( 'NONE', #46913, #58480, #35548, .T. ) ;
#23025=LINE ( 'NONE', #9378, #73744 ) ;
#23030=CIRCLE ( 'NONE', #36040, 25.39999999999999858 ) ;
#23037=CARTESIAN_POINT ( 'NONE',  ( -103.1875000000000000, 127.0000000000000000, -7.937500000001080913 ) ) ;
#23053=ORIENTED_EDGE ( 'NONE', *, *, #4083, .F. ) ;
#23078=DIRECTION ( 'NONE',  ( 0.000000000000000000, 0.000000000000000000, -1.000000000000000000 ) ) ;
#23080=DIRECTION ( 'NONE',  ( 0.000000000000000000, -1.000000000000000000, 0.000000000000000000 ) ) ;
#23089=FACE_BOUND ( 'NONE', #39946, .T. ) ;
#23091=VERTEX_POINT ( 'NONE', #87294 ) ;
#23098=EDGE_CURVE ( 'NONE', #12422, #68005, #9496, .T. ) ;
#23109=CARTESIAN_POINT ( 'NONE',  ( 33.98325472291465132, 104.3431970271542042, -3.174999999999999822 ) ) ;
#23116=DIRECTION ( 'NONE',  ( 0.000000000000000000, 0.000000000000000000, -1.000000000000000000 ) ) ;
#23118=CIRCLE ( 'NONE', #39028, 7.143750000000004263 ) ;
#23120=CARTESIAN_POINT ( 'NONE',  ( 82.64146475440669803, 69.93366089391891194, 85.00925061401017047 ) ) ;
#23124=EDGE_LOOP ( 'NONE', ( #33266, #60870, #12317, #85954 ) ) ;
#23138=AXIS2_PLACEMENT_3D ( 'NONE', #167, #36032, #27868 ) ;
#23151=EDGE_CURVE ( 'NONE', #54126, #56554, #20882, .T. ) ;
#23153=ORIENTED_EDGE ( 'NONE', *, *, #2221, .F. ) ;
#23191=DIRECTION ( 'NONE',  ( 0.000000000000000000, 1.000000000000000000, 0.000000000000000000 ) ) ;
#23226=EDGE_LOOP ( 'NONE', ( #78536, #3617, #35124, #43743 ) ) ;
#23240=DIRECTION ( 'NONE',  ( 0.000000000000000000, 1.000000000000000000, 0.000000000000000000 ) ) ;
#23266=ORIENTED_EDGE ( 'NONE', *, *, #89696, .T. ) ;
#23275=CARTESIAN_POINT ( 'NONE',  ( 103.1875000000000000, 127.0000000000000000, 3.602774393244745134E-13 ) ) ;
#23280=EDGE_LOOP ( 'NONE', ( #1782, #3226, #33373, #31312 ) ) ;
#23306=EDGE_LOOP ( 'NONE', ( #52254, #28541 ) ) ;
#23311=ADVANCED_FACE ( 'NONE', ( #45383 ), #73103, .F. ) ;
#23314=LINE ( 'NONE', #77353, #16143 ) ;
#23368=CARTESIAN_POINT ( 'NONE',  ( -72.96458098368751166, 127.0000000000000000, 72.96458098368620426 ) ) ;
#23395=DIRECTION ( 'NONE',  ( 1.000000000000000000, 0.000000000000000000, 1.047445008332813989E-14 ) ) ;
#23403=ORIENTED_EDGE ( 'NONE', *, *, #4920, .T. ) ;
#23412=CARTESIAN_POINT ( 'NONE',  ( -130.0575199856854169, 76.93632333215535368, -11.39952500586003836 ) ) ;
#23416=EDGE_CURVE ( 'NONE', #37218, #69459, #60080, .T. ) ;
#23430=FACE_OUTER_BOUND ( 'NONE', #61624, .T. ) ;
#23454=CARTESIAN_POINT ( 'NONE',  ( -3.291704278000410433, 94.82304653311918230, -130.5151038487541655 ) ) ;
#23473=CARTESIAN_POINT ( 'NONE',  ( 80.04418453221538243, 94.12556101775334128, 87.45628510944696643 ) ) ;
#23518=ORIENTED_EDGE ( 'NONE', *, *, #45338, .T. ) ;
#23534=ORIENTED_EDGE ( 'NONE', *, *, #84995, .T. ) ;
#23540=EDGE_LOOP ( 'NONE', ( #78974, #24488, #74105, #1724 ) ) ;
#23544=CARTESIAN_POINT ( 'NONE',  ( 82.89895571708159139, 81.72130195885951309, 100.8594679592221155 ) ) ;
#23545=CARTESIAN_POINT ( 'NONE',  ( -3.174999999999644995, 104.3431970271541616, -33.98325472291465132 ) ) ;
#23561=CARTESIAN_POINT ( 'NONE',  ( 85.85227416678092993, 70.17658267799284033, 81.76234319299453546 ) ) ;
#23567=ORIENTED_EDGE ( 'NONE', *, *, #15336, .F. ) ;
#23575=CYLINDRICAL_SURFACE ( 'NONE', #39006, 12.70000000000000462 ) ;
#23580=ORIENTED_EDGE ( 'NONE', *, *, #1494, .F. ) ;
#23585=CARTESIAN_POINT ( 'NONE',  ( 92.32962665258614265, 81.72118090664558565, -74.36911441044638593 ) ) ;
#23593=VERTEX_POINT ( 'NONE', #50308 ) ;
#23604=FACE_OUTER_BOUND ( 'NONE', #59527, .T. ) ;
#23608=ORIENTED_EDGE ( 'NONE', *, *, #80409, .F. ) ;
#23653=DIRECTION ( 'NONE',  ( 0.000000000000000000, 0.000000000000000000, 1.000000000000000000 ) ) ;
#23666=PLANE ( 'NONE',  #2992 ) ;
#23667=CARTESIAN_POINT ( 'NONE',  ( 0.000000000000000000, 125.7300000000000040, 0.000000000000000000 ) ) ;
#23669=ADVANCED_FACE ( 'NONE', ( #51198 ), #84423, .F. ) ;
#23675=CARTESIAN_POINT ( 'NONE',  ( 3.175000000000355094, 104.3431970271541616, -33.98325472291460159 ) ) ;
#23691=CARTESIAN_POINT ( 'NONE',  ( -99.18048580889399091, 90.29814575435203494, 84.90178614994292161 ) ) ;
#23692=VECTOR ( 'NONE', #6073, 999.9999999999998863 ) ;
#23706=LINE ( 'NONE', #31380, #82424 ) ;
#23727=VERTEX_POINT ( 'NONE', #64406 ) ;
#23737=CARTESIAN_POINT ( 'NONE',  ( -5.635138049808393390, 71.13823012824934722, 130.4366002064613212 ) ) ;
#23742=CARTESIAN_POINT ( 'NONE',  ( -69.72411017813060141, 127.0000000000000000, 69.72411017812929401 ) ) ;
#23743=DIRECTION ( 'NONE',  ( 0.000000000000000000, 1.000000000000000000, 0.000000000000000000 ) ) ;
#23746=CARTESIAN_POINT ( 'NONE',  ( 1.598849875094818280E-14, 61.59999999999999432, -130.5560000000000116 ) ) ;
#23774=VERTEX_POINT ( 'NONE', #17153 ) ;
#23788=ADVANCED_FACE ( 'NONE', ( #52957 ), #32101, .F. ) ;
#23800=CARTESIAN_POINT ( 'NONE',  ( 118.4859477596447306, 70.52090377575430580, -4.094325160631359317 ) ) ;
#23820=CARTESIAN_POINT ( 'NONE',  ( -0.8399620612054651270, 69.85000000000003695, 118.5560000000000400 ) ) ;
#23847=CARTESIAN_POINT ( 'NONE',  ( -130.2059614519578759, 74.16222525595216553, -9.571858562769296697 ) ) ;
#23868=ORIENTED_EDGE ( 'NONE', *, *, #84286, .T. ) ;
#23892=DIRECTION ( 'NONE',  ( 0.000000000000000000, 1.000000000000000000, 0.000000000000000000 ) ) ;
#23903=CARTESIAN_POINT ( 'NONE',  ( 105.4788588808464027, 127.0000000000000000, 3.968750000000405009 ) ) ;
#23910=VECTOR ( 'NONE', #73589, 1000.000000000000114 ) ;
#23921=DIRECTION ( 'NONE',  ( 0.000000000000000000, -1.000000000000000000, 0.000000000000000000 ) ) ;
#23945=FACE_OUTER_BOUND ( 'NONE', #43707, .T. ) ;
#23998=CARTESIAN_POINT ( 'NONE',  ( 77.45828646618581104, 73.28361289573329884, 89.75424775947740841 ) ) ;
#24015=CARTESIAN_POINT ( 'NONE',  ( 0.000000000000000000, 127.0000000000000000, -110.3312500000000114 ) ) ;
#24020=FACE_OUTER_BOUND ( 'NONE', #89646, .T. ) ;
#24027=LINE ( 'NONE', #79446, #18977 ) ;
#24046=EDGE_CURVE ( 'NONE', #24962, #60191, #22513, .T. ) ;
#24068=EDGE_CURVE ( 'NONE', #2616, #25068, #27975, .T. ) ;
#24072=PLANE ( 'NONE',  #53356 ) ;
#24088=DIRECTION ( 'NONE',  ( 0.000000000000000000, 1.000000000000000000, 0.000000000000000000 ) ) ;
#24097=DIRECTION ( 'NONE',  ( 0.000000000000000000, -1.000000000000000000, 0.000000000000000000 ) ) ;
#24106=FACE_OUTER_BOUND ( 'NONE', #48290, .T. ) ;
#24108=CIRCLE ( 'NONE', #64688, 25.39999999999999858 ) ;
#24109=ORIENTED_EDGE ( 'NONE', *, *, #17984, .F. ) ;
#24117=CARTESIAN_POINT ( 'NONE',  ( -7.301849239715819957E-13, 120.6499999999999915, 98.60478223830740774 ) ) ;
#24122=ORIENTED_EDGE ( 'NONE', *, *, #82650, .F. ) ;
#24127=EDGE_CURVE ( 'NONE', #49254, #23727, #60695, .T. ) ;
#24148=ADVANCED_FACE ( 'NONE', ( #74790 ), #68431, .F. ) ;
#24180=VERTEX_POINT ( 'NONE', #28425 ) ;
#24190=CARTESIAN_POINT ( 'NONE',  ( 72.96458098368650269, 117.4749999999999943, 80.90208098368729850 ) ) ;
#24220=CARTESIAN_POINT ( 'NONE',  ( 105.4788588808464027, 120.6499999999999915, 3.968750000000405009 ) ) ;
#24234=LINE ( 'NONE', #51900, #66703 ) ;
#24236=CARTESIAN_POINT ( 'NONE',  ( 117.9723322394569891, 77.68452076096559722, 11.75283433610099593 ) ) ;
#24254=VERTEX_POINT ( 'NONE', #8904 ) ;
#24255=VERTEX_POINT ( 'NONE', #28888 ) ;
#24268=VERTEX_POINT ( 'NONE', #73329 ) ;
#24273=CARTESIAN_POINT ( 'NONE',  ( 0.000000000000000000, 125.7300000000000040, 0.000000000000000000 ) ) ;
#24275=ORIENTED_EDGE ( 'NONE', *, *, #30381, .T. ) ;
#24285=CARTESIAN_POINT ( 'NONE',  ( -130.5480269016124453, 69.93117631934792655, 1.660224752218731892 ) ) ;
#24325=CARTESIAN_POINT ( 'NONE',  ( -12.27464498081148214, 85.83590841536251048, -129.9777558447946717 ) ) ;
#24328=DIRECTION ( 'NONE',  ( 0.000000000000000000, -1.000000000000000000, 0.000000000000000000 ) ) ;
#24335=VERTEX_POINT ( 'NONE', #4748 ) ;
#24345=CARTESIAN_POINT ( 'NONE',  ( 2.883802008152356322, 70.17481864577712258, -130.5247784292598112 ) ) ;
#24351=ORIENTED_EDGE ( 'NONE', *, *, #30213, .T. ) ;
#24353=CARTESIAN_POINT ( 'NONE',  ( 10.33024153997673089, 89.94921403597288645, 130.1468737228267685 ) ) ;
#24392=FACE_BOUND ( 'NONE', #67493, .T. ) ;
#24402=CARTESIAN_POINT ( 'NONE',  ( 0.000000000000000000, 95.25000000000000000, 9.525000000000000355 ) ) ;
#24414=DIRECTION ( 'NONE',  ( 0.000000000000000000, 0.000000000000000000, 1.000000000000000000 ) ) ;
#24417=FACE_OUTER_BOUND ( 'NONE', #18408, .T. ) ;
#24426=EDGE_CURVE ( 'NONE', #24335, #30196, #53756, .T. ) ;
#24433=VECTOR ( 'NONE', #23191, 1000.000000000000000 ) ;
#24440=CARTESIAN_POINT ( 'NONE',  ( 84.41866557162614981, 69.84937538953987257, 83.24493215373445310 ) ) ;
#24452=CARTESIAN_POINT ( 'NONE',  ( 117.9171910823873048, 85.85031469618031963, 12.29178224785222895 ) ) ;
#24453=FACE_OUTER_BOUND ( 'NONE', #49790, .T. ) ;
#24458=VERTEX_POINT ( 'NONE', #48286 ) ;
#24463=CARTESIAN_POINT ( 'NONE',  ( -3.968749999999935163, 120.6499999999999915, -100.8961411191535973 ) ) ;
#24474=ORIENTED_EDGE ( 'NONE', *, *, #16573, .T. ) ;
#24488=ORIENTED_EDGE ( 'NONE', *, *, #31019, .T. ) ;
#24555=EDGE_LOOP ( 'NONE', ( #1702, #70108 ) ) ;
#24557=CARTESIAN_POINT ( 'NONE',  ( -72.96458098368600531, 127.0000000000000000, -72.96458098368781009 ) ) ;
#24560=VERTEX_POINT ( 'NONE', #40142 ) ;
#24566=CARTESIAN_POINT ( 'NONE',  ( -99.62873342662618370, 89.26666702275852572, 84.37439091330368512 ) ) ;
#24592=AXIS2_PLACEMENT_3D ( 'NONE', #1222, #28926, #23018 ) ;
#24651=ORIENTED_EDGE ( 'NONE', *, *, #10171, .T. ) ;
#24655=LINE ( 'NONE', #24220, #21132 ) ;
#24662=VECTOR ( 'NONE', #4066, 1000.000000000000114 ) ;
#24664=ORIENTED_EDGE ( 'NONE', *, *, #49782, .T. ) ;
#24675=CARTESIAN_POINT ( 'NONE',  ( 117.8738102209309062, 81.71068249639864689, -12.69999999999876827 ) ) ;
#24678=FACE_BOUND ( 'NONE', #17784, .T. ) ;
#24687=VECTOR ( 'NONE', #19993, 1000.000000000000000 ) ;
#24695=EDGE_CURVE ( 'NONE', #58480, #12034, #64518, .T. ) ;
#24696=CARTESIAN_POINT ( 'NONE',  ( -7.400192735666117905, 72.22046014531929359, 118.3253218772466511 ) ) ;
#24724=EDGE_LOOP ( 'NONE', ( #58101, #83524 ) ) ;
#24764=EDGE_LOOP ( 'NONE', ( #42119, #85746 ) ) ;
#24777=CIRCLE ( 'NONE', #14671, 7.937500000000000000 ) ;
#24785=CARTESIAN_POINT ( 'NONE',  ( 8.383129030752360933, 73.00074830044857777, -130.2869803084437592 ) ) ;
#24811=DIRECTION ( 'NONE',  ( 0.000000000000000000, 1.000000000000000000, 0.000000000000000000 ) ) ;
#24828=DIRECTION ( 'NONE',  ( -0.000000000000000000, 1.000000000000000000, -0.000000000000000000 ) ) ;
#24835=ORIENTED_EDGE ( 'NONE', *, *, #1213, .T. ) ;
#24855=VECTOR ( 'NONE', #28071, 1000.000000000000000 ) ;
#24862=DIRECTION ( 'NONE',  ( 0.000000000000000000, 1.000000000000000000, 0.000000000000000000 ) ) ;
#24894=CARTESIAN_POINT ( 'NONE',  ( 118.5108459337403701, 94.82191660594808980, -3.295896443148412569 ) ) ;
#24900=B_SPLINE_CURVE_WITH_KNOTS ( 'NONE', 3,
 ( #33735, #26916, #53245, #81013, #47789, #74177, #18759, #68706, #13738, #88272, #47342, #81902, #26472, #19653, #4691, #75070, #82353, #32372, #46443, #11957, #74617, #54591, #39641, #61425, #40088, #75524, #89152, #13298, #67343, #40987, #5131, #53696, #6472, #34165, #81463, #19213, #85037, #83686, #42318, #110, #21458, #70049, #6921, #55941, #77763, #29162, #36433, #64133 ),
 .UNSPECIFIED., .F., .F.,
 ( 4, 2, 2, 2, 2, 2, 2, 2, 2, 1, 2, 2, 2, 2, 2, 2, 2, 2, 2, 2, 2, 1, 2, 2, 4 ),
 ( 0.05959919981814693069, 0.06208168506169067097, 0.06332292768346255152, 0.06456417030523442513, 0.06704665554877820011, 0.06828789817055008760, 0.06952914079232196121, 0.07201162603586572231, 0.07325286865763758204, 0.07449411127940944177, 0.07573535390118130151, 0.07697659652295317512, 0.07945908176649690846, 0.08194156701004062793, 0.08318280963181251542, 0.08442405225358438903, 0.08690653749712810849, 0.08814778011889995435, 0.08938902274067181408, 0.09187150798421550579, 0.09311275060598732389, 0.09435399322775914199, 0.09559523584953097397, 0.09683647847130280595, 0.09931896371484646990 ),
 .UNSPECIFIED. ) ;
#24921=EDGE_CURVE ( 'NONE', #83340, #63421, #84042, .T. ) ;
#24928=CARTESIAN_POINT ( 'NONE',  ( -118.5107509192928603, 70.27900073646857493, 3.299277431129246541 ) ) ;
#24951=DIRECTION ( 'NONE',  ( 0.000000000000000000, 0.000000000000000000, 1.000000000000000000 ) ) ;
#24962=VERTEX_POINT ( 'NONE', #37556 ) ;
#24967=CARTESIAN_POINT ( 'NONE',  ( -129.9368274816651478, 82.54999999999999716, 12.69999999999954809 ) ) ;
#24969=CARTESIAN_POINT ( 'NONE',  ( 3.175000000000334666, 124.5870000000000033, -31.75000000000000000 ) ) ;
#24970=EDGE_LOOP ( 'NONE', ( #62665, #54014, #41862, #10052, #26772, #84532, #5966, #42843, #4363, #88411 ) ) ;
#24981=CARTESIAN_POINT ( 'NONE',  ( 100.7940789023227239, 84.21348395916258767, -82.97845804870311781 ) ) ;
#24996=CARTESIAN_POINT ( 'NONE',  ( 98.60478223830740774, 127.0000000000000000, 3.859079674607175002E-13 ) ) ;
#25010=CARTESIAN_POINT ( 'NONE',  ( -118.0447731586489652, 88.91144712388910420, -10.99980504627875533 ) ) ;
#25011=DIRECTION ( 'NONE',  ( 1.000000000000000000, 0.000000000000000000, 0.000000000000000000 ) ) ;
#25018=CARTESIAN_POINT ( 'NONE',  ( 0.000000000000000000, 127.0000000000000000, 0.000000000000000000 ) ) ;
#25032=EDGE_CURVE ( 'NONE', #3366, #66196, #28390, .T. ) ;
#25065=CARTESIAN_POINT ( 'NONE',  ( 5.210259806972410633E-15, 95.25000000000000000, -42.54500000000000171 ) ) ;
#25068=VERTEX_POINT ( 'NONE', #40213 ) ;
#25104=CARTESIAN_POINT ( 'NONE',  ( -86.19129576945097426, 72.98383416765815923, 98.06260288352420673 ) ) ;
#25107=ORIENTED_EDGE ( 'NONE', *, *, #29322, .T. ) ;
#25111=DIRECTION ( 'NONE',  ( 0.9659258262890680902, 0.000000000000000000, 0.2588190451025215166 ) ) ;
#25115=CARTESIAN_POINT ( 'NONE',  ( 118.3040894999503081, 72.45860812971085352, -7.755682336160053758 ) ) ;
#25123=ORIENTED_EDGE ( 'NONE', *, *, #21826, .T. ) ;
#25136=CARTESIAN_POINT ( 'NONE',  ( -11.75195648705195062, 77.68235131038592556, 117.9724202733717817 ) ) ;
#25215=ORIENTED_EDGE ( 'NONE', *, *, #57036, .F. ) ;
#25224=CARTESIAN_POINT ( 'NONE',  ( 92.06080542007410372, 85.83559868056555331, 74.70172715947595066 ) ) ;
#25247=CARTESIAN_POINT ( 'NONE',  ( -76.20505178924449297, 120.6499999999999915, 76.20505178924310030 ) ) ;
#25250=ADVANCED_FACE ( 'NONE', ( #11073 ), #4722, .F. ) ;
#25263=ORIENTED_EDGE ( 'NONE', *, *, #37965, .T. ) ;
#25270=DIRECTION ( 'NONE',  ( 0.000000000000000000, 1.000000000000000000, 0.000000000000000000 ) ) ;
#25315=DIRECTION ( 'NONE',  ( 0.000000000000000000, 1.000000000000000000, 0.000000000000000000 ) ) ;
#25328=CARTESIAN_POINT ( 'NONE',  ( 118.1268318574024505, 90.28416741362497078, -10.08204661438621841 ) ) ;
#25333=LINE ( 'NONE', #46206, #2768 ) ;
#25336=STYLED_ITEM ( 'NONE', ( #67264 ), #79963 ) ;
#25359=CARTESIAN_POINT ( 'NONE',  ( -118.4859477596447306, 70.52090377575432001, 4.094325160632186211 ) ) ;
#25365=EDGE_CURVE ( 'NONE', #24255, #2062, #43954, .T. ) ;
#25376=ORIENTED_EDGE ( 'NONE', *, *, #71843, .T. ) ;
#25378=EDGE_CURVE ( 'NONE', #2431, #5415, #55515, .T. ) ;
#25421=CARTESIAN_POINT ( 'NONE',  ( 97.63151088911762088, 92.64985122628468162, -86.68005309089086552 ) ) ;
#25425=CARTESIAN_POINT ( 'NONE',  ( -1.669011862100898913, 69.93236506402145380, -118.5470928879096562 ) ) ;
#25439=CARTESIAN_POINT ( 'NONE',  ( 97.46299999999996544, 82.54999999999999716, 1.020870737183004530E-12 ) ) ;
#25443=EDGE_CURVE ( 'NONE', #56554, #54126, #10630, .T. ) ;
#25451=CARTESIAN_POINT ( 'NONE',  ( -84.72230615113582530, 89.94765885072627043, 99.33304294513301613 ) ) ;
#25460=ORIENTED_EDGE ( 'NONE', *, *, #52507, .F. ) ;
#25478=ADVANCED_FACE ( 'NONE', ( #15574 ), #16019, .F. ) ;
#25486=CARTESIAN_POINT ( 'NONE',  ( 129.9449521816639788, 84.21449860606324478, -12.61764002986369171 ) ) ;
#25489=ORIENTED_EDGE ( 'NONE', *, *, #40574, .T. ) ;
#25499=AXIS2_PLACEMENT_3D ( 'NONE', #54809, #75287, #13064 ) ;
#25507=ORIENTED_EDGE ( 'NONE', *, *, #15614, .T. ) ;
#25514=DIRECTION ( 'NONE',  ( 1.000000000000000000, 0.000000000000000000, 6.982966722218760189E-15 ) ) ;
#25520=CARTESIAN_POINT ( 'NONE',  ( -72.96458098368751166, 101.5999999999999943, 72.96458098368620426 ) ) ;
#25552=EDGE_CURVE ( 'NONE', #8910, #61529, #35540, .T. ) ;
#25580=CYLINDRICAL_SURFACE ( 'NONE', #82189, 7.937500000000000000 ) ;
#25582=EDGE_CURVE ( 'NONE', #68811, #15841, #63713, .T. ) ;
#25592=ORIENTED_EDGE ( 'NONE', *, *, #88982, .F. ) ;
#25598=FACE_OUTER_BOUND ( 'NONE', #75762, .T. ) ;
#25629=CARTESIAN_POINT ( 'NONE',  ( 72.96458098368650269, 117.4749999999999943, 72.96458098368729850 ) ) ;
#25640=CARTESIAN_POINT ( 'NONE',  ( -7.301849239715819957E-13, 120.6499999999999915, 98.60478223830740774 ) ) ;
#25656=FACE_OUTER_BOUND ( 'NONE', #20828, .T. ) ;
#25673=CARTESIAN_POINT ( 'NONE',  ( -72.96458098368600531, 127.0000000000000000, -65.02708098368781009 ) ) ;
#25688=EDGE_LOOP ( 'NONE', ( #54259, #45049 ) ) ;
#25693=ORIENTED_EDGE ( 'NONE', *, *, #11484, .T. ) ;
#25695=EDGE_CURVE ( 'NONE', #45930, #6765, #80475, .T. ) ;
#25701=B_SPLINE_CURVE_WITH_KNOTS ( 'NONE', 3,
 ( #11105, #18367, #5653, #81526, #32892, #61045, #68322, #38813, #26984, #46507, #46951, #54650, #52846, #74243, #11574, #81966, #39265, #80618, #73332, #88775, #4751, #12018, #75131, #53309, #87424 ),
 .UNSPECIFIED., .F., .F.,
 ( 4, 2, 2, 1, 2, 2, 2, 2, 2, 2, 2, 2, 4 ),
 ( 0.03973448063954118648, 0.04221847903031242938, 0.04346047822569805430, 0.04470247742108367228, 0.04594447661646929720, 0.04718647581185492212, 0.04967047420262618584, 0.05091247339801183852, 0.05215447259339749120, 0.05463847098416878961, 0.05588047017955442841, 0.05712246937494005333, 0.05960646776571127542 ),
 .UNSPECIFIED. ) ;
#25719=CARTESIAN_POINT ( 'NONE',  ( -67.92268098368600704, 117.4749999999999943, -72.96458098368781009 ) ) ;
#25739=DIRECTION ( 'NONE',  ( 0.000000000000000000, 1.000000000000000000, 0.000000000000000000 ) ) ;
#25748=CARTESIAN_POINT ( 'NONE',  ( 5.244075232672828157, 94.12423341047686165, -130.4512049017868094 ) ) ;
#25749=CARTESIAN_POINT ( 'NONE',  ( 99.77245543246479542, 76.20343663217362007, -84.20430400022915762 ) ) ;
#25751=CARTESIAN_POINT ( 'NONE',  ( 6.174546696621020337E-16, 117.4749999999999943, -108.2293999999999983 ) ) ;
#25761=CARTESIAN_POINT ( 'NONE',  ( 68.53801554307389665, 120.6499999999999915, 74.15067561874289481 ) ) ;
#25765=LINE ( 'NONE', #67101, #84552 ) ;
#25819=CARTESIAN_POINT ( 'NONE',  ( -118.4860207371918221, 70.52018178143200089, -4.092354625462838236 ) ) ;
#25849=CARTESIAN_POINT ( 'NONE',  ( 69.72411017813010403, 120.6499999999999915, -69.72411017812979139 ) ) ;
#25863=CARTESIAN_POINT ( 'NONE',  ( -130.3837601098274490, 93.33885111288434189, 6.713053715883731343 ) ) ;
#25874=CARTESIAN_POINT ( 'NONE',  ( 95.16331303980187784, 94.60320878023495084, -89.38347482486616968 ) ) ;
#25881=AXIS2_PLACEMENT_3D ( 'NONE', #71032, #1082, #28794 ) ;
#25898=ORIENTED_EDGE ( 'NONE', *, *, #55622, .T. ) ;
#25901=AXIS2_PLACEMENT_3D ( 'NONE', #33560, #83509, #67637 ) ;
#25903=EDGE_LOOP ( 'NONE', ( #12480, #84561 ) ) ;
#25907=CARTESIAN_POINT ( 'NONE',  ( -118.0074504647927398, 88.17653575778737718, -11.39323553397000666 ) ) ;
#25910=VECTOR ( 'NONE', #53047, 1000.000000000000000 ) ;
#25929=ORIENTED_EDGE ( 'NONE', *, *, #83933, .F. ) ;
#25943=CARTESIAN_POINT ( 'NONE',  ( 130.4355093393840832, 93.94653598907720493, -5.619751006018297801 ) ) ;
#25975=DIRECTION ( 'NONE',  ( 0.000000000000000000, 1.000000000000000000, 0.000000000000000000 ) ) ;
#25987=FACE_OUTER_BOUND ( 'NONE', #82737, .T. ) ;
#25994=ADVANCED_FACE ( 'NONE', ( #29987 ), #16354, .F. ) ;
#26007=CYLINDRICAL_SURFACE ( 'NONE', #19594, 130.5560000000000116 ) ;
#26028=EDGE_LOOP ( 'NONE', ( #12817, #52497, #9302, #52263 ) ) ;
#26056=DIRECTION ( 'NONE',  ( -0.000000000000000000, 1.000000000000000000, -0.000000000000000000 ) ) ;
#26073=DIRECTION ( 'NONE',  ( 0.000000000000000000, -1.000000000000000000, 0.000000000000000000 ) ) ;
#26082=FACE_OUTER_BOUND ( 'NONE', #14431, .T. ) ;
#26086=VECTOR ( 'NONE', #36561, 1000.000000000000000 ) ;
#26130=B_SPLINE_CURVE_WITH_KNOTS ( 'NONE', 3,
 ( #34774, #6187, #62477, #61570, #89306, #27070, #54740, #82503, #41128, #27957, #21156, #65163, #51079, #2507, #2948, #10202, #70653, #78378, #22963, #86074, #43815, #71555, #24285, #8885, #85637, #8427, #17024, #37909, #71110, #2059, #77918, #86516, #57449, #29319, #16140, #31083, #23847, #79262, #65609, #85191, #23412, #44707, #9317, #3390, #37018, #30649, #36584, #58345 ),
 .UNSPECIFIED., .F., .F.,
 ( 4, 2, 2, 2, 2, 2, 2, 2, 2, 1, 2, 2, 2, 2, 2, 2, 2, 2, 2, 2, 2, 1, 2, 2, 4 ),
 ( 0.05959919981814688211, 0.06208168506169060852, 0.06332292768346245437, 0.06456417030523430023, 0.06704665554877801970, 0.06828789817054987943, 0.06952914079232173916, 0.07201162603586545863, 0.07325286865763731836, 0.07449411127940917809, 0.07573535390118102395, 0.07697659652295288368, 0.07945908176649660315, 0.08194156701004032262, 0.08318280963181218235, 0.08442405225358404208, 0.08690653749712776155, 0.08814778011889962128, 0.08938902274067148102, 0.09187150798421522824, 0.09311275060598708797, 0.09435399322775894770, 0.09559523584953080744, 0.09683647847130266717, 0.09931896371484638664 ),
 .UNSPECIFIED. ) ;
#26132=DIRECTION ( 'NONE',  ( 0.000000000000000000, 0.000000000000000000, 1.000000000000000000 ) ) ;
#26141=FACE_OUTER_BOUND ( 'NONE', #46777, .T. ) ;
#26144=CARTESIAN_POINT ( 'NONE',  ( 0.000000000000000000, 125.7300000000000040, 0.000000000000000000 ) ) ;
#26149=PRODUCT_DEFINITION_FORMATION_WITH_SPECIFIED_SOURCE ( 'ANY', '', #75331, .NOT_KNOWN. ) ;
#26155=CARTESIAN_POINT ( 'NONE',  ( 72.96458098368701428, 127.0000000000000000, -72.96458098368670164 ) ) ;
#26194=CARTESIAN_POINT ( 'NONE',  ( -105.4788588808462038, 127.0000000000000000, -3.968750000001139977 ) ) ;
#26203=CARTESIAN_POINT ( 'NONE',  ( 0.8301116440132043639, 95.22976338641700522, -130.5540265925894801 ) ) ;
#26224=DIRECTION ( 'NONE',  ( 8.659560562355121445E-17, -0.7071067811865315855, 0.7071067811865634489 ) ) ;
#26228=CARTESIAN_POINT ( 'NONE',  ( 118.5385583271987855, 95.08639429146512612, 2.073938160689064336 ) ) ;
#26232=EDGE_CURVE ( 'NONE', #22899, #39347, #53052, .T. ) ;
#26271=CARTESIAN_POINT ( 'NONE',  ( 6.364907348149458244, 71.52879593750107290, -118.3870396030140029 ) ) ;
#26272=DIRECTION ( 'NONE',  ( 0.000000000000000000, 1.000000000000000000, 0.000000000000000000 ) ) ;
#26282=DIRECTION ( 'NONE',  ( 0.000000000000000000, -1.000000000000000000, 0.000000000000000000 ) ) ;
#26315=EDGE_CURVE ( 'NONE', #37237, #41991, #74437, .T. ) ;
#26320=CARTESIAN_POINT ( 'NONE',  ( 83.41565754067528360, 86.63355734047006251, -100.4326241145867300 ) ) ;
#26334=ORIENTED_EDGE ( 'NONE', *, *, #15336, .T. ) ;
#26345=EDGE_CURVE ( 'NONE', #14963, #24180, #2023, .T. ) ;
#26356=FACE_OUTER_BOUND ( 'NONE', #61549, .T. ) ;
#26362=DIRECTION ( 'NONE',  ( 0.000000000000000000, 0.000000000000000000, -1.000000000000000000 ) ) ;
#26377=FACE_BOUND ( 'NONE', #6457, .T. ) ;
#26386=CARTESIAN_POINT ( 'NONE',  ( 130.1098569802757652, 89.26666702275853993, 10.78644903371371733 ) ) ;
#26397=CARTESIAN_POINT ( 'NONE',  ( -12.03356702080700202, 78.46872568947895843, -130.0002966128845969 ) ) ;
#26405=EDGE_LOOP ( 'NONE', ( #74014, #35538, #68185, #41196 ) ) ;
#26419=FACE_OUTER_BOUND ( 'NONE', #44552, .T. ) ;
#26455=ORIENTED_EDGE ( 'NONE', *, *, #7102, .F. ) ;
#26462=DIRECTION ( 'NONE',  ( 0.000000000000000000, 0.000000000000000000, 1.000000000000000000 ) ) ;
#26464=FACE_OUTER_BOUND ( 'NONE', #10738, .T. ) ;
#26465=CARTESIAN_POINT ( 'NONE',  ( -107.7702177616926065, 120.6499999999999915, -1.170464777364108012E-12 ) ) ;
#26472=CARTESIAN_POINT ( 'NONE',  ( -98.64078293412680409, 73.86195533656251655, -85.52748787272817310 ) ) ;
#26482=DIRECTION ( 'NONE',  ( -0.7071067811865512365, 0.000000000000000000, 0.7071067811865436870 ) ) ;
#26516=ORIENTED_EDGE ( 'NONE', *, *, #10468, .F. ) ;
#26534=ORIENTED_EDGE ( 'NONE', *, *, #13297, .F. ) ;
#26550=VECTOR ( 'NONE', #86452, 1000.000000000000114 ) ;
#26574=VERTEX_POINT ( 'NONE', #24402 ) ;
#26578=CARTESIAN_POINT ( 'NONE',  ( -103.1875000000000000, 127.0000000000000000, -1.080832317973422076E-12 ) ) ;
#26633=ORIENTED_EDGE ( 'NONE', *, *, #40750, .T. ) ;
#26653=VERTEX_POINT ( 'NONE', #72550 ) ;
#26663=ORIENTED_EDGE ( 'NONE', *, *, #65372, .T. ) ;
#26664=ORIENTED_EDGE ( 'NONE', *, *, #82457, .F. ) ;
#26665=CIRCLE ( 'NONE', #78889, 118.5560000000000116 ) ;
#26672=CARTESIAN_POINT ( 'NONE',  ( 1.451892247740217613E-14, 95.25000000000000000, -118.5560000000000116 ) ) ;
#26707=CARTESIAN_POINT ( 'NONE',  ( 10.09446275336743781, 74.79825716961998694, -118.1263904669630733 ) ) ;
#26734=EDGE_CURVE ( 'NONE', #30196, #38484, #47042, .T. ) ;
#26747=CARTESIAN_POINT ( 'NONE',  ( -129.9681618895518795, 85.43248893795410481, 12.37548408773453623 ) ) ;
#26755=PLANE ( 'NONE',  #64137 ) ;
#26756=CARTESIAN_POINT ( 'NONE',  ( 99.18048580889457355, 90.29814575435202073, -84.90178614994225370 ) ) ;
#26760=CARTESIAN_POINT ( 'NONE',  ( -12.27510648567648133, 79.26588701359587219, -117.9188774285743762 ) ) ;
#26762=EDGE_CURVE ( 'NONE', #20160, #59338, #14685, .T. ) ;
#26772=ORIENTED_EDGE ( 'NONE', *, *, #85286, .F. ) ;
#26775=CYLINDRICAL_SURFACE ( 'NONE', #60177, 12.70000000000000107 ) ;
#26787=CARTESIAN_POINT ( 'NONE',  ( -118.5560163110023808, 95.25015226514366873, -0.4098827902168798998 ) ) ;
#26814=AXIS2_PLACEMENT_3D ( 'NONE', #89655, #19701, #81512 ) ;
#26826=CARTESIAN_POINT ( 'NONE',  ( 130.5461193570662601, 95.14808745951974345, 1.659440300508242760 ) ) ;
#26828=VERTEX_POINT ( 'NONE', #58244 ) ;
#26836=CARTESIAN_POINT ( 'NONE',  ( -1.668880554893940493, 69.93234144696143062, -130.5479136978233896 ) ) ;
#26864=FACE_OUTER_BOUND ( 'NONE', #66548, .T. ) ;
#26867=VECTOR ( 'NONE', #74804, 1000.000000000000000 ) ;
#26889=CARTESIAN_POINT ( 'NONE',  ( 0.000000000000000000, 127.0000000000000000, -103.1875000000000000 ) ) ;
#26892=CARTESIAN_POINT ( 'NONE',  ( -100.0252357601321762, 76.93632333215533947, 83.90387289223399137 ) ) ;
#26901=PLANE ( 'NONE',  #68037 ) ;
#26903=CARTESIAN_POINT ( 'NONE',  ( 0.000000000000000000, 101.5999999999999943, 88.90000000000000568 ) ) ;
#26912=ORIENTED_EDGE ( 'NONE', *, *, #53723, .F. ) ;
#26916=CARTESIAN_POINT ( 'NONE',  ( -100.8594679592207086, 81.71102547120852932, -82.89895571708335353 ) ) ;
#26951=DIRECTION ( 'NONE',  ( 0.000000000000000000, 0.000000000000000000, 1.000000000000000000 ) ) ;
#26984=CARTESIAN_POINT ( 'NONE',  ( -6.350224805574129938, 93.55624312175208956, -118.3863781049609685 ) ) ;
#27000=ORIENTED_EDGE ( 'NONE', *, *, #55187, .F. ) ;
#27056=ORIENTED_EDGE ( 'NONE', *, *, #65981, .F. ) ;
#27070=CARTESIAN_POINT ( 'NONE',  ( -130.0003553321326990, 78.46683822717000112, 12.03293382262464206 ) ) ;
#27075=VECTOR ( 'NONE', #57320, 1000.000000000000000 ) ;
#27081=CARTESIAN_POINT ( 'NONE',  ( 105.4788588808464027, 127.0000000000000000, 3.968750000000405009 ) ) ;
#27096=DIRECTION ( 'NONE',  ( 0.000000000000000000, 0.000000000000000000, 1.000000000000000000 ) ) ;
#27111=ORIENTED_EDGE ( 'NONE', *, *, #50507, .T. ) ;
#27146=VERTEX_POINT ( 'NONE', #48613 ) ;
#27150=VERTEX_POINT ( 'NONE', #40484 ) ;
#27153=CARTESIAN_POINT ( 'NONE',  ( -12.59756045763256793, 84.21337188079044722, 117.8848095194958034 ) ) ;
#27158=VERTEX_POINT ( 'NONE', #21397 ) ;
#27166=CARTESIAN_POINT ( 'NONE',  ( 11.75195648705195062, 77.68235131038592556, -117.9724202733717817 ) ) ;
#27174=ORIENTED_EDGE ( 'NONE', *, *, #66045, .F. ) ;
#27183=CARTESIAN_POINT ( 'NONE',  ( 0.000000000000000000, 95.25000000000000000, 0.000000000000000000 ) ) ;
#27200=CARTESIAN_POINT ( 'NONE',  ( 90.25011051337631329, 70.17666187254640420, 94.33955404248759180 ) ) ;
#27210=LINE ( 'NONE', #19502, #51027 ) ;
#27243=CARTESIAN_POINT ( 'NONE',  ( 86.67600044576353469, 70.52018178143200089, -80.88853703239280435 ) ) ;
#27245=DIRECTION ( 'NONE',  ( 0.000000000000000000, -1.000000000000000000, 0.000000000000000000 ) ) ;
#27252=VECTOR ( 'NONE', #61619, 1000.000000000000000 ) ;
#27256=DIRECTION ( 'NONE',  ( 0.8660254037844381525, 0.000000000000000000, 0.5000000000000007772 ) ) ;
#27268=ORIENTED_EDGE ( 'NONE', *, *, #238, .T. ) ;
#27278=CARTESIAN_POINT ( 'NONE',  ( 130.5480414536683895, 95.16896684734908263, -1.658263961149670118 ) ) ;
#27287=ORIENTED_EDGE ( 'NONE', *, *, #29285, .F. ) ;
#27308=EDGE_CURVE ( 'NONE', #28373, #69770, #33466, .T. ) ;
#27319=CARTESIAN_POINT ( 'NONE',  ( 11.89159109876203146, 78.07192968827520474, 117.9582163940502966 ) ) ;
#27363=DIRECTION ( 'NONE',  ( 0.000000000000000000, 0.000000000000000000, 1.000000000000000000 ) ) ;
#27382=VECTOR ( 'NONE', #77041, 1000.000000000000000 ) ;
#27428=FACE_OUTER_BOUND ( 'NONE', #53680, .T. ) ;
#27433=LINE ( 'NONE', #55112, #51459 ) ;
#27436=EDGE_LOOP ( 'NONE', ( #77779, #22205, #73954, #63135 ) ) ;
#27438=EDGE_LOOP ( 'NONE', ( #76215, #72071 ) ) ;
#27440=AXIS2_PLACEMENT_3D ( 'NONE', #75977, #48245, #26482 ) ;
#27473=CARTESIAN_POINT ( 'NONE',  ( -82.89895571708225930, 82.96445444011520465, -100.8594679592215329 ) ) ;
#27480=EDGE_LOOP ( 'NONE', ( #22191, #39475, #52552, #7704 ) ) ;
#27485=ORIENTED_EDGE ( 'NONE', *, *, #88683, .T. ) ;
#27510=CARTESIAN_POINT ( 'NONE',  ( 130.1093520674643287, 75.84295037288963215, 10.79257909650501013 ) ) ;
#27512=ORIENTED_EDGE ( 'NONE', *, *, #84562, .F. ) ;
#27531=EDGE_CURVE ( 'NONE', #29629, #40068, #72233, .T. ) ;
#27547=CARTESIAN_POINT ( 'NONE',  ( -69.72411017812909506, 120.6499999999999915, -69.72411017813089984 ) ) ;
#27554=ORIENTED_EDGE ( 'NONE', *, *, #25032, .F. ) ;
#27578=CARTESIAN_POINT ( 'NONE',  ( -77.39114642429849766, 120.6499999999999915, -71.77848634863219957 ) ) ;
#27588=DIRECTION ( 'NONE',  ( 0.000000000000000000, 0.000000000000000000, 1.000000000000000000 ) ) ;
#27589=CIRCLE ( 'NONE', #78395, 7.143750000000001599 ) ;
#27593=VERTEX_POINT ( 'NONE', #73556 ) ;
#27595=ORIENTED_EDGE ( 'NONE', *, *, #57971, .T. ) ;
#27604=CARTESIAN_POINT ( 'NONE',  ( -117.9190617242382046, 79.25941250729457010, -12.27333445685015967 ) ) ;
#27605=ORIENTED_EDGE ( 'NONE', *, *, #48735, .F. ) ;
#27608=LINE ( 'NONE', #48920, #58618 ) ;
#27612=CARTESIAN_POINT ( 'NONE',  ( 5.635505087355097587, 71.13841253056517644, -118.4244851085658468 ) ) ;
#27627=ADVANCED_FACE ( 'NONE', ( #20401 ), #33564, .F. ) ;
#27643=ORIENTED_EDGE ( 'NONE', *, *, #46375, .F. ) ;
#27650=CARTESIAN_POINT ( 'NONE',  ( 98.64078293412623566, 73.86195533656253076, 85.52748787272882680 ) ) ;
#27667=EDGE_CURVE ( 'NONE', #22899, #50035, #24777, .T. ) ;
#27668=CARTESIAN_POINT ( 'NONE',  ( -100.8961411191535973, 127.0000000000000000, -3.968750000001104894 ) ) ;
#27679=FACE_OUTER_BOUND ( 'NONE', #42620, .T. ) ;
#27686=ORIENTED_EDGE ( 'NONE', *, *, #35254, .T. ) ;
#27724=LINE ( 'NONE', #61776, #10291 ) ;
#27755=AXIS2_PLACEMENT_3D ( 'NONE', #41152, #54764, #82534 ) ;
#27773=CARTESIAN_POINT ( 'NONE',  ( 107.7702177616926065, 127.0000000000000000, 4.179089330879380409E-13 ) ) ;
#27787=CARTESIAN_POINT ( 'NONE',  ( -100.5868491334642272, 79.25971567868505474, 83.22961976134736517 ) ) ;
#27805=ORIENTED_EDGE ( 'NONE', *, *, #78527, .F. ) ;
#27806=VERTEX_POINT ( 'NONE', #84873 ) ;
#27809=CARTESIAN_POINT ( 'NONE',  ( -91.90730674524679955, 86.63388195152285221, -74.89049941105116659 ) ) ;
#27827=B_SPLINE_CURVE_WITH_KNOTS ( 'NONE', 3,
 ( #68050, #67147, #19005, #45345, #4928, #53940, #86714, #66240, #46233, #73066, #4032, #87601, #5376, #52593, #31732, #59430, #60318, #73969, #46688, #25359, #24928, #80349, #18100, #53031, #45787, #33076, #88056, #11287, #25819, #73515, #38991, #66699, #48461, #7173, #75313, #69397, #19899, #82150, #35299, #89399, #13094, #14440, #42117, #27604, #6711, #13979, #62121, #62570 ),
 .UNSPECIFIED., .F., .F.,
 ( 4, 2, 2, 2, 2, 2, 2, 2, 2, 1, 2, 2, 2, 2, 2, 2, 2, 2, 2, 2, 2, 1, 2, 2, 4 ),
 ( 0.05960646776571126848, 0.06208927922045070352, 0.06333068494782041757, 0.06457209067519013856, 0.06705490212992959442, 0.06829630785729932929, 0.06953771358466906416, 0.07202052503940857553, 0.07326193076677831040, 0.07450333649414805914, 0.07574474222151779401, 0.07698614794888752888, 0.07946895940362701249, 0.08195177085836649611, 0.08319317658573623098, 0.08443458231310596585, 0.08691739376784544946, 0.08815879949521518433, 0.08940020522258490532, 0.09188301667732433342, 0.09312442240469404053, 0.09436582813206376152, 0.09560723385943348251, 0.09684863958680320351, 0.09933145104154258997 ),
 .UNSPECIFIED. ) ;
#27833=CARTESIAN_POINT ( 'NONE',  ( 1.654053778667920804, 95.16954379564978694, 118.5472977239360972 ) ) ;
#27843=EDGE_CURVE ( 'NONE', #63081, #58666, #2192, .T. ) ;
#27868=DIRECTION ( 'NONE',  ( 0.000000000000000000, 0.000000000000000000, 1.000000000000000000 ) ) ;
#27871=ORIENTED_EDGE ( 'NONE', *, *, #30435, .F. ) ;
#27896=CARTESIAN_POINT ( 'NONE',  ( -81.46681417397449820, 70.27900073646854651, 86.13269706310923368 ) ) ;
#27899=VERTEX_POINT ( 'NONE', #16268 ) ;
#27926=ORIENTED_EDGE ( 'NONE', *, *, #79574, .F. ) ;
#27928=DIRECTION ( 'NONE',  ( 0.000000000000000000, 0.000000000000000000, 1.000000000000000000 ) ) ;
#27929=VERTEX_POINT ( 'NONE', #37155 ) ;
#27957=CARTESIAN_POINT ( 'NONE',  ( -130.1467648208192713, 75.15271101351808625, 10.33160863867537316 ) ) ;
#27960=DIRECTION ( 'NONE',  ( 1.000000000000000000, 0.000000000000000000, 0.000000000000000000 ) ) ;
#27965=DIRECTION ( 'NONE',  ( 0.000000000000000000, 0.000000000000000000, 1.000000000000000000 ) ) ;
#27972=DIRECTION ( 'NONE',  ( 0.000000000000000000, 1.000000000000000000, 0.000000000000000000 ) ) ;
#27975=LINE ( 'NONE', #83402, #29772 ) ;
#27988=DIRECTION ( 'NONE',  ( -0.000000000000000000, 1.000000000000000000, 0.000000000000000000 ) ) ;
#27997=ORIENTED_EDGE ( 'NONE', *, *, #3964, .T. ) ;
#28006=VERTEX_POINT ( 'NONE', #87093 ) ;
#28013=CARTESIAN_POINT ( 'NONE',  ( 98.64044413062926253, 91.23859726994550101, 85.52787878288761192 ) ) ;
#28019=CARTESIAN_POINT ( 'NONE',  ( -105.4788588808464027, 120.6499999999999915, 3.968749999998844924 ) ) ;
#28024=EDGE_CURVE ( 'NONE', #69770, #28373, #74117, .T. ) ;
#28028=FACE_OUTER_BOUND ( 'NONE', #54785, .T. ) ;
#28044=CARTESIAN_POINT ( 'NONE',  ( 77.39114642429960611, 120.6499999999999915, -71.77848634863110533 ) ) ;
#28055=EDGE_CURVE ( 'NONE', #72426, #83684, #89785, .T. ) ;
#28062=DIRECTION ( 'NONE',  ( 0.000000000000000000, 0.000000000000000000, 1.000000000000000000 ) ) ;
#28071=DIRECTION ( 'NONE',  ( 0.000000000000000000, 1.000000000000000000, 0.000000000000000000 ) ) ;
#28085=CARTESIAN_POINT ( 'NONE',  ( 86.19613171056606404, 73.00415124681447310, 98.05713019660873897 ) ) ;
#28103=VERTEX_POINT ( 'NONE', #6212 ) ;
#28111=DIRECTION ( 'NONE',  ( 0.000000000000000000, 0.000000000000000000, -1.000000000000000000 ) ) ;
#28116=ORIENTED_EDGE ( 'NONE', *, *, #3352, .F. ) ;
#28117=CARTESIAN_POINT ( 'NONE',  ( -91.11128979799197225, 89.26692529358290074, 75.85717701425203074 ) ) ;
#28121=CARTESIAN_POINT ( 'NONE',  ( -118.2599598282757114, 92.11680164986013608, 8.393562877891261209 ) ) ;
#28123=ADVANCED_FACE ( 'NONE', ( #68437 ), #7105, .F. ) ;
#28124=ADVANCED_FACE ( 'NONE', ( #81188 ), #55219, .F. ) ;
#28174=CARTESIAN_POINT ( 'NONE',  ( -7.759765182912740755, 72.46180059790658845, -130.3270382739332831 ) ) ;
#28182=CARTESIAN_POINT ( 'NONE',  ( -74.36911441044668436, 82.54999999999999716, -92.32962665258587265 ) ) ;
#28184=CARTESIAN_POINT ( 'NONE',  ( 0.000000000000000000, 124.5870000000000033, 0.000000000000000000 ) ) ;
#28187=CARTESIAN_POINT ( 'NONE',  ( 105.4788588808462038, 120.6499999999999915, -3.968749999999580336 ) ) ;
#28192=EDGE_LOOP ( 'NONE', ( #44740, #387 ) ) ;
#28197=CARTESIAN_POINT ( 'NONE',  ( 90.24991642302090611, 70.17656663518266669, -94.33976020835932275 ) ) ;
#28217=CARTESIAN_POINT ( 'NONE',  ( -3.968749999999935163, 120.6499999999999915, -100.8961411191535973 ) ) ;
#28225=DIRECTION ( 'NONE',  ( 0.000000000000000000, 0.000000000000000000, -1.000000000000000000 ) ) ;
#28227=CARTESIAN_POINT ( 'NONE',  ( -87.71474477836267170, 71.54617234588346264, 96.70122665881213209 ) ) ;
#28249=CARTESIAN_POINT ( 'NONE',  ( -91.26325766987453392, 88.91291927174614784, -75.67533895324370974 ) ) ;
#28251=CARTESIAN_POINT ( 'NONE',  ( 92.32962665258456525, 82.54999999999999716, 74.36911441044829019 ) ) ;
#28254=FACE_OUTER_BOUND ( 'NONE', #41812, .T. ) ;
#28304=CARTESIAN_POINT ( 'NONE',  ( -5.624702496966066612, 93.94413577832827400, 130.4352985349312632 ) ) ;
#28321=ORIENTED_EDGE ( 'NONE', *, *, #52507, .T. ) ;
#28331=DIRECTION ( 'NONE',  ( 0.000000000000000000, 1.000000000000000000, 0.000000000000000000 ) ) ;
#28333=CARTESIAN_POINT ( 'NONE',  ( -88.21655330423224939, 71.53193882405246029, 79.20758933349385700 ) ) ;
#28356=ORIENTED_EDGE ( 'NONE', *, *, #31247, .F. ) ;
#28358=EDGE_LOOP ( 'NONE', ( #1254, #45418 ) ) ;
#28363=CARTESIAN_POINT ( 'NONE',  ( -100.8594679592206518, 83.38918798244688446, -82.89895571708331090 ) ) ;
#28369=VECTOR ( 'NONE', #61825, 1000.000000000000000 ) ;
#28373=VERTEX_POINT ( 'NONE', #8912 ) ;
#28375=CARTESIAN_POINT ( 'NONE',  ( 105.4788588808464027, 120.6499999999999915, 3.968750000000405009 ) ) ;
#28390=CIRCLE ( 'NONE', #42902, 7.937500000000000000 ) ;
#28402=CARTESIAN_POINT ( 'NONE',  ( 130.0261948852675005, 77.68489675156568808, 11.75299070208665597 ) ) ;
#28409=CIRCLE ( 'NONE', #8129, 7.937500000000000000 ) ;
#28425=CARTESIAN_POINT ( 'NONE',  ( 0.000000000000000000, 95.25000000000000000, 38.10000000000000142 ) ) ;
#28439=LINE ( 'NONE', #43402, #13210 ) ;
#28462=CARTESIAN_POINT ( 'NONE',  ( 90.83954799657384171, 95.08644067748865325, 93.77212533081443269 ) ) ;
#28487=CARTESIAN_POINT ( 'NONE',  ( -10.09762896578686409, 90.29673011329586529, 118.1261022283270421 ) ) ;
#28517=FACE_BOUND ( 'NONE', #71398, .T. ) ;
#28524=DIRECTION ( 'NONE',  ( 0.000000000000000000, 0.000000000000000000, 1.000000000000000000 ) ) ;
#28531=CARTESIAN_POINT ( 'NONE',  ( 0.000000000000000000, 101.5999999999999943, 0.000000000000000000 ) ) ;
#28541=ORIENTED_EDGE ( 'NONE', *, *, #2352, .T. ) ;
#28575=DIRECTION ( 'NONE',  ( 1.000000000000000000, 0.000000000000000000, 1.047445008332813989E-14 ) ) ;
#28579=CARTESIAN_POINT ( 'NONE',  ( -117.8738102209308352, 83.38952084682854604, 12.69999999999959428 ) ) ;
#28581=CYLINDRICAL_SURFACE ( 'NONE', #16888, 12.70000000000000107 ) ;
#28589=EDGE_CURVE ( 'NONE', #23091, #27806, #47854, .T. ) ;
#28602=CARTESIAN_POINT ( 'NONE',  ( 84.41404664249431278, 95.23005795263748041, -83.24642779537427373 ) ) ;
#28623=VECTOR ( 'NONE', #42574, 1000.000000000000000 ) ;
#28633=CARTESIAN_POINT ( 'NONE',  ( -4.100932966941606139, 70.52316614063619227, -130.4921811224707824 ) ) ;
#28640=DIRECTION ( 'NONE',  ( 0.000000000000000000, 1.000000000000000000, 0.000000000000000000 ) ) ;
#28641=VERTEX_POINT ( 'NONE', #76930 ) ;
#28645=ORIENTED_EDGE ( 'NONE', *, *, #33602, .F. ) ;
#28656=CARTESIAN_POINT ( 'NONE',  ( 94.61736061587667734, 70.27756284692564748, -89.95878776288191148 ) ) ;
#28673=AXIS2_PLACEMENT_3D ( 'NONE', #7228, #15834, #76712 ) ;
#28676=LINE ( 'NONE', #972, #41870 ) ;
#28689=DIRECTION ( 'NONE',  ( 0.000000000000000000, -1.000000000000000000, 0.000000000000000000 ) ) ;
#28690=CARTESIAN_POINT ( 'NONE',  ( -86.67141577317396184, 72.45841406287408404, 97.63922045723946042 ) ) ;
#28705=DIRECTION ( 'NONE',  ( 0.4999999999999986122, 0.000000000000000000, 0.8660254037844394848 ) ) ;
#28727=DIRECTION ( 'NONE',  ( 0.000000000000000000, 1.000000000000000000, 0.000000000000000000 ) ) ;
#28730=DIRECTION ( 'NONE',  ( -1.000000000000000000, 0.000000000000000000, 0.000000000000000000 ) ) ;
#28743=CARTESIAN_POINT ( 'NONE',  ( 0.000000000000000000, 61.59999999999999432, 118.5560000000000116 ) ) ;
#28768=EDGE_CURVE ( 'NONE', #57023, #32260, #71471, .T. ) ;
#28794=DIRECTION ( 'NONE',  ( 0.000000000000000000, 0.000000000000000000, 1.000000000000000000 ) ) ;
#28806=CARTESIAN_POINT ( 'NONE',  ( -92.32962665258560264, 82.54999999999999716, 74.36911441044701121 ) ) ;
#28814=AXIS2_PLACEMENT_3D ( 'NONE', #71409, #9173, #36436 ) ;
#28828=VECTOR ( 'NONE', #2453, 1000.000000000000000 ) ;
#28855=ORIENTED_EDGE ( 'NONE', *, *, #84995, .F. ) ;
#28866=CARTESIAN_POINT ( 'NONE',  ( 130.4924667154230065, 70.52006616879376111, 4.092011266638223788 ) ) ;
#28867=ORIENTED_EDGE ( 'NONE', *, *, #16766, .F. ) ;
#28882=DIRECTION ( 'NONE',  ( 1.000000000000000000, 0.000000000000000000, 1.047444401652940007E-14 ) ) ;
#28888=CARTESIAN_POINT ( 'NONE',  ( 1.088711004441995877E-14, 101.5999999999999943, -88.90000000000000568 ) ) ;
#28906=FACE_OUTER_BOUND ( 'NONE', #66031, .T. ) ;
#28917=CARTESIAN_POINT ( 'NONE',  ( -71.77848634863029531, 120.6499999999999915, -77.39114642430038771 ) ) ;
#28926=DIRECTION ( 'NONE',  ( 0.000000000000000000, -1.000000000000000000, 0.000000000000000000 ) ) ;
#28930=DIRECTION ( 'NONE',  ( 0.7071067811865460184, 0.000000000000000000, 0.7071067811865489050 ) ) ;
#28931=CARTESIAN_POINT ( 'NONE',  ( -7.205548786489490269E-13, 127.0000000000000000, 103.1875000000000000 ) ) ;
#28939=EDGE_CURVE ( 'NONE', #55858, #35298, #27210, .T. ) ;
#28941=VECTOR ( 'NONE', #57336, 1000.000000000000114 ) ;
#28954=CARTESIAN_POINT ( 'NONE',  ( -12.29197255332129401, 85.84955738763289901, 117.9171711396470386 ) ) ;
#28958=VERTEX_POINT ( 'NONE', #68556 ) ;
#28967=CARTESIAN_POINT ( 'NONE',  ( 12.70000000000000107, 82.54999999999999716, -117.8738102209307641 ) ) ;
#28977=ORIENTED_EDGE ( 'NONE', *, *, #83033, .F. ) ;
#28978=DIRECTION ( 'NONE',  ( 1.000000000000000000, 0.000000000000000000, 0.000000000000000000 ) ) ;
#28988=ADVANCED_FACE ( 'NONE', ( #19959 ), #26755, .F. ) ;
#28999=ORIENTED_EDGE ( 'NONE', *, *, #2750, .T. ) ;
#29014=LINE ( 'NONE', #14942, #71410 ) ;
#29016=FACE_OUTER_BOUND ( 'NONE', #17575, .T. ) ;
#29019=AXIS2_PLACEMENT_3D ( 'NONE', #74755, #3592, #40219 ) ;
#29032=DIRECTION ( 'NONE',  ( 0.000000000000000000, -1.000000000000000000, 0.000000000000000000 ) ) ;
#29040=CARTESIAN_POINT ( 'NONE',  ( -78.17042387453707875, 92.64232203292145584, 89.13693605261745745 ) ) ;
#29046=CARTESIAN_POINT ( 'NONE',  ( 84.43201024598467086, 69.85063172184842983, -83.23139715273229911 ) ) ;
#29050=DIRECTION ( 'NONE',  ( -0.7071067811865436870, 0.000000000000000000, -0.7071067811865514585 ) ) ;
#29062=CARTESIAN_POINT ( 'NONE',  ( 80.31773373136907423, 94.30044247306076954, -87.20679752240577898 ) ) ;
#29096=CARTESIAN_POINT ( 'NONE',  ( 0.000000000000000000, 127.0000000000000000, -103.1875000000000000 ) ) ;
#29115=CARTESIAN_POINT ( 'NONE',  ( 83.22858459372966422, 79.26455342200334542, -100.5877059554736093 ) ) ;
#29116=CARTESIAN_POINT ( 'NONE',  ( 100.8961411191535973, 120.6499999999999915, -3.968749999999580336 ) ) ;
#29128=DIRECTION ( 'NONE',  ( 0.000000000000000000, 1.000000000000000000, 0.000000000000000000 ) ) ;
#29133=LINE ( 'NONE', #49547, #57844 ) ;
#29135=AXIS2_PLACEMENT_3D ( 'NONE', #60671, #4832, #33873 ) ;
#29154=VECTOR ( 'NONE', #41388, 1000.000000000000000 ) ;
#29161=EDGE_LOOP ( 'NONE', ( #60070, #33429 ) ) ;
#29162=CARTESIAN_POINT ( 'NONE',  ( -82.96136257730057650, 80.89704698943971550, -100.8082743238004610 ) ) ;
#29163=CARTESIAN_POINT ( 'NONE',  ( -88.20392011030175183, 93.55466788070658879, -79.21949419058860542 ) ) ;
#29166=AXIS2_PLACEMENT_3D ( 'NONE', #7825, #14196, #13746 ) ;
#29183=EDGE_CURVE ( 'NONE', #9320, #83315, #29014, .T. ) ;
#29190=VERTEX_POINT ( 'NONE', #78522 ) ;
#29201=AXIS2_PLACEMENT_3D ( 'NONE', #67279, #32763, #30648 ) ;
#29203=CARTESIAN_POINT ( 'NONE',  ( 0.000000000000000000, 117.4749999999999943, -95.25000000000000000 ) ) ;
#29226=CARTESIAN_POINT ( 'NONE',  ( -12.67977336836081825, 83.37982733273464930, 129.9388093972407034 ) ) ;
#29236=ADVANCED_FACE ( 'NONE', ( #85342 ), #78072, .F. ) ;
#29276=CARTESIAN_POINT ( 'NONE',  ( -99.17062120112652224, 90.28418055714726620, -84.91247172076052152 ) ) ;
#29285=EDGE_CURVE ( 'NONE', #66793, #64886, #14665, .T. ) ;
#29292=PLANE ( 'NONE',  #82524 ) ;
#29299=LINE ( 'NONE', #71534, #26086 ) ;
#29308=VERTEX_POINT ( 'NONE', #87551 ) ;
#29319=CARTESIAN_POINT ( 'NONE',  ( -130.3267157422428966, 72.47310549519059464, -7.740869983443031010 ) ) ;
#29320=ORIENTED_EDGE ( 'NONE', *, *, #14255, .T. ) ;
#29321=AXIS2_PLACEMENT_3D ( 'NONE', #26578, #40195, #18416 ) ;
#29322=EDGE_CURVE ( 'NONE', #10974, #18138, #127, .T. ) ;
#29359=ORIENTED_EDGE ( 'NONE', *, *, #2442, .T. ) ;
#29372=ORIENTED_EDGE ( 'NONE', *, *, #61802, .T. ) ;
#29380=CARTESIAN_POINT ( 'NONE',  ( 88.25669247804529505, 93.94566094357735153, 96.20686424029969430 ) ) ;
#29437=EDGE_LOOP ( 'NONE', ( #75649, #42301, #41755, #33537 ) ) ;
#29444=VERTEX_POINT ( 'NONE', #33022 ) ;
#29471=EDGE_CURVE ( 'NONE', #27150, #14550, #59561, .T. ) ;
#29480=VERTEX_POINT ( 'NONE', #19849 ) ;
#29483=ORIENTED_EDGE ( 'NONE', *, *, #50914, .F. ) ;
#29485=CARTESIAN_POINT ( 'NONE',  ( -80.88915705228852460, 94.58006533271586136, 86.67541640318147245 ) ) ;
#29513=ORIENTED_EDGE ( 'NONE', *, *, #89818, .F. ) ;
#29522=PLANE ( 'NONE',  #50654 ) ;
#29524=ADVANCED_FACE ( 'NONE', ( #20310 ), #41169, .T. ) ;
#29555=AXIS2_PLACEMENT_3D ( 'NONE', #6485, #21016, #33748 ) ;
#29597=VECTOR ( 'NONE', #50242, 1000.000000000000000 ) ;
#29599=DIRECTION ( 'NONE',  ( 0.000000000000000000, -1.000000000000000000, 0.000000000000000000 ) ) ;
#29603=ORIENTED_EDGE ( 'NONE', *, *, #64146, .F. ) ;
#29607=CARTESIAN_POINT ( 'NONE',  ( -84.99816483510880971, 95.16897323824362331, -82.65294504194714875 ) ) ;
#29629=VERTEX_POINT ( 'NONE', #41631 ) ;
#29632=ORIENTED_EDGE ( 'NONE', *, *, #79860, .F. ) ;
#29640=CARTESIAN_POINT ( 'NONE',  ( -11.00676631360785862, 76.20068480870281746, 130.0913480697105342 ) ) ;
#29647=FACE_OUTER_BOUND ( 'NONE', #69260, .T. ) ;
#29655=AXIS2_PLACEMENT_3D ( 'NONE', #62488, #48838, #27965 ) ;
#29692=EDGE_CURVE ( 'NONE', #45031, #12282, #14862, .T. ) ;
#29699=( GEOMETRIC_REPRESENTATION_CONTEXT ( 3 ) GLOBAL_UNCERTAINTY_ASSIGNED_CONTEXT ( ( #81741 ) ) GLOBAL_UNIT_ASSIGNED_CONTEXT ( ( #80927, #68179, #74087 ) ) REPRESENTATION_CONTEXT ( 'NONE', 'WORKASPACE' ) );
#29723=B_SPLINE_CURVE_WITH_KNOTS ( 'NONE', 3,
 ( #32013, #79307, #31123, #71595, #23454, #17065, #78862, #45620, #72033, #9803, #9356, #73354, #37513, #65212, #37063, #51993, #86560, #64767, #2988, #72478, #24325, #38832, #37948, #79752, #2552 ),
 .UNSPECIFIED., .F., .F.,
 ( 4, 2, 2, 1, 2, 2, 2, 2, 2, 2, 2, 2, 4 ),
 ( 0.03972946622853321813, 0.04221318292723494348, 0.04345504127658580962, 0.04469689962593667576, 0.04593875797528754190, 0.04718061632463840110, 0.04966433302334011257, 0.05090619137269095096, 0.05214804972204178934, 0.05463176642074347306, 0.05587362477009431838, 0.05711548311944515677, 0.05959919981814688211 ),
 .UNSPECIFIED. ) ;
#29734=AXIS2_PLACEMENT_3D ( 'NONE', #25520, #46390, #32321 ) ;
#29751=ORIENTED_EDGE ( 'NONE', *, *, #77000, .F. ) ;
#29764=CARTESIAN_POINT ( 'NONE',  ( 31.75000000000000000, 124.5870000000000033, -3.174999999999999822 ) ) ;
#29766=ORIENTED_EDGE ( 'NONE', *, *, #28589, .F. ) ;
#29772=VECTOR ( 'NONE', #81632, 1000.000000000000114 ) ;
#29782=CARTESIAN_POINT ( 'NONE',  ( 3.968750000000000000, 120.6499999999999915, -105.4788588808464027 ) ) ;
#29795=CARTESIAN_POINT ( 'NONE',  ( -74.15067561874319324, 120.6499999999999915, 68.53801554307369770 ) ) ;
#29797=CARTESIAN_POINT ( 'NONE',  ( -72.96458098368751166, 127.0000000000000000, 65.82083098368619289 ) ) ;
#29813=DIRECTION ( 'NONE',  ( 0.000000000000000000, 1.000000000000000000, 0.000000000000000000 ) ) ;
#29820=EDGE_CURVE ( 'NONE', #59781, #35831, #44431, .T. ) ;
#29826=CARTESIAN_POINT ( 'NONE',  ( 91.73195104381078124, 95.23006786499112764, 92.89936586972081045 ) ) ;
#29847=EDGE_CURVE ( 'NONE', #13859, #80299, #62561, .T. ) ;
#29853=CONICAL_SURFACE ( 'NONE', #31254, 190.5000000000000000, 0.7853981633974300713 ) ;
#29871=FACE_OUTER_BOUND ( 'NONE', #48349, .T. ) ;
#29917=CARTESIAN_POINT ( 'NONE',  ( 86.67734222162479796, 70.52090377575433422, 80.88709205069480390 ) ) ;
#29933=DIRECTION ( 'NONE',  ( 1.000000000000000000, 0.000000000000000000, 0.000000000000000000 ) ) ;
#29941=CARTESIAN_POINT ( 'NONE',  ( -76.39920031718024518, 90.28416741362498499, 90.65736737572441939 ) ) ;
#29956=DIRECTION ( 'NONE',  ( 0.000000000000000000, 0.000000000000000000, -1.000000000000000000 ) ) ;
#29958=CARTESIAN_POINT ( 'NONE',  ( 69.72411017812960665, 127.0000000000000000, 69.72411017813040246 ) ) ;
#29968=LINE ( 'NONE', #7730, #8673 ) ;
#29987=FACE_OUTER_BOUND ( 'NONE', #18605, .T. ) ;
#30000=ORIENTED_EDGE ( 'NONE', *, *, #78325, .F. ) ;
#30025=CARTESIAN_POINT ( 'NONE',  ( -72.96458098368600531, 127.0000000000000000, -80.90208098368781009 ) ) ;
#30033=CARTESIAN_POINT ( 'NONE',  ( -3.968750000000754508, 120.6499999999999915, 100.8961411191535973 ) ) ;
#30043=AXIS2_PLACEMENT_3D ( 'NONE', #29782, #63400, #1181 ) ;
#30044=DIRECTION ( 'NONE',  ( -0.000000000000000000, -0.000000000000000000, 1.000000000000000000 ) ) ;
#30050=DIRECTION ( 'NONE',  ( 0.000000000000000000, -1.000000000000000000, 0.000000000000000000 ) ) ;
#30112=CARTESIAN_POINT ( 'NONE',  ( 77.39114642429899504, 120.6499999999999915, 71.77848634863160271 ) ) ;
#30123=CIRCLE ( 'NONE', #18503, 34.13125000000000142 ) ;
#30146=ORIENTED_EDGE ( 'NONE', *, *, #13627, .T. ) ;
#30147=VECTOR ( 'NONE', #70416, 1000.000000000000000 ) ;
#30156=CARTESIAN_POINT ( 'NONE',  ( 0.000000000000000000, 127.0000000000000000, -190.5000000000000000 ) ) ;
#30169=CARTESIAN_POINT ( 'NONE',  ( 68.53801554307389665, 120.6499999999999915, 74.15067561874289481 ) ) ;
#30176=AXIS2_PLACEMENT_3D ( 'NONE', #42096, #7596, #49805 ) ;
#30183=AXIS2_PLACEMENT_3D ( 'NONE', #58562, #80379, #60346 ) ;
#30189=CARTESIAN_POINT ( 'NONE',  ( -72.96458098368600531, 127.0000000000000000, -65.82083098368781293 ) ) ;
#30190=ORIENTED_EDGE ( 'NONE', *, *, #44023, .T. ) ;
#30196=VERTEX_POINT ( 'NONE', #22907 ) ;
#30197=AXIS2_PLACEMENT_3D ( 'NONE', #35888, #70879, #57672 ) ;
#30206=DIRECTION ( 'NONE',  ( 0.000000000000000000, 1.000000000000000000, 0.000000000000000000 ) ) ;
#30213=EDGE_CURVE ( 'NONE', #3990, #16856, #78772, .T. ) ;
#30232=ORIENTED_EDGE ( 'NONE', *, *, #13633, .T. ) ;
#30237=CARTESIAN_POINT ( 'NONE',  ( -67.35192090801770348, 120.6499999999999915, -78.57724105935601244 ) ) ;
#30255=CARTESIAN_POINT ( 'NONE',  ( -71.77848634863029531, 120.6499999999999915, -77.39114642430038771 ) ) ;
#30282=ORIENTED_EDGE ( 'NONE', *, *, #67433, .T. ) ;
#30285=ORIENTED_EDGE ( 'NONE', *, *, #40061, .F. ) ;
#30288=VECTOR ( 'NONE', #15596, 1000.000000000000000 ) ;
#30289=LINE ( 'NONE', #78461, #3212 ) ;
#30317=AXIS2_PLACEMENT_3D ( 'NONE', #65302, #18031, #86643 ) ;
#30330=CARTESIAN_POINT ( 'NONE',  ( 0.000000000000000000, 127.0000000000000000, -110.3312500000000114 ) ) ;
#30332=FACE_OUTER_BOUND ( 'NONE', #54845, .T. ) ;
#30336=CARTESIAN_POINT ( 'NONE',  ( 31.75000000000000000, 124.5870000000000033, 3.174999999999999822 ) ) ;
#30346=CARTESIAN_POINT ( 'NONE',  ( 83.22961976134631357, 79.25971567868505474, 100.5868491334651225 ) ) ;
#30350=LINE ( 'NONE', #23109, #33630 ) ;
#30362=CARTESIAN_POINT ( 'NONE',  ( 87.20837788851326877, 70.80054595721396993, 80.31601367611443720 ) ) ;
#30381=EDGE_CURVE ( 'NONE', #5511, #1241, #20436, .T. ) ;
#30401=CYLINDRICAL_SURFACE ( 'NONE', #1895, 12.70000000000000107 ) ;
#30435=EDGE_CURVE ( 'NONE', #34288, #48773, #7254, .T. ) ;
#30437=DIRECTION ( 'NONE',  ( 0.000000000000000000, -1.000000000000000000, 0.000000000000000000 ) ) ;
#30448=ADVANCED_FACE ( 'NONE', ( #9052 ), #63094, .F. ) ;
#30455=ORIENTED_EDGE ( 'NONE', *, *, #769, .F. ) ;
#30457=LINE ( 'NONE', #58155, #56462 ) ;
#30467=EDGE_CURVE ( 'NONE', #57201, #70164, #1018, .T. ) ;
#30474=EDGE_LOOP ( 'NONE', ( #35998, #77619, #38485, #84830 ) ) ;
#30486=ORIENTED_EDGE ( 'NONE', *, *, #55213, .F. ) ;
#30492=CARTESIAN_POINT ( 'NONE',  ( -100.8594679592212486, 82.96445444011520465, 82.89895571708262878 ) ) ;
#30512=EDGE_CURVE ( 'NONE', #64107, #13859, #45756, .T. ) ;
#30535=EDGE_CURVE ( 'NONE', #8142, #32905, #18071, .T. ) ;
#30573=DIRECTION ( 'NONE',  ( -0.2588190451025281225, 0.000000000000000000, 0.9659258262890663138 ) ) ;
#30589=ORIENTED_EDGE ( 'NONE', *, *, #81091, .T. ) ;
#30600=CARTESIAN_POINT ( 'NONE',  ( 118.2598914205052552, 72.98405218941671535, -8.394510633989694881 ) ) ;
#30603=PLANE ( 'NONE',  #6691 ) ;
#30607=ORIENTED_EDGE ( 'NONE', *, *, #86456, .F. ) ;
#30611=DIRECTION ( 'NONE',  ( 0.000000000000000000, -1.000000000000000000, 0.000000000000000000 ) ) ;
#30619=EDGE_CURVE ( 'NONE', #87954, #43612, #79438, .T. ) ;
#30623=CARTESIAN_POINT ( 'NONE',  ( -2.884119045937113768, 70.17489121805367347, 118.5216098345816960 ) ) ;
#30625=EDGE_CURVE ( 'NONE', #74189, #89290, #14801, .T. ) ;
#30631=EDGE_CURVE ( 'NONE', #43486, #52485, #3119, .T. ) ;
#30642=AXIS2_PLACEMENT_3D ( 'NONE', #79075, #3215, #78193 ) ;
#30648=DIRECTION ( 'NONE',  ( 0.000000000000000000, 0.000000000000000000, 1.000000000000000000 ) ) ;
#30649=CARTESIAN_POINT ( 'NONE',  ( -129.9447564289581578, 80.89704698943971550, -12.61967231918767496 ) ) ;
#30652=CIRCLE ( 'NONE', #21917, 7.937500000000000000 ) ;
#30657=CARTESIAN_POINT ( 'NONE',  ( 72.96458098368701428, 127.0000000000000000, -72.96458098368670164 ) ) ;
#30665=CARTESIAN_POINT ( 'NONE',  ( -3.175000000000109956, 104.3431970271541900, 31.75000000000000000 ) ) ;
#30694=CARTESIAN_POINT ( 'NONE',  ( 0.000000000000000000, 92.07499999999998863, 0.000000000000000000 ) ) ;
#30714=CARTESIAN_POINT ( 'NONE',  ( 12.70000000000000107, 83.38939070830900846, 129.9368274816650626 ) ) ;
#30748=CARTESIAN_POINT ( 'NONE',  ( -82.89895571708295563, 82.54999999999999716, 100.8594679592209644 ) ) ;
#30760=EDGE_LOOP ( 'NONE', ( #75804, #67720, #55607, #51349 ) ) ;
#30766=FACE_OUTER_BOUND ( 'NONE', #47799, .T. ) ;
#30771=DIRECTION ( 'NONE',  ( 0.000000000000000000, -1.000000000000000000, 0.000000000000000000 ) ) ;
#30799=CARTESIAN_POINT ( 'NONE',  ( 76.38829385798568694, 74.80137413886473041, 90.66736180499722764 ) ) ;
#30821=DIRECTION ( 'NONE',  ( 0.9659258262890704216, 0.000000000000000000, -0.2588190451025129124 ) ) ;
#30827=CARTESIAN_POINT ( 'NONE',  ( -6.802569982901797644E-16, 69.84999999999999432, -118.5560000000000116 ) ) ;
#30841=CARTESIAN_POINT ( 'NONE',  ( -7.196800215918080040E-13, 127.0000000000000000, 110.3312500000000114 ) ) ;
#30848=VERTEX_POINT ( 'NONE', #1685 ) ;
#30856=DIRECTION ( 'NONE',  ( -0.2588190451025206285, 0.000000000000000000, 0.9659258262890683122 ) ) ;
#30867=LINE ( 'NONE', #87175, #46179 ) ;
#30903=CARTESIAN_POINT ( 'NONE',  ( 71.77848634863140376, 127.0000000000000000, -77.39114642429929347 ) ) ;
#30917=LINE ( 'NONE', #67562, #41191 ) ;
#30927=VECTOR ( 'NONE', #44385, 1000.000000000000000 ) ;
#30930=CARTESIAN_POINT ( 'NONE',  ( -91.72735010416610635, 95.24968527363476767, 92.90667244829751326 ) ) ;
#30945=CARTESIAN_POINT ( 'NONE',  ( -100.8961411191535973, 127.0000000000000000, 3.968749999998880451 ) ) ;
#30977=CARTESIAN_POINT ( 'NONE',  ( -11.75210537873753402, 77.68270844259760111, 130.0262747911924635 ) ) ;
#30991=VECTOR ( 'NONE', #80821, 1000.000000000000000 ) ;
#31018=DIRECTION ( 'NONE',  ( 0.000000000000000000, 0.000000000000000000, -1.000000000000000000 ) ) ;
#31019=EDGE_CURVE ( 'NONE', #5511, #24458, #9031, .T. ) ;
#31083=CARTESIAN_POINT ( 'NONE',  ( -130.2664984484596005, 73.28356282573680858, -8.694507028640293456 ) ) ;
#31101=PLANE ( 'NONE',  #43054 ) ;
#31123=CARTESIAN_POINT ( 'NONE',  ( -1.653891986036712280, 95.16955141394549855, -130.5480982590283645 ) ) ;
#31143=CARTESIAN_POINT ( 'NONE',  ( 0.8398470015645936870, 69.84999999999999432, -130.5559999999999832 ) ) ;
#31147=AXIS2_PLACEMENT_3D ( 'NONE', #83217, #41400, #69129 ) ;
#31196=AXIS2_PLACEMENT_3D ( 'NONE', #43232, #17338, #65913 ) ;
#31233=CARTESIAN_POINT ( 'NONE',  ( 76.79083731950140645, 74.16215221268211621, 90.32738470895372984 ) ) ;
#31244=CARTESIAN_POINT ( 'NONE',  ( 118.5560163110023524, 95.25015226514366873, 0.4098827902177066274 ) ) ;
#31247=EDGE_CURVE ( 'NONE', #41448, #35668, #51081, .T. ) ;
#31254=AXIS2_PLACEMENT_3D ( 'NONE', #59050, #87675, #66321 ) ;
#31262=VERTEX_POINT ( 'NONE', #67917 ) ;
#31270=CARTESIAN_POINT ( 'NONE',  ( 31.75000000000000000, 104.3431970271542042, -3.174999999999999822 ) ) ;
#31277=CARTESIAN_POINT ( 'NONE',  ( 0.000000000000000000, 127.0000000000000000, -188.9759999999999991 ) ) ;
#31297=EDGE_CURVE ( 'NONE', #71309, #8142, #88381, .T. ) ;
#31306=FACE_OUTER_BOUND ( 'NONE', #37325, .T. ) ;
#31312=ORIENTED_EDGE ( 'NONE', *, *, #24127, .T. ) ;
#31347=CARTESIAN_POINT ( 'NONE',  ( -71.77848634863029531, 120.6499999999999915, -77.39114642430038771 ) ) ;
#31380=CARTESIAN_POINT ( 'NONE',  ( 72.96458098368650269, 127.0000000000000000, 65.02708098368729850 ) ) ;
#31391=EDGE_LOOP ( 'NONE', ( #19958, #37256, #20098, #47489 ) ) ;
#31407=EDGE_CURVE ( 'NONE', #28006, #27158, #75801, .T. ) ;
#31415=ADVANCED_FACE ( 'NONE', ( #218 ), #48338, .F. ) ;
#31421=LINE ( 'NONE', #25065, #53341 ) ;
#31424=DIRECTION ( 'NONE',  ( 0.2588190451025215166, 0.000000000000000000, -0.9659258262890680902 ) ) ;
#31437=DIRECTION ( 'NONE',  ( 0.000000000000000000, 0.000000000000000000, 1.000000000000000000 ) ) ;
#31442=DIRECTION ( 'NONE',  ( 0.000000000000000000, 1.000000000000000000, 0.000000000000000000 ) ) ;
#31449=FACE_OUTER_BOUND ( 'NONE', #11006, .T. ) ;
#31461=FACE_BOUND ( 'NONE', #4623, .T. ) ;
#31474=CARTESIAN_POINT ( 'NONE',  ( 117.8738102209305936, 81.72118090664554302, 12.70000000000123030 ) ) ;
#31509=DIRECTION ( 'NONE',  ( -0.000000000000000000, 1.000000000000000000, 0.000000000000000000 ) ) ;
#31525=AXIS2_PLACEMENT_3D ( 'NONE', #7194, #34884, #42138 ) ;
#31551=ORIENTED_EDGE ( 'NONE', *, *, #65643, .F. ) ;
#31561=CARTESIAN_POINT ( 'NONE',  ( -2.684158038187649039E-15, 69.84999999999999432, 130.5560000000000116 ) ) ;
#31567=DIRECTION ( 'NONE',  ( -1.000000000000000000, 0.000000000000000000, -1.047445008332813989E-14 ) ) ;
#31585=CARTESIAN_POINT ( 'NONE',  ( 12.37530111100094743, 79.66613297688917328, -129.9681797613511947 ) ) ;
#31594=AXIS2_PLACEMENT_3D ( 'NONE', #29096, #9106, #50415 ) ;
#31595=CARTESIAN_POINT ( 'NONE',  ( 9.270409258063832425, 91.24028187096000408, 130.2267823906806541 ) ) ;
#31619=EDGE_LOOP ( 'NONE', ( #67982, #61575, #72802, #31931 ) ) ;
#31641=EDGE_CURVE ( 'NONE', #60807, #11982, #52545, .T. ) ;
#31655=ADVANCED_FACE ( 'NONE', ( #66453 ), #73727, .F. ) ;
#31681=CARTESIAN_POINT ( 'NONE',  ( 0.000000000000000000, 92.07499999999998863, 0.000000000000000000 ) ) ;
#31697=CARTESIAN_POINT ( 'NONE',  ( 117.8738102209308920, 82.54999999999999716, -12.69999999999876827 ) ) ;
#31724=DIRECTION ( 'NONE',  ( 0.000000000000000000, 0.000000000000000000, 1.000000000000000000 ) ) ;
#31732=CARTESIAN_POINT ( 'NONE',  ( -118.3040894999502655, 72.45860812971085352, 7.755682336160878876 ) ) ;
#31737=FACE_OUTER_BOUND ( 'NONE', #70983, .T. ) ;
#31773=ORIENTED_EDGE ( 'NONE', *, *, #69735, .T. ) ;
#31777=CYLINDRICAL_SURFACE ( 'NONE', #7576, 42.54500000000000171 ) ;
#31790=FACE_OUTER_BOUND ( 'NONE', #72584, .T. ) ;
#31795=ORIENTED_EDGE ( 'NONE', *, *, #3565, .F. ) ;
#31814=CARTESIAN_POINT ( 'NONE',  ( -82.89895571708295563, 82.54999999999999716, 100.8594679592209644 ) ) ;
#31815=FACE_BOUND ( 'NONE', #7356, .T. ) ;
#31819=CARTESIAN_POINT ( 'NONE',  ( 0.000000000000000000, 124.5870000000000033, 0.000000000000000000 ) ) ;
#31832=AXIS2_PLACEMENT_3D ( 'NONE', #83723, #47610, #54860 ) ;
#31851=AXIS2_PLACEMENT_3D ( 'NONE', #64488, #50390, #56760 ) ;
#31868=CARTESIAN_POINT ( 'NONE',  ( -89.13771950014300671, 72.45860812971082510, -78.16952835488712026 ) ) ;
#31897=VECTOR ( 'NONE', #586, 1000.000000000000114 ) ;
#31898=ORIENTED_EDGE ( 'NONE', *, *, #55622, .F. ) ;
#31907=DIRECTION ( 'NONE',  ( 0.000000000000000000, -1.000000000000000000, 0.000000000000000000 ) ) ;
#31912=CARTESIAN_POINT ( 'NONE',  ( -83.22858459372896789, 79.26455342200334542, 100.5877059554742061 ) ) ;
#31925=CARTESIAN_POINT ( 'NONE',  ( 118.0439878494275945, 76.20320268897036442, 11.00820894928519245 ) ) ;
#31931=ORIENTED_EDGE ( 'NONE', *, *, #76554, .F. ) ;
#31949=VECTOR ( 'NONE', #60298, 999.9999999999998863 ) ;
#32013=CARTESIAN_POINT ( 'NONE',  ( 1.598849865763559337E-14, 95.25000000000000000, -130.5560000000000116 ) ) ;
#32023=ORIENTED_EDGE ( 'NONE', *, *, #54081, .F. ) ;
#32049=EDGE_CURVE ( 'NONE', #78413, #7174, #76722, .T. ) ;
#32051=DIRECTION ( 'NONE',  ( 0.000000000000000000, -1.000000000000000000, 0.000000000000000000 ) ) ;
#32084=EDGE_CURVE ( 'NONE', #3056, #6765, #83997, .T. ) ;
#32101=CYLINDRICAL_SURFACE ( 'NONE', #18151, 7.937500000000000000 ) ;
#32102=DIRECTION ( 'NONE',  ( -0.5000000000000061062, 0.000000000000000000, 0.8660254037844351549 ) ) ;
#32105=ADVANCED_FACE ( 'NONE', ( #22812 ), #45005, .T. ) ;
#32112=CARTESIAN_POINT ( 'NONE',  ( 10.78734560828563183, 89.26522093196125240, -130.1097824653510031 ) ) ;
#32151=CARTESIAN_POINT ( 'NONE',  ( -68.91674821478409285, 82.54999999999999716, -68.91674821478481761 ) ) ;
#32173=CARTESIAN_POINT ( 'NONE',  ( 3.174999999999889688, 111.1250000000000000, 31.75000000000000000 ) ) ;
#32176=FACE_OUTER_BOUND ( 'NONE', #31391, .T. ) ;
#32211=DIRECTION ( 'NONE',  ( -0.9659258262890690894, 0.000000000000000000, -0.2588190451025180749 ) ) ;
#32215=CARTESIAN_POINT ( 'NONE',  ( -130.1467854596290010, 89.94765885072629885, 10.33135106516698265 ) ) ;
#32219=CIRCLE ( 'NONE', #16293, 190.5000000000000000 ) ;
#32220=EDGE_CURVE ( 'NONE', #39347, #12421, #41943, .T. ) ;
#32231=VECTOR ( 'NONE', #62728, 1000.000000000000000 ) ;
#32236=VERTEX_POINT ( 'NONE', #87260 ) ;
#32257=FACE_OUTER_BOUND ( 'NONE', #60411, .T. ) ;
#32260=VERTEX_POINT ( 'NONE', #3688 ) ;
#32289=CARTESIAN_POINT ( 'NONE',  ( 130.5247076678899703, 94.92443974548208985, -2.887521757539373457 ) ) ;
#32306=CARTESIAN_POINT ( 'NONE',  ( -88.44575049335551853, 71.76236341257998674, -78.94931995840768479 ) ) ;
#32312=LINE ( 'NONE', #53181, #9818 ) ;
#32321=DIRECTION ( 'NONE',  ( 0.000000000000000000, 0.000000000000000000, 1.000000000000000000 ) ) ;
#32361=CARTESIAN_POINT ( 'NONE',  ( 117.8738102209306362, 82.54999999999999716, 12.70000000000123386 ) ) ;
#32372=CARTESIAN_POINT ( 'NONE',  ( -96.20681132576102357, 71.15434825076368952, -88.25674559704586386 ) ) ;
#32384=CARTESIAN_POINT ( 'NONE',  ( -1.665763066381118485, 69.93250922127340630, 118.5470808886261125 ) ) ;
#32463=CARTESIAN_POINT ( 'NONE',  ( -7.196800215918080040E-13, 117.4749999999999943, 110.3312500000000114 ) ) ;
#32477=CARTESIAN_POINT ( 'NONE',  ( 80.89343850130745750, 94.60304557064716846, 86.67392531623393381 ) ) ;
#32498=CARTESIAN_POINT ( 'NONE',  ( 100.8594679592218171, 82.54999999999999716, -82.89895571708191824 ) ) ;
#32505=ORIENTED_EDGE ( 'NONE', *, *, #39832, .F. ) ;
#32516=ORIENTED_EDGE ( 'NONE', *, *, #71708, .F. ) ;
#32522=ORIENTED_EDGE ( 'NONE', *, *, #88901, .T. ) ;
#32544=ADVANCED_FACE ( 'NONE', ( #87044 ), #22703, .T. ) ;
#32547=ORIENTED_EDGE ( 'NONE', *, *, #51810, .T. ) ;
#32553=CARTESIAN_POINT ( 'NONE',  ( 8.387211759491236762, 92.12327290876406494, -130.2876699444761073 ) ) ;
#32557=ADVANCED_FACE ( 'NONE', ( #43107, #63576, #80233, #17981 ), #73395, .T. ) ;
#32576=VERTEX_POINT ( 'NONE', #64030 ) ;
#32599=CARTESIAN_POINT ( 'NONE',  ( -3.968750000000754508, 127.0000000000000000, 100.8961411191535973 ) ) ;
#32601=LINE ( 'NONE', #73495, #66822 ) ;
#32605=EDGE_LOOP ( 'NONE', ( #22541, #25489 ) ) ;
#32614=VERTEX_POINT ( 'NONE', #32498 ) ;
#32668=CARTESIAN_POINT ( 'NONE',  ( -130.4667782423797746, 94.30053025434479252, 4.871090630222163043 ) ) ;
#32679=ORIENTED_EDGE ( 'NONE', *, *, #27667, .T. ) ;
#32688=CARTESIAN_POINT ( 'NONE',  ( -33.98325472291465132, 124.5870000000000033, 3.174999999999764899 ) ) ;
#32710=CARTESIAN_POINT ( 'NONE',  ( -84.19383299529339126, 88.91243380484083048, 99.78216974382904425 ) ) ;
#32728=AXIS2_PLACEMENT_3D ( 'NONE', #88530, #4506, #45368 ) ;
#32745=DIRECTION ( 'NONE',  ( 0.000000000000000000, -1.000000000000000000, 0.000000000000000000 ) ) ;
#32747=FILL_AREA_STYLE ('',( #39112 ) ) ;
#32758=CIRCLE ( 'NONE', #83545, 130.5560000000000116 ) ;
#32763=DIRECTION ( 'NONE',  ( 0.000000000000000000, 1.000000000000000000, 0.000000000000000000 ) ) ;
#32788=ORIENTED_EDGE ( 'NONE', *, *, #51307, .T. ) ;
#32821=EDGE_CURVE ( 'NONE', #43994, #48000, #1592, .T. ) ;
#32824=LINE ( 'NONE', #68258, #59424 ) ;
#32868=VERTEX_POINT ( 'NONE', #56527 ) ;
#32892=CARTESIAN_POINT ( 'NONE',  ( -3.292096649336115011, 94.82294024675948663, -118.5109520256350208 ) ) ;
#32899=DIRECTION ( 'NONE',  ( 0.9659258262890688673, 0.000000000000000000, -0.2588190451025189631 ) ) ;
#32905=VERTEX_POINT ( 'NONE', #62896 ) ;
#32915=CARTESIAN_POINT ( 'NONE',  ( -76.20754074253656540, 75.15251084995277608, 90.81844170390348836 ) ) ;
#32944=EDGE_LOOP ( 'NONE', ( #36637, #72476 ) ) ;
#32975=EDGE_CURVE ( 'NONE', #6171, #61270, #56536, .T. ) ;
#33010=CARTESIAN_POINT ( 'NONE',  ( 11.57415360872102994, 87.79424630570801469, -130.0420457590603860 ) ) ;
#33012=DIRECTION ( 'NONE',  ( 3.386875084296745512E-15, 0.000000000000000000, -1.000000000000000000 ) ) ;
#33022=CARTESIAN_POINT ( 'NONE',  ( 0.000000000000000000, 101.5999999999999943, -98.14560000000000173 ) ) ;
#33024=LINE ( 'NONE', #47083, #67252 ) ;
#33034=ORIENTED_EDGE ( 'NONE', *, *, #24695, .F. ) ;
#33051=DIRECTION ( 'NONE',  ( -0.7071067811865437980, 0.000000000000000000, -0.7071067811865512365 ) ) ;
#33058=ORIENTED_EDGE ( 'NONE', *, *, #50811, .F. ) ;
#33076=CARTESIAN_POINT ( 'NONE',  ( -118.5469577077833065, 69.93366089391888352, -1.674277437722204720 ) ) ;
#33094=AXIS2_PLACEMENT_3D ( 'NONE', #52630, #80392, #11330 ) ;
#33098=DIRECTION ( 'NONE',  ( 0.000000000000000000, 1.000000000000000000, 0.000000000000000000 ) ) ;
#33122=CARTESIAN_POINT ( 'NONE',  ( -130.5540562089606738, 95.23006786499111342, -0.8254869398575555017 ) ) ;
#33134=CARTESIAN_POINT ( 'NONE',  ( 95.94886839522645516, 94.12569442554141119, -88.53717826876584240 ) ) ;
#33139=CARTESIAN_POINT ( 'NONE',  ( -6.720192613126054759, 71.76561204655834558, -118.3658933525135524 ) ) ;
#33142=AXIS2_PLACEMENT_3D ( 'NONE', #3254, #50486, #78232 ) ;
#33171=DIRECTION ( 'NONE',  ( 0.000000000000000000, 0.000000000000000000, -1.000000000000000000 ) ) ;
#33186=EDGE_CURVE ( 'NONE', #81111, #73627, #6059, .T. ) ;
#33202=CARTESIAN_POINT ( 'NONE',  ( 130.0906791124284894, 88.91243380484084469, -11.02261862230788303 ) ) ;
#33210=VERTEX_POINT ( 'NONE', #87378 ) ;
#33221=CARTESIAN_POINT ( 'NONE',  ( -92.12448541806607238, 79.66685870724428753, -74.62312585591620007 ) ) ;
#33248=CARTESIAN_POINT ( 'NONE',  ( 2.323620343766204915E-14, 101.5999999999999943, -188.9759999999999991 ) ) ;
#33266=ORIENTED_EDGE ( 'NONE', *, *, #59967, .T. ) ;
#33288=DIRECTION ( 'NONE',  ( 0.000000000000000000, 0.000000000000000000, 1.000000000000000000 ) ) ;
#33302=LINE ( 'NONE', #75083, #68711 ) ;
#33331=ORIENTED_EDGE ( 'NONE', *, *, #27531, .F. ) ;
#33362=VECTOR ( 'NONE', #6634, 1000.000000000000000 ) ;
#33373=ORIENTED_EDGE ( 'NONE', *, *, #51902, .T. ) ;
#33379=CARTESIAN_POINT ( 'NONE',  ( -33.98325472291465132, 124.5870000000000033, 3.174999999999764899 ) ) ;
#33385=CARTESIAN_POINT ( 'NONE',  ( 86.67541640318067664, 94.58006533271583294, 80.88915705228943409 ) ) ;
#33395=CARTESIAN_POINT ( 'NONE',  ( -88.25669247804601980, 93.94566094357733732, -96.20686424029906902 ) ) ;
#33414=FACE_OUTER_BOUND ( 'NONE', #23226, .T. ) ;
#33429=ORIENTED_EDGE ( 'NONE', *, *, #29471, .F. ) ;
#33461=DIRECTION ( 'NONE',  ( 0.000000000000000000, 0.000000000000000000, 1.000000000000000000 ) ) ;
#33466=CIRCLE ( 'NONE', #20375, 7.143750000000004263 ) ;
#33470=AXIS2_PLACEMENT_3D ( 'NONE', #77123, #71208, #14899 ) ;
#33483=FACE_BOUND ( 'NONE', #55145, .T. ) ;
#33484=ADVANCED_FACE ( 'NONE', ( #7386, #35076, #86380, #50500 ), #16893, .F. ) ;
#33493=VECTOR ( 'NONE', #15724, 1000.000000000000000 ) ;
#33502=CARTESIAN_POINT ( 'NONE',  ( -72.96458098368751166, 117.4749999999999943, 72.96458098368620426 ) ) ;
#33510=ORIENTED_EDGE ( 'NONE', *, *, #82758, .F. ) ;
#33532=CARTESIAN_POINT ( 'NONE',  ( -100.8594679592212344, 82.54999999999999716, 82.89895571708261457 ) ) ;
#33537=ORIENTED_EDGE ( 'NONE', *, *, #58715, .T. ) ;
#33555=DIRECTION ( 'NONE',  ( 0.7071067811865536790, 0.000000000000000000, -0.7071067811865414665 ) ) ;
#33560=CARTESIAN_POINT ( 'NONE',  ( -103.1875000000000000, 127.0000000000000000, -1.080832317973422076E-12 ) ) ;
#33564=PLANE ( 'NONE',  #8849 ) ;
#33565=CARTESIAN_POINT ( 'NONE',  ( -129.9777364973647025, 85.83513192049078100, 12.27484926615008476 ) ) ;
#33582=VECTOR ( 'NONE', #30821, 1000.000000000000114 ) ;
#33602=EDGE_CURVE ( 'NONE', #89451, #4210, #76146, .T. ) ;
#33604=ORIENTED_EDGE ( 'NONE', *, *, #15284, .T. ) ;
#33610=CARTESIAN_POINT ( 'NONE',  ( -117.8738102209307215, 82.96450994655481281, -12.70000000000041496 ) ) ;
#33615=FACE_OUTER_BOUND ( 'NONE', #71763, .T. ) ;
#33630=VECTOR ( 'NONE', #50779, 1000.000000000000000 ) ;
#33635=AXIS2_PLACEMENT_3D ( 'NONE', #17020, #10199, #40472 ) ;
#33643=CYLINDRICAL_SURFACE ( 'NONE', #40758, 5.041900000000001825 ) ;
#33655=AXIS2_PLACEMENT_3D ( 'NONE', #25719, #19808, #88860 ) ;
#33710=DIRECTION ( 'NONE',  ( 0.000000000000000000, -1.000000000000000000, 0.000000000000000000 ) ) ;
#33735=CARTESIAN_POINT ( 'NONE',  ( -100.8594679592206802, 82.54999999999999716, -82.89895571708333932 ) ) ;
#33746=CARTESIAN_POINT ( 'NONE',  ( -12.37524867428841091, 79.66590588004265783, 117.9083757119989428 ) ) ;
#33747=CARTESIAN_POINT ( 'NONE',  ( -98.60478223830740774, 120.6499999999999915, -1.074461880482445986E-12 ) ) ;
#33748=DIRECTION ( 'NONE',  ( 1.000000000000000000, 0.000000000000000000, 6.878358445406130340E-15 ) ) ;
#33757=ORIENTED_EDGE ( 'NONE', *, *, #40449, .T. ) ;
#33783=PLANE ( 'NONE',  #58689 ) ;
#33833=CARTESIAN_POINT ( 'NONE',  ( 83.24642779537398951, 95.23005795263748041, 84.41404664249461121 ) ) ;
#33851=CYLINDRICAL_SURFACE ( 'NONE', #57854, 88.90000000000000568 ) ;
#33873=DIRECTION ( 'NONE',  ( 0.000000000000000000, 0.000000000000000000, 1.000000000000000000 ) ) ;
#33895=DIRECTION ( 'NONE',  ( -0.5000000000000008882, 0.000000000000000000, 0.8660254037844382635 ) ) ;
#33913=VECTOR ( 'NONE', #33098, 1000.000000000000000 ) ;
#33915=ORIENTED_EDGE ( 'NONE', *, *, #61620, .F. ) ;
#33916=EDGE_CURVE ( 'NONE', #25068, #45031, #41778, .T. ) ;
#33968=CARTESIAN_POINT ( 'NONE',  ( 2.884119045937113768, 70.17489121805367347, -118.5216098345816960 ) ) ;
#33978=CIRCLE ( 'NONE', #60098, 5.041900000000001825 ) ;
#34004=CARTESIAN_POINT ( 'NONE',  ( -130.0134714785365304, 87.03008507238369873, 11.89083589963811072 ) ) ;
#34016=CARTESIAN_POINT ( 'NONE',  ( 72.96458098368650269, 117.4749999999999943, 78.00648098368728256 ) ) ;
#34024=AXIS2_PLACEMENT_3D ( 'NONE', #11784, #4964, #39917 ) ;
#34038=VECTOR ( 'NONE', #59825, 1000.000000000000000 ) ;
#34040=CARTESIAN_POINT ( 'NONE',  ( -117.9189176348423160, 85.83559868056555331, 12.27472195321796278 ) ) ;
#34046=FACE_BOUND ( 'NONE', #57229, .T. ) ;
#34060=CARTESIAN_POINT ( 'NONE',  ( 91.91945768840240305, 86.64222086580514315, -74.87617104506203702 ) ) ;
#34069=EDGE_CURVE ( 'NONE', #76220, #2396, #67505, .T. ) ;
#34079=CARTESIAN_POINT ( 'NONE',  ( 130.5150051272323140, 94.82199753261677699, -3.295598630355848879 ) ) ;
#34091=CARTESIAN_POINT ( 'NONE',  ( -10.33379165269208499, 75.15577250977247559, -130.1465911299492006 ) ) ;
#34100=DIRECTION ( 'NONE',  ( 0.000000000000000000, 0.000000000000000000, 1.000000000000000000 ) ) ;
#34114=FILL_AREA_STYLE ('',( #40036 ) ) ;
#34115=AXIS2_PLACEMENT_3D ( 'NONE', #74080, #11862, #39105 ) ;
#34117=CARTESIAN_POINT ( 'NONE',  ( 83.52520760052966864, 78.07027470200927155, -100.3415888741734818 ) ) ;
#34136=VERTEX_POINT ( 'NONE', #87129 ) ;
#34138=PLANE ( 'NONE',  #42806 ) ;
#34139=ORIENTED_EDGE ( 'NONE', *, *, #68472, .F. ) ;
#34145=CARTESIAN_POINT ( 'NONE',  ( 105.4788588808464027, 120.6499999999999915, 3.968750000000405009 ) ) ;
#34146=CARTESIAN_POINT ( 'NONE',  ( -100.8594679592212344, 82.54999999999999716, 82.89895571708261457 ) ) ;
#34157=DIRECTION ( 'NONE',  ( 0.5000000000000008882, 0.000000000000000000, -0.8660254037844382635 ) ) ;
#34165=CARTESIAN_POINT ( 'NONE',  ( -86.68128281353534703, 72.47310549519059464, -97.62852612868761071 ) ) ;
#34171=ORIENTED_EDGE ( 'NONE', *, *, #2514, .T. ) ;
#34178=ORIENTED_EDGE ( 'NONE', *, *, #40683, .T. ) ;
#34179=CIRCLE ( 'NONE', #7863, 34.13125000000000142 ) ;
#34197=CARTESIAN_POINT ( 'NONE',  ( 12.70000000000000107, 82.54999999999999716, 117.8738102209307641 ) ) ;
#34199=ORIENTED_EDGE ( 'NONE', *, *, #23098, .T. ) ;
#34221=CARTESIAN_POINT ( 'NONE',  ( -31.75000000000000000, 124.5870000000000033, 3.174999999999779998 ) ) ;
#34227=CARTESIAN_POINT ( 'NONE',  ( 12.67976775996874395, 83.37995484863286322, -117.8759955821573016 ) ) ;
#34241=DIRECTION ( 'NONE',  ( 0.000000000000000000, -1.000000000000000000, 0.000000000000000000 ) ) ;
#34245=VECTOR ( 'NONE', #2905, 1000.000000000000000 ) ;
#34250=LINE ( 'NONE', #25761, #65047 ) ;
#34259=CARTESIAN_POINT ( 'NONE',  ( -92.27899210470870628, 80.89685143461889538, 74.43211355457145828 ) ) ;
#34277=ORIENTED_EDGE ( 'NONE', *, *, #50166, .T. ) ;
#34288=VERTEX_POINT ( 'NONE', #28019 ) ;
#34294=ORIENTED_EDGE ( 'NONE', *, *, #16766, .T. ) ;
#34297=EDGE_CURVE ( 'NONE', #34136, #32236, #40018, .T. ) ;
#34307=FACE_OUTER_BOUND ( 'NONE', #40673, .T. ) ;
#34310=ADVANCED_FACE ( 'NONE', ( #68017 ), #55697, .F. ) ;
#34318=ORIENTED_EDGE ( 'NONE', *, *, #44395, .T. ) ;
#34319=CARTESIAN_POINT ( 'NONE',  ( 130.2059614519578190, 74.16222525595217974, 9.571858562770211520 ) ) ;
#34376=LINE ( 'NONE', #5341, #80496 ) ;
#34406=CARTESIAN_POINT ( 'NONE',  ( 72.96458098368701428, 117.4749999999999943, -80.90208098368670164 ) ) ;
#34434=DIRECTION ( 'NONE',  ( 0.000000000000000000, 0.000000000000000000, 1.000000000000000000 ) ) ;
#34435=CONICAL_SURFACE ( 'NONE', #85254, 24.63800000000000168, 0.7853981633974710386 ) ;
#34457=AXIS2_PLACEMENT_3D ( 'NONE', #85305, #23080, #78487 ) ;
#34465=ORIENTED_EDGE ( 'NONE', *, *, #38830, .T. ) ;
#34470=DIRECTION ( 'NONE',  ( -1.000000000000000000, 0.000000000000000000, -3.491481338843133355E-15 ) ) ;
#34473=CARTESIAN_POINT ( 'NONE',  ( 92.27764637677411486, 80.88465057165900873, 74.43377912862234780 ) ) ;
#34482=PLANE ( 'NONE',  #60259 ) ;
#34488=CIRCLE ( 'NONE', #21476, 9.525000000000000355 ) ;
#34496=CARTESIAN_POINT ( 'NONE',  ( -118.4860461769941935, 94.58006533271584715, 4.091503224720273835 ) ) ;
#34499=CARTESIAN_POINT ( 'NONE',  ( 77.68655577178724059, 72.98405218941671535, -89.55818655986089993 ) ) ;
#34519=CARTESIAN_POINT ( 'NONE',  ( 90.66710916952493449, 90.29828471680515634, -76.38857008572948359 ) ) ;
#34543=ORIENTED_EDGE ( 'NONE', *, *, #24127, .F. ) ;
#34554=ORIENTED_EDGE ( 'NONE', *, *, #73261, .T. ) ;
#34555=CARTESIAN_POINT ( 'NONE',  ( -87.71317827224427788, 71.15456258041353976, -79.76251016565912266 ) ) ;
#34560=DIRECTION ( 'NONE',  ( -0.8660254037844379305, 0.000000000000000000, 0.5000000000000011102 ) ) ;
#34570=CARTESIAN_POINT ( 'NONE',  ( 88.25674559704616229, 71.15434825076370373, -96.20681132576072514 ) ) ;
#34575=CIRCLE ( 'NONE', #7026, 7.937500000000000000 ) ;
#34598=CARTESIAN_POINT ( 'NONE',  ( 105.4788588808462038, 120.6499999999999915, -3.968749999999580336 ) ) ;
#34599=ADVANCED_FACE ( 'NONE', ( #6038 ), #61417, .F. ) ;
#34601=DIRECTION ( 'NONE',  ( 0.8660254037844387076, 0.000000000000000000, 0.4999999999999998890 ) ) ;
#34602=DIRECTION ( 'NONE',  ( -0.2588190451025194072, 0.000000000000000000, -0.9659258262890686453 ) ) ;
#34611=CARTESIAN_POINT ( 'NONE',  ( 72.96458098368650269, 101.5999999999999943, 72.96458098368729850 ) ) ;
#34612=EDGE_CURVE ( 'NONE', #51571, #72171, #32758, .T. ) ;
#34624=CARTESIAN_POINT ( 'NONE',  ( -89.55756476669488109, 92.11680164986012187, -77.68727430815000901 ) ) ;
#34650=CARTESIAN_POINT ( 'NONE',  ( 6.350224805574143261, 93.55624312175208956, 118.3863781049609543 ) ) ;
#34652=ORIENTED_EDGE ( 'NONE', *, *, #57519, .T. ) ;
#34660=CARTESIAN_POINT ( 'NONE',  ( 0.000000000000000000, 82.54999999999999716, 97.46299999999996544 ) ) ;
#34673=CARTESIAN_POINT ( 'NONE',  ( -103.1875000000000000, 117.4749999999999943, -7.143750000001079847 ) ) ;
#34686=LINE ( 'NONE', #61052, #70809 ) ;
#34711=CARTESIAN_POINT ( 'NONE',  ( -83.24493215373352939, 69.84937538953987257, 84.41866557162701667 ) ) ;
#34718=EDGE_CURVE ( 'NONE', #63421, #41468, #41856, .T. ) ;
#34730=ORIENTED_EDGE ( 'NONE', *, *, #17250, .T. ) ;
#34735=CARTESIAN_POINT ( 'NONE',  ( -86.68005309089119237, 92.64985122628466740, -97.63151088911729403 ) ) ;
#34774=CARTESIAN_POINT ( 'NONE',  ( -129.9368274816651478, 82.54999999999999716, 12.69999999999954809 ) ) ;
#34777=AXIS2_PLACEMENT_3D ( 'NONE', #63366, #62013, #54729 ) ;
#34811=EDGE_CURVE ( 'NONE', #13215, #82109, #75959, .T. ) ;
#34829=DIRECTION ( 'NONE',  ( 0.000000000000000000, 1.000000000000000000, 0.000000000000000000 ) ) ;
#34833=CARTESIAN_POINT ( 'NONE',  ( 94.61838531165655297, 94.82199753261677699, 89.95770503246943406 ) ) ;
#34836=CARTESIAN_POINT ( 'NONE',  ( 76.20505178924389611, 120.6499999999999915, -76.20505178924359768 ) ) ;
#34842=EDGE_CURVE ( 'NONE', #62184, #72426, #82198, .T. ) ;
#34848=DIRECTION ( 'NONE',  ( 0.000000000000000000, 0.000000000000000000, 1.000000000000000000 ) ) ;
#34858=CARTESIAN_POINT ( 'NONE',  ( -11.00058663074870680, 88.91008943578141555, 118.0447001808843766 ) ) ;
#34874=LINE ( 'NONE', #49836, #328 ) ;
#34875=AXIS2_PLACEMENT_3D ( 'NONE', #80071, #31442, #11002 ) ;
#34876=EDGE_CURVE ( 'NONE', #16565, #52873, #76854, .T. ) ;
#34884=DIRECTION ( 'NONE',  ( 0.000000000000000000, 1.000000000000000000, 0.000000000000000000 ) ) ;
#34904=CARTESIAN_POINT ( 'NONE',  ( 96.94335780202260366, 71.76234181793742550, 87.44698480207861735 ) ) ;
#34910=ADVANCED_FACE ( 'NONE', ( #9162 ), #52236, .F. ) ;
#34934=DIRECTION ( 'NONE',  ( -1.000000000000000000, 0.000000000000000000, -3.491481338843133355E-15 ) ) ;
#34941=CARTESIAN_POINT ( 'NONE',  ( -3.174999999999664979, 104.3431970271541616, -31.75000000000000000 ) ) ;
#34947=CARTESIAN_POINT ( 'NONE',  ( 75.00102098090802372, 78.06989712577870932, -91.81719692706813873 ) ) ;
#34973=CIRCLE ( 'NONE', #30642, 5.041900000000001825 ) ;
#34981=DIRECTION ( 'NONE',  ( 0.000000000000000000, 1.000000000000000000, 0.000000000000000000 ) ) ;
#35013=CARTESIAN_POINT ( 'NONE',  ( 84.91200770515678187, 74.81660785136578795, -99.17101862044572158 ) ) ;
#35019=EDGE_CURVE ( 'NONE', #9633, #51660, #48756, .T. ) ;
#35043=CARTESIAN_POINT ( 'NONE',  ( -94.61736061587603785, 70.27756284692561906, 89.95878776288257939 ) ) ;
#35050=FACE_OUTER_BOUND ( 'NONE', #19279, .T. ) ;
#35062=CARTESIAN_POINT ( 'NONE',  ( -83.24642779537455795, 95.23005795263746620, -84.41404664249405698 ) ) ;
#35076=FACE_BOUND ( 'NONE', #4281, .T. ) ;
#35114=LINE ( 'NONE', #55536, #69454 ) ;
#35118=CARTESIAN_POINT ( 'NONE',  ( 10.78716141056406741, 89.26551436951581309, -118.0644550036098508 ) ) ;
#35119=CARTESIAN_POINT ( 'NONE',  ( -8.387211759491222551, 92.12327290876403652, 130.2876699444761073 ) ) ;
#35124=ORIENTED_EDGE ( 'NONE', *, *, #2514, .F. ) ;
#35133=CARTESIAN_POINT ( 'NONE',  ( 129.9368274816649489, 82.96445444011519044, 12.70000000000135998 ) ) ;
#35138=AXIS2_PLACEMENT_3D ( 'NONE', #85761, #51195, #17149 ) ;
#35159=CARTESIAN_POINT ( 'NONE',  ( -7.205548786489490269E-13, 127.0000000000000000, 103.1875000000000000 ) ) ;
#35169=CARTESIAN_POINT ( 'NONE',  ( 11.41387019979801387, 76.91918732108555901, 130.0565070412864372 ) ) ;
#35170=CARTESIAN_POINT ( 'NONE',  ( -100.8069756963041499, 84.21449860606321636, -82.96293804092829305 ) ) ;
#35211=CARTESIAN_POINT ( 'NONE',  ( 130.2867309503043884, 73.00415124681448731, 8.386992461123922382 ) ) ;
#35223=ADVANCED_FACE ( 'NONE', ( #13617 ), #28581, .F. ) ;
#35238=EDGE_LOOP ( 'NONE', ( #785, #51298, #30589, #81772 ) ) ;
#35254=EDGE_CURVE ( 'NONE', #9436, #75690, #5913, .T. ) ;
#35273=CARTESIAN_POINT ( 'NONE',  ( 83.90854149456365008, 88.17609398443094904, 100.0213216842708732 ) ) ;
#35298=VERTEX_POINT ( 'NONE', #30827 ) ;
#35299=CARTESIAN_POINT ( 'NONE',  ( -118.0639734269500565, 75.84278307195158675, -10.79247489890467193 ) ) ;
#35333=LINE ( 'NONE', #8093, #24855 ) ;
#35334=DIRECTION ( 'NONE',  ( 0.000000000000000000, 1.000000000000000000, 0.000000000000000000 ) ) ;
#35358=ORIENTED_EDGE ( 'NONE', *, *, #19109, .T. ) ;
#35370=ORIENTED_EDGE ( 'NONE', *, *, #66045, .T. ) ;
#35374=DIRECTION ( 'NONE',  ( -0.8660254037844387076, 0.000000000000000000, 0.4999999999999998890 ) ) ;
#35376=CARTESIAN_POINT ( 'NONE',  ( -97.46299999999996544, 82.54999999999999716, -3.402902457276681768E-13 ) ) ;
#35382=CARTESIAN_POINT ( 'NONE',  ( -92.07164801315005320, 85.85031469618033384, 74.68844285250203541 ) ) ;
#35390=DIRECTION ( 'NONE',  ( -1.000000000000000000, 0.000000000000000000, 0.000000000000000000 ) ) ;
#35401=LINE ( 'NONE', #901, #58852 ) ;
#35409=AXIS2_PLACEMENT_3D ( 'NONE', #48443, #13963, #27588 ) ;
#35415=DIRECTION ( 'NONE',  ( 0.000000000000000000, 1.000000000000000000, 0.000000000000000000 ) ) ;
#35425=CARTESIAN_POINT ( 'NONE',  ( 68.53801554307449351, 120.6499999999999915, -74.15067561874229796 ) ) ;
#35427=PLANE ( 'NONE',  #42147 ) ;
#35447=CARTESIAN_POINT ( 'NONE',  ( -80.88853703239314541, 70.52018178143197247, -86.67600044576322205 ) ) ;
#35450=VERTEX_POINT ( 'NONE', #32599 ) ;
#35468=DIRECTION ( 'NONE',  ( 0.000000000000000000, 0.000000000000000000, 1.000000000000000000 ) ) ;
#35476=VECTOR ( 'NONE', #54641, 1000.000000000000000 ) ;
#35477=LINE ( 'NONE', #85009, #8515 ) ;
#35481=VECTOR ( 'NONE', #75016, 1000.000000000000000 ) ;
#35487=CYLINDRICAL_SURFACE ( 'NONE', #42734, 7.143750000000004263 ) ;
#35489=PLANE ( 'NONE',  #9484 ) ;
#35500=CARTESIAN_POINT ( 'NONE',  ( 3.174999999999879918, 111.1250000000000000, 33.98325472291465132 ) ) ;
#35533=ORIENTED_EDGE ( 'NONE', *, *, #61915, .T. ) ;
#35538=ORIENTED_EDGE ( 'NONE', *, *, #22128, .T. ) ;
#35540=LINE ( 'NONE', #22836, #51212 ) ;
#35548=B_SPLINE_CURVE_WITH_KNOTS ( 'NONE', 3,
 ( #71882, #44590, #65058, #2841, #36903, #10097, #63718, #23737, #84627, #8766, #57789, #58239, #79598, #85967, #37802, #65502, #29640, #3286, #30977, #51845, #17357, #45038, #72768, #10537, #1499 ),
 .UNSPECIFIED., .F., .F.,
 ( 4, 2, 2, 2, 2, 2, 2, 2, 2, 1, 2, 2, 4 ),
 ( 2.608264963112508895E-18, 0.002483666291998854608, 0.003725499437998279744, 0.004967332583997703145, 0.007450998875996568162, 0.008692832021995991129, 0.009934665167995411494, 0.01241833145999425222, 0.01366016460599367086, 0.01490199775199309122, 0.01614383089799251159, 0.01738566404399193022, 0.01986933033599076748 ),
 .UNSPECIFIED. ) ;
#35582=DIRECTION ( 'NONE',  ( 0.000000000000000000, 0.000000000000000000, 1.000000000000000000 ) ) ;
#35601=CARTESIAN_POINT ( 'NONE',  ( -79.76251016565881002, 71.15456258041352555, 87.71317827224459052 ) ) ;
#35607=VECTOR ( 'NONE', #59503, 999.9999999999998863 ) ;
#35610=VECTOR ( 'NONE', #28331, 1000.000000000000000 ) ;
#35625=VECTOR ( 'NONE', #14343, 1000.000000000000000 ) ;
#35634=AXIS2_PLACEMENT_3D ( 'NONE', #46294, #59484, #66303 ) ;
#35636=ORIENTED_EDGE ( 'NONE', *, *, #25443, .T. ) ;
#35653=ORIENTED_EDGE ( 'NONE', *, *, #27531, .T. ) ;
#35660=ADVANCED_FACE ( 'NONE', ( #28028 ), #72516, .F. ) ;
#35664=FACE_OUTER_BOUND ( 'NONE', #23124, .T. ) ;
#35665=ORIENTED_EDGE ( 'NONE', *, *, #5103, .T. ) ;
#35666=CARTESIAN_POINT ( 'NONE',  ( 130.4793906290846337, 70.66229531820916065, 4.488385961154077286 ) ) ;
#35668=VERTEX_POINT ( 'NONE', #23037 ) ;
#35686=DIRECTION ( 'NONE',  ( 0.000000000000000000, 1.000000000000000000, 0.000000000000000000 ) ) ;
#35698=LINE ( 'NONE', #50216, #60874 ) ;
#35704=AXIS2_PLACEMENT_3D ( 'NONE', #21658, #2098, #84784 ) ;
#35707=ORIENTED_EDGE ( 'NONE', *, *, #64702, .F. ) ;
#35723=CARTESIAN_POINT ( 'NONE',  ( 0.000000000000000000, 92.07499999999998863, 9.525000000000000355 ) ) ;
#35724=CARTESIAN_POINT ( 'NONE',  ( 96.20559720633507084, 93.94653598907720493, 88.25806911646444064 ) ) ;
#35742=ORIENTED_EDGE ( 'NONE', *, *, #55213, .T. ) ;
#35774=DIRECTION ( 'NONE',  ( -0.7071067811865487940, 0.000000000000000000, 0.7071067811865463515 ) ) ;
#35787=CARTESIAN_POINT ( 'NONE',  ( 0.000000000000000000, 92.07499999999998863, 0.000000000000000000 ) ) ;
#35797=CARTESIAN_POINT ( 'NONE',  ( 91.71670967179916545, 69.85063703626885001, 92.91726854070194008 ) ) ;
#35831=VERTEX_POINT ( 'NONE', #78451 ) ;
#35836=CARTESIAN_POINT ( 'NONE',  ( -80.31773373136844896, 94.30044247306078375, 87.20679752240629057 ) ) ;
#35886=ADVANCED_FACE ( 'NONE', ( #40201 ), #34435, .T. ) ;
#35887=AXIS2_PLACEMENT_3D ( 'NONE', #82167, #6287, #13997 ) ;
#35888=CARTESIAN_POINT ( 'NONE',  ( -103.1875000000000000, 117.4749999999999943, -1.080832317973422076E-12 ) ) ;
#35891=AXIS2_PLACEMENT_3D ( 'NONE', #53692, #13293, #11952 ) ;
#35916=CARTESIAN_POINT ( 'NONE',  ( 92.91726854070162744, 69.85063703626886422, -91.71670967179946388 ) ) ;
#35917=LINE ( 'NONE', #1417, #42289 ) ;
#35942=LINE ( 'NONE', #30033, #73031 ) ;
#35957=CYLINDRICAL_SURFACE ( 'NONE', #82130, 7.937500000000000000 ) ;
#35960=EDGE_CURVE ( 'NONE', #64446, #59215, #39316, .T. ) ;
#35971=CARTESIAN_POINT ( 'NONE',  ( -87.20679752240603477, 94.30044247306076954, -80.31773373136881844 ) ) ;
#35994=ORIENTED_EDGE ( 'NONE', *, *, #34612, .F. ) ;
#35997=CARTESIAN_POINT ( 'NONE',  ( 0.000000000000000000, 103.1240000000000236, 190.5000000000000000 ) ) ;
#35998=ORIENTED_EDGE ( 'NONE', *, *, #51307, .F. ) ;
#36000=DIRECTION ( 'NONE',  ( -0.8660254037844381525, 0.000000000000000000, -0.5000000000000007772 ) ) ;
#36011=AXIS2_PLACEMENT_3D ( 'NONE', #55371, #63104, #62207 ) ;
#36013=LINE ( 'NONE', #49172, #28941 ) ;
#36030=CARTESIAN_POINT ( 'NONE',  ( -4.090559613967782226, 94.60197653454001454, 130.4941709638410146 ) ) ;
#36032=DIRECTION ( 'NONE',  ( 0.000000000000000000, 1.000000000000000000, 0.000000000000000000 ) ) ;
#36040=AXIS2_PLACEMENT_3D ( 'NONE', #76754, #42653, #14077 ) ;
#36084=CARTESIAN_POINT ( 'NONE',  ( 2.899933897858971488, 70.17843983949715891, 130.5244343740981776 ) ) ;
#36094=ORIENTED_EDGE ( 'NONE', *, *, #42100, .T. ) ;
#36106=VECTOR ( 'NONE', #40302, 1000.000000000000000 ) ;
#36111=ORIENTED_EDGE ( 'NONE', *, *, #8810, .F. ) ;
#36120=CARTESIAN_POINT ( 'NONE',  ( 74.15067561874209900, 127.0000000000000000, 68.53801554307469246 ) ) ;
#36123=CARTESIAN_POINT ( 'NONE',  ( 4.665904304751420031E-15, 92.07499999999998863, -38.10000000000000142 ) ) ;
#36126=ORIENTED_EDGE ( 'NONE', *, *, #16573, .F. ) ;
#36140=CARTESIAN_POINT ( 'NONE',  ( 103.1875000000000000, 127.0000000000000000, 3.602774393244745134E-13 ) ) ;
#36146=LINE ( 'NONE', #42048, #27382 ) ;
#36160=ORIENTED_EDGE ( 'NONE', *, *, #8465, .F. ) ;
#36167=ORIENTED_EDGE ( 'NONE', *, *, #40677, .F. ) ;
#36188=DIRECTION ( 'NONE',  ( 0.000000000000000000, -1.000000000000000000, 0.000000000000000000 ) ) ;
#36194=FACE_OUTER_BOUND ( 'NONE', #80357, .T. ) ;
#36208=DIRECTION ( 'NONE',  ( 0.000000000000000000, -1.000000000000000000, 0.000000000000000000 ) ) ;
#36235=LINE ( 'NONE', #63946, #73620 ) ;
#36261=CARTESIAN_POINT ( 'NONE',  ( 95.69968022530667895, 70.80031561532538831, 88.80809839403396211 ) ) ;
#36275=CARTESIAN_POINT ( 'NONE',  ( 74.36911441044796334, 82.54999999999999716, -92.32962665258483526 ) ) ;
#36280=FACE_OUTER_BOUND ( 'NONE', #3027, .T. ) ;
#36296=DIRECTION ( 'NONE',  ( 0.000000000000000000, 0.000000000000000000, 1.000000000000000000 ) ) ;
#36302=CARTESIAN_POINT ( 'NONE',  ( -87.45628510944614220, 94.12556101775332706, 80.04418453221629193 ) ) ;
#36310=LINE ( 'NONE', #43549, #9240 ) ;
#36323=CARTESIAN_POINT ( 'NONE',  ( 78.17042387453767560, 92.64232203292142742, -89.13693605261687480 ) ) ;
#36369=ADVANCED_FACE ( 'NONE', ( #3804 ), #25580, .F. ) ;
#36399=ORIENTED_EDGE ( 'NONE', *, *, #27843, .F. ) ;
#36404=ORIENTED_EDGE ( 'NONE', *, *, #83252, .T. ) ;
#36420=DIRECTION ( 'NONE',  ( 0.000000000000000000, 1.000000000000000000, 0.000000000000000000 ) ) ;
#36422=CARTESIAN_POINT ( 'NONE',  ( -96.20686424029877060, 93.94566094357732311, 88.25669247804634665 ) ) ;
#36433=CARTESIAN_POINT ( 'NONE',  ( -82.89895571708224509, 81.72130195885952730, -100.8594679592214902 ) ) ;
#36434=CARTESIAN_POINT ( 'NONE',  ( -76.79137032886092129, 90.93965867633431799, -90.32698471909156979 ) ) ;
#36436=DIRECTION ( 'NONE',  ( 0.000000000000000000, 0.000000000000000000, 1.000000000000000000 ) ) ;
#36468=AXIS2_PLACEMENT_3D ( 'NONE', #85210, #28882, #22976 ) ;
#36469=VERTEX_POINT ( 'NONE', #1813 ) ;
#36490=CARTESIAN_POINT ( 'NONE',  ( -12.59759614370980252, 84.21308071816545748, 129.9468022370901394 ) ) ;
#36493=EDGE_CURVE ( 'NONE', #12394, #1981, #56753, .T. ) ;
#36536=LINE ( 'NONE', #45103, #83609 ) ;
#36538=ORIENTED_EDGE ( 'NONE', *, *, #52222, .F. ) ;
#36561=DIRECTION ( 'NONE',  ( 0.000000000000000000, 1.000000000000000000, 0.000000000000000000 ) ) ;
#36578=PLANE ( 'NONE',  #77685 ) ;
#36583=EDGE_LOOP ( 'NONE', ( #57907, #66550, #87485, #85593 ) ) ;
#36584=CARTESIAN_POINT ( 'NONE',  ( -129.9368274816650626, 81.72130195885952730, -12.70000000000045404 ) ) ;
#36588=AXIS2_PLACEMENT_3D ( 'NONE', #44402, #72138, #9913 ) ;
#36620=DIRECTION ( 'NONE',  ( 0.000000000000000000, 0.000000000000000000, 1.000000000000000000 ) ) ;
#36627=VERTEX_POINT ( 'NONE', #3582 ) ;
#36636=ORIENTED_EDGE ( 'NONE', *, *, #19955, .T. ) ;
#36637=ORIENTED_EDGE ( 'NONE', *, *, #78627, .T. ) ;
#36643=CARTESIAN_POINT ( 'NONE',  ( 83.02643542997934389, 84.62817240485476589, 100.7545871043113408 ) ) ;
#36692=DIRECTION ( 'NONE',  ( -0.000000000000000000, 1.000000000000000000, 0.000000000000000000 ) ) ;
#36696=CYLINDRICAL_SURFACE ( 'NONE', #8685, 38.10000000000000142 ) ;
#36724=VECTOR ( 'NONE', #60789, 1000.000000000000000 ) ;
#36743=DIRECTION ( 'NONE',  ( -0.000000000000000000, 1.000000000000000000, 0.000000000000000000 ) ) ;
#36751=CARTESIAN_POINT ( 'NONE',  ( -81.46927207886238875, 94.82191660594814664, 86.13037352894157550 ) ) ;
#36754=CYLINDRICAL_SURFACE ( 'NONE', #44977, 7.143749999999999822 ) ;
#36762=VERTEX_POINT ( 'NONE', #9964 ) ;
#36765=LINE ( 'NONE', #72627, #54707 ) ;
#36767=DIRECTION ( 'NONE',  ( 0.000000000000000000, -1.000000000000000000, 0.000000000000000000 ) ) ;
#36775=VERTEX_POINT ( 'NONE', #13092 ) ;
#36794=ORIENTED_EDGE ( 'NONE', *, *, #3907, .F. ) ;
#36800=DIRECTION ( 'NONE',  ( -0.5000000000000061062, 0.000000000000000000, 0.8660254037844351549 ) ) ;
#36830=DIRECTION ( 'NONE',  ( 0.000000000000000000, 1.000000000000000000, 0.000000000000000000 ) ) ;
#36836=AXIS2_PLACEMENT_3D ( 'NONE', #6407, #55872, #34100 ) ;
#36856=CARTESIAN_POINT ( 'NONE',  ( -92.60677566276767436, 95.25015599858943460, 92.02731164704691480 ) ) ;
#36888=CARTESIAN_POINT ( 'NONE',  ( 31.75000000000000000, 111.1250000000000000, 3.174999999999999822 ) ) ;
#36903=CARTESIAN_POINT ( 'NONE',  ( -3.286472755014015146, 70.27551020174914242, 130.5152393712291428 ) ) ;
#36926=CIRCLE ( 'NONE', #29734, 5.041900000000001825 ) ;
#36956=CARTESIAN_POINT ( 'NONE',  ( -100.8961411191535973, 120.6499999999999915, 3.968749999998880451 ) ) ;
#36962=CARTESIAN_POINT ( 'NONE',  ( -7.196800215918080040E-13, 127.0000000000000000, 110.3312500000000114 ) ) ;
#36964=LINE ( 'NONE', #2456, #86666 ) ;
#36966=CARTESIAN_POINT ( 'NONE',  ( -3.175000000000109956, 111.1250000000000000, 31.75000000000000000 ) ) ;
#36988=ORIENTED_EDGE ( 'NONE', *, *, #26232, .T. ) ;
#36991=VECTOR ( 'NONE', #70028, 1000.000000000000000 ) ;
#37005=ORIENTED_EDGE ( 'NONE', *, *, #33602, .T. ) ;
#37007=LINE ( 'NONE', #49725, #38609 ) ;
#37018=CARTESIAN_POINT ( 'NONE',  ( -129.9681501387584035, 79.66749569656610674, -12.37561169055459231 ) ) ;
#37056=AXIS2_PLACEMENT_3D ( 'NONE', #18734, #33710, #75942 ) ;
#37061=VECTOR ( 'NONE', #33012, 1000.000000000000000 ) ;
#37063=CARTESIAN_POINT ( 'NONE',  ( -10.08079905861141690, 90.28579524239222565, -130.1664991954058905 ) ) ;
#37083=ADVANCED_FACE ( 'NONE', ( #33414 ), #3920, .F. ) ;
#37086=DIRECTION ( 'NONE',  ( -0.7071067811865460184, 0.000000000000000000, -0.7071067811865489050 ) ) ;
#37088=CARTESIAN_POINT ( 'NONE',  ( 75.85717701425106441, 89.26692529358290074, 91.11128979799275385 ) ) ;
#37115=ORIENTED_EDGE ( 'NONE', *, *, #4887, .F. ) ;
#37124=LINE ( 'NONE', #43014, #77896 ) ;
#37140=DIRECTION ( 'NONE',  ( 0.000000000000000000, 1.000000000000000000, 0.000000000000000000 ) ) ;
#37155=CARTESIAN_POINT ( 'NONE',  ( 72.96458098368701428, 117.4749999999999943, -78.00648098368678518 ) ) ;
#37171=CARTESIAN_POINT ( 'NONE',  ( 83.23139715273200068, 69.85063172184842983, 84.43201024598489823 ) ) ;
#37200=DIRECTION ( 'NONE',  ( 0.000000000000000000, -1.000000000000000000, 0.000000000000000000 ) ) ;
#37202=CARTESIAN_POINT ( 'NONE',  ( 91.90683392111127148, 78.46407912418312947, -74.89107914305729707 ) ) ;
#37208=VERTEX_POINT ( 'NONE', #30189 ) ;
#37218=VERTEX_POINT ( 'NONE', #78802 ) ;
#37220=CARTESIAN_POINT ( 'NONE',  ( -7.205548786489490269E-13, 127.0000000000000000, 111.1250000000000000 ) ) ;
#37237=VERTEX_POINT ( 'NONE', #16559 ) ;
#37256=ORIENTED_EDGE ( 'NONE', *, *, #44027, .F. ) ;
#37259=ORIENTED_EDGE ( 'NONE', *, *, #60049, .F. ) ;
#37305=CARTESIAN_POINT ( 'NONE',  ( -88.80956239834375765, 94.30053025434482095, 95.69832483115281718 ) ) ;
#37310=CARTESIAN_POINT ( 'NONE',  ( 0.000000000000000000, 198.8420489685532004, -25.39999999999999858 ) ) ;
#37325=EDGE_LOOP ( 'NONE', ( #27111, #39670, #64374, #49338 ) ) ;
#37359=LINE ( 'NONE', #23746, #68330 ) ;
#37414=CARTESIAN_POINT ( 'NONE',  ( 118.5472164932298256, 69.93120980984943458, -1.660430599528443851 ) ) ;
#37438=CIRCLE ( 'NONE', #88222, 130.5560000000000116 ) ;
#37445=VERTEX_POINT ( 'NONE', #87236 ) ;
#37483=EDGE_CURVE ( 'NONE', #69399, #64426, #15584, .T. ) ;
#37496=DIRECTION ( 'NONE',  ( 8.659560562355169516E-17, -0.7071067811865280328, 0.7071067811865670016 ) ) ;
#37508=EDGE_CURVE ( 'NONE', #75109, #83315, #39066, .T. ) ;
#37512=AXIS2_PLACEMENT_3D ( 'NONE', #16769, #36767, #29956 ) ;
#37513=CARTESIAN_POINT ( 'NONE',  ( -9.270409258063830649, 91.24028187095998987, -130.2267823906806257 ) ) ;
#37535=CARTESIAN_POINT ( 'NONE',  ( 74.36911441044604487, 82.54999999999999716, 92.32962665258637003 ) ) ;
#37539=CARTESIAN_POINT ( 'NONE',  ( 4.867771054587877622, 94.30191638479369942, 130.4669033451685891 ) ) ;
#37547=ORIENTED_EDGE ( 'NONE', *, *, #82457, .T. ) ;
#37556=CARTESIAN_POINT ( 'NONE',  ( -7.205548786489490269E-13, 117.4749999999999943, 108.2293999999999983 ) ) ;
#37562=ORIENTED_EDGE ( 'NONE', *, *, #22033, .T. ) ;
#37568=CARTESIAN_POINT ( 'NONE',  ( 0.000000000000000000, 61.59999999999999432, 0.000000000000000000 ) ) ;
#37596=LINE ( 'NONE', #78939, #30927 ) ;
#37597=EDGE_CURVE ( 'NONE', #27593, #27929, #51789, .T. ) ;
#37608=DIRECTION ( 'NONE',  ( 0.000000000000000000, 1.000000000000000000, 0.000000000000000000 ) ) ;
#37625=CARTESIAN_POINT ( 'NONE',  ( 91.26337341211373655, 76.18740257834571139, 75.67519899969754249 ) ) ;
#37628=EDGE_LOOP ( 'NONE', ( #30285, #10713, #79953, #48119 ) ) ;
#37644=CARTESIAN_POINT ( 'NONE',  ( -3.175000000000109956, 104.3431970271541900, 31.75000000000000000 ) ) ;
#37647=DIRECTION ( 'NONE',  ( 0.000000000000000000, 0.000000000000000000, 1.000000000000000000 ) ) ;
#37667=ORIENTED_EDGE ( 'NONE', *, *, #4534, .T. ) ;
#37683=DIRECTION ( 'NONE',  ( 0.000000000000000000, -1.000000000000000000, 0.000000000000000000 ) ) ;
#37694=CYLINDRICAL_SURFACE ( 'NONE', #32728, 7.143750000000004263 ) ;
#37721=EDGE_LOOP ( 'NONE', ( #23153, #201, #54039, #62292 ) ) ;
#37737=VERTEX_POINT ( 'NONE', #44881 ) ;
#37771=DIRECTION ( 'NONE',  ( 0.000000000000000000, 0.000000000000000000, 1.000000000000000000 ) ) ;
#37792=DIRECTION ( 'NONE',  ( 8.659560562354778784E-17, 0.7071067811865600072, -0.7071067811865350272 ) ) ;
#37802=CARTESIAN_POINT ( 'NONE',  ( -10.09455232642977052, 74.79837219561763106, 130.1659940687516723 ) ) ;
#37807=EDGE_CURVE ( 'NONE', #64886, #2396, #40342, .T. ) ;
#37814=ORIENTED_EDGE ( 'NONE', *, *, #27308, .F. ) ;
#37848=LINE ( 'NONE', #78310, #79176 ) ;
#37862=CARTESIAN_POINT ( 'NONE',  ( -6.706703101270981046E-13, 127.0000000000000000, 96.04375000000000284 ) ) ;
#37866=CARTESIAN_POINT ( 'NONE',  ( 118.4576332894986734, 70.80054595721395572, -4.873637472994857056 ) ) ;
#37868=CARTESIAN_POINT ( 'NONE',  ( -69.72411017812909506, 127.0000000000000000, -69.72411017813089984 ) ) ;
#37882=ORIENTED_EDGE ( 'NONE', *, *, #28768, .F. ) ;
#37883=ORIENTED_EDGE ( 'NONE', *, *, #1621, .F. ) ;
#37909=CARTESIAN_POINT ( 'NONE',  ( -130.5150461639146044, 70.27756284692560484, -3.294108455003483815 ) ) ;
#37930=DIRECTION ( 'NONE',  ( 0.000000000000000000, 0.000000000000000000, 1.000000000000000000 ) ) ;
#37948=CARTESIAN_POINT ( 'NONE',  ( -12.61760061281886003, 84.21489741558211506, -129.9449561063389638 ) ) ;
#37963=CARTESIAN_POINT ( 'NONE',  ( 0.000000000000000000, 127.0000000000000000, -98.14560000000000173 ) ) ;
#37965=EDGE_CURVE ( 'NONE', #89588, #32260, #22607, .T. ) ;
#37971=ORIENTED_EDGE ( 'NONE', *, *, #29692, .F. ) ;
#37979=EDGE_CURVE ( 'NONE', #28373, #6171, #37124, .T. ) ;
#37982=EDGE_LOOP ( 'NONE', ( #56693, #80663, #51882, #2846 ) ) ;
#37995=EDGE_CURVE ( 'NONE', #41588, #30196, #14897, .T. ) ;
#37998=ADVANCED_FACE ( 'NONE', ( #71649, #71205 ), #64825, .T. ) ;
#38015=FACE_BOUND ( 'NONE', #14691, .T. ) ;
#38027=CARTESIAN_POINT ( 'NONE',  ( 0.000000000000000000, 61.59999999999999432, 0.000000000000000000 ) ) ;
#38056=VERTEX_POINT ( 'NONE', #30748 ) ;
#38074=CARTESIAN_POINT ( 'NONE',  ( 118.1709372608869160, 90.93089219781630561, -9.551212252128932434 ) ) ;
#38075=DIRECTION ( 'NONE',  ( -0.7071067811865487940, 0.000000000000000000, 0.7071067811865463515 ) ) ;
#38077=ORIENTED_EDGE ( 'NONE', *, *, #3745, .F. ) ;
#38168=DIRECTION ( 'NONE',  ( 0.000000000000000000, 0.000000000000000000, 1.000000000000000000 ) ) ;
#38188=CARTESIAN_POINT ( 'NONE',  ( -100.4448767513717513, 86.64186789594789673, 83.40142812120620874 ) ) ;
#38206=CYLINDRICAL_SURFACE ( 'NONE', #79565, 7.143749999999999822 ) ;
#38207=DIRECTION ( 'NONE',  ( 0.000000000000000000, 0.000000000000000000, 1.000000000000000000 ) ) ;
#38228=ORIENTED_EDGE ( 'NONE', *, *, #1414, .F. ) ;
#38248=CARTESIAN_POINT ( 'NONE',  ( 76.20505178924339873, 120.6499999999999915, 76.20505178924419454 ) ) ;
#38285=CARTESIAN_POINT ( 'NONE',  ( -82.89895571708294142, 81.71102547120851511, 100.8594679592209644 ) ) ;
#38296=CARTESIAN_POINT ( 'NONE',  ( 118.3661894536416526, 71.76236341257998674, -6.714990428327953786 ) ) ;
#38332=ORIENTED_EDGE ( 'NONE', *, *, #85334, .F. ) ;
#38372=CARTESIAN_POINT ( 'NONE',  ( -72.96458098368600531, 127.0000000000000000, -72.96458098368781009 ) ) ;
#38404=CIRCLE ( 'NONE', #31147, 7.937500000000000000 ) ;
#38411=CARTESIAN_POINT ( 'NONE',  ( 12.37532827966387927, 85.43317223346194567, 129.9681767497193334 ) ) ;
#38440=FACE_BOUND ( 'NONE', #63821, .T. ) ;
#38442=PLANE ( 'NONE',  #48156 ) ;
#38468=LINE ( 'NONE', #26194, #41497 ) ;
#38473=CARTESIAN_POINT ( 'NONE',  ( -103.1875000000000000, 127.0000000000000000, -1.080832317973422076E-12 ) ) ;
#38476=LINE ( 'NONE', #66179, #1042 ) ;
#38484=VERTEX_POINT ( 'NONE', #80039 ) ;
#38485=ORIENTED_EDGE ( 'NONE', *, *, #65102, .T. ) ;
#38506=CARTESIAN_POINT ( 'NONE',  ( 117.9423201497064611, 86.64222086580515736, 12.05142355921225317 ) ) ;
#38544=ORIENTED_EDGE ( 'NONE', *, *, #8097, .F. ) ;
#38555=CARTESIAN_POINT ( 'NONE',  ( 71.77848634863079269, 127.0000000000000000, 77.39114642429989033 ) ) ;
#38602=CARTESIAN_POINT ( 'NONE',  ( -72.96458098368600531, 117.4749999999999943, -80.90208098368781009 ) ) ;
#38608=LINE ( 'NONE', #17731, #63980 ) ;
#38609=VECTOR ( 'NONE', #15224, 999.9999999999998863 ) ;
#38629=CARTESIAN_POINT ( 'NONE',  ( -118.5451175586562158, 95.14807216649715826, -1.659552426423821503 ) ) ;
#38638=ORIENTED_EDGE ( 'NONE', *, *, #21220, .F. ) ;
#38640=CARTESIAN_POINT ( 'NONE',  ( 107.7702177616926065, 120.6499999999999915, 4.179089330879380409E-13 ) ) ;
#38650=VECTOR ( 'NONE', #34560, 1000.000000000000114 ) ;
#38677=CARTESIAN_POINT ( 'NONE',  ( -89.55818655986118415, 72.98405218941672956, -77.68655577178692795 ) ) ;
#38680=ORIENTED_EDGE ( 'NONE', *, *, #74708, .T. ) ;
#38724=CARTESIAN_POINT ( 'NONE',  ( 69.72411017813010403, 120.6499999999999915, -69.72411017812979139 ) ) ;
#38728=CARTESIAN_POINT ( 'NONE',  ( -84.19388261207966195, 76.18750001922977333, 99.78212687779766554 ) ) ;
#38741=CARTESIAN_POINT ( 'NONE',  ( 118.2594037030538772, 73.00424585431355240, 8.387096233284163205 ) ) ;
#38753=AXIS2_PLACEMENT_3D ( 'NONE', #12581, #27988, #40268 ) ;
#38788=VECTOR ( 'NONE', #4949, 999.9999999999998863 ) ;
#38806=EDGE_CURVE ( 'NONE', #7755, #29308, #78156, .T. ) ;
#38813=CARTESIAN_POINT ( 'NONE',  ( -5.617021782840702748, 93.94788616487885236, -118.4234307144629241 ) ) ;
#38830=EDGE_CURVE ( 'NONE', #89346, #29480, #79522, .T. ) ;
#38832=CARTESIAN_POINT ( 'NONE',  ( -12.37532827966388282, 85.43317223346198830, -129.9681767497193903 ) ) ;
#38851=CARTESIAN_POINT ( 'NONE',  ( 74.68844285250109749, 85.85031469618033384, 92.07164801315086322 ) ) ;
#38859=AXIS2_PLACEMENT_3D ( 'NONE', #72168, #37200, #37647 ) ;
#38871=ORIENTED_EDGE ( 'NONE', *, *, #38830, .F. ) ;
#38880=ORIENTED_EDGE ( 'NONE', *, *, #56517, .T. ) ;
#38891=ORIENTED_EDGE ( 'NONE', *, *, #8731, .F. ) ;
#38915=EDGE_CURVE ( 'NONE', #27899, #45930, #80826, .T. ) ;
#38927=CARTESIAN_POINT ( 'NONE',  ( -72.96458098368751166, 117.4749999999999943, 67.92268098368620599 ) ) ;
#38928=CIRCLE ( 'NONE', #33094, 7.143750000000004263 ) ;
#38943=CARTESIAN_POINT ( 'NONE',  ( 3.175000000000334666, 111.1250000000000000, -31.75000000000000000 ) ) ;
#38955=CARTESIAN_POINT ( 'NONE',  ( 118.4232034889089249, 93.94553785444266225, 5.621872244392114304 ) ) ;
#38991=CARTESIAN_POINT ( 'NONE',  ( -118.4241986436612564, 71.14137858619480426, -5.641441481138969039 ) ) ;
#38996=ORIENTED_EDGE ( 'NONE', *, *, #6749, .T. ) ;
#39006=AXIS2_PLACEMENT_3D ( 'NONE', #65336, #38075, #65765 ) ;
#39028=AXIS2_PLACEMENT_3D ( 'NONE', #87308, #82303, #59572 ) ;
#39029=LINE ( 'NONE', #58574, #41827 ) ;
#39033=CARTESIAN_POINT ( 'NONE',  ( -130.2060295542616757, 90.93932679091003024, -9.571439627454301657 ) ) ;
#39048=EDGE_CURVE ( 'NONE', #26574, #43857, #34488, .T. ) ;
#39066=LINE ( 'NONE', #12265, #73527 ) ;
#39074=CARTESIAN_POINT ( 'NONE',  ( -83.52531662946618951, 87.03008507238368452, 100.3414980266876739 ) ) ;
#39092=CARTESIAN_POINT ( 'NONE',  ( 69.72411017813010403, 127.0000000000000000, -69.72411017812979139 ) ) ;
#39093=VECTOR ( 'NONE', #74632, 1000.000000000000000 ) ;
#39105=DIRECTION ( 'NONE',  ( 0.000000000000000000, 0.000000000000000000, 1.000000000000000000 ) ) ;
#39112=FILL_AREA_STYLE_COLOUR ( '', #58721 ) ;
#39114=AXIS2_PLACEMENT_3D ( 'NONE', #16783, #60659, #88398 ) ;
#39120=LINE ( 'NONE', #72318, #76356 ) ;
#39166=ORIENTED_EDGE ( 'NONE', *, *, #76284, .F. ) ;
#39192=DIRECTION ( 'NONE',  ( 0.000000000000000000, 1.000000000000000000, 0.000000000000000000 ) ) ;
#39214=CARTESIAN_POINT ( 'NONE',  ( -12.27293249669208919, 79.25788962028573792, 117.9191036749242301 ) ) ;
#39218=AXIS2_PLACEMENT_3D ( 'NONE', #75486, #53656, #6005 ) ;
#39264=ADVANCED_FACE ( 'NONE', ( #30766, #86186 ), #67068, .T. ) ;
#39265=CARTESIAN_POINT ( 'NONE',  ( -11.02155491792549391, 88.91427639974091335, -118.0434862571549957 ) ) ;
#39297=ORIENTED_EDGE ( 'NONE', *, *, #18249, .F. ) ;
#39301=CARTESIAN_POINT ( 'NONE',  ( 31.75000000000000000, 111.1250000000000000, 3.174999999999999822 ) ) ;
#39305=CARTESIAN_POINT ( 'NONE',  ( 88.44471653959712398, 93.33860577356861654, 78.95047879920433331 ) ) ;
#39309=EDGE_LOOP ( 'NONE', ( #56107, #35370 ) ) ;
#39316=LINE ( 'NONE', #67024, #6884 ) ;
#39328=VECTOR ( 'NONE', #55047, 1000.000000000000000 ) ;
#39341=DIRECTION ( 'NONE',  ( 0.000000000000000000, 0.000000000000000000, -1.000000000000000000 ) ) ;
#39347=VERTEX_POINT ( 'NONE', #66615 ) ;
#39382=CARTESIAN_POINT ( 'NONE',  ( 5.624702496966087928, 93.94413577832827400, -130.4352985349313201 ) ) ;
#39395=LINE ( 'NONE', #46187, #34038 ) ;
#39408=CARTESIAN_POINT ( 'NONE',  ( 117.9083627453487821, 85.43299024555679466, -12.37536754217405033 ) ) ;
#39413=AXIS2_PLACEMENT_3D ( 'NONE', #34941, #15862, #28575 ) ;
#39422=VECTOR ( 'NONE', #35334, 1000.000000000000000 ) ;
#39447=ADVANCED_FACE ( 'NONE', ( #88870 ), #268, .T. ) ;
#39451=B_SPLINE_CURVE_WITH_KNOTS ( 'NONE', 3,
 ( #75324, #5844, #62129, #33968, #12650, #55732, #89862, #27612, #26271, #83052, #42125, #69852, #68059, #20804, #26707, #89408, #7623, #53947, #27166, #77558, #15788, #43463, #49384, #8071, #28967 ),
 .UNSPECIFIED., .F., .F.,
 ( 4, 2, 2, 2, 2, 2, 2, 2, 2, 1, 2, 2, 4 ),
 ( 6.610103225985008611E-19, 0.002483982529268030041, 0.003725973793902044844, 0.004967965058536060081, 0.007451947587804091423, 0.008693938852438104492, 0.009935930117072118428, 0.01241991264634014977, 0.01366190391097416197, 0.01490389517560817417, 0.01614588644024218464, 0.01738787770487619858, 0.01987186023414422298 ),
 .UNSPECIFIED. ) ;
#39465=LINE ( 'NONE', #53509, #38788 ) ;
#39475=ORIENTED_EDGE ( 'NONE', *, *, #14262, .F. ) ;
#39486=CARTESIAN_POINT ( 'NONE',  ( -130.4513346304067909, 94.12569442554141119, -5.240856348472988202 ) ) ;
#39520=CARTESIAN_POINT ( 'NONE',  ( 0.000000000000000000, 125.7300000000000040, 0.000000000000000000 ) ) ;
#39584=ORIENTED_EDGE ( 'NONE', *, *, #16374, .T. ) ;
#39588=DIRECTION ( 'NONE',  ( 0.000000000000000000, 1.000000000000000000, 0.000000000000000000 ) ) ;
#39590=CARTESIAN_POINT ( 'NONE',  ( 1.598849875094818280E-14, 61.59999999999999432, -130.5560000000000116 ) ) ;
#39605=PLANE ( 'NONE',  #76653 ) ;
#39612=PLANE ( 'NONE',  #39633 ) ;
#39616=EDGE_CURVE ( 'NONE', #19496, #53446, #18046, .T. ) ;
#39633=AXIS2_PLACEMENT_3D ( 'NONE', #73700, #10575, #31907 ) ;
#39641=CARTESIAN_POINT ( 'NONE',  ( -93.48535127324140603, 69.93117631934791234, -91.13743891206647163 ) ) ;
#39670=ORIENTED_EDGE ( 'NONE', *, *, #50811, .T. ) ;
#39679=DIRECTION ( 'NONE',  ( 0.000000000000000000, 1.000000000000000000, 0.000000000000000000 ) ) ;
#39725=EDGE_CURVE ( 'NONE', #59751, #9320, #49299, .T. ) ;
#39726=CARTESIAN_POINT ( 'NONE',  ( -75.37281393334444601, 76.91656954603718077, 91.51265874544296253 ) ) ;
#39731=ORIENTED_EDGE ( 'NONE', *, *, #22843, .T. ) ;
#39738=FACE_OUTER_BOUND ( 'NONE', #2788, .T. ) ;
#39740=CARTESIAN_POINT ( 'NONE',  ( 12.70000000000000107, 82.54999999999999716, -129.9368274816650910 ) ) ;
#39749=CARTESIAN_POINT ( 'NONE',  ( -95.16508291382886853, 94.58014758961630264, -89.37916159652625936 ) ) ;
#39809=CARTESIAN_POINT ( 'NONE',  ( 1.663881452865401345, 95.14749909259209915, -130.5460625349953148 ) ) ;
#39815=EDGE_LOOP ( 'NONE', ( #29372, #11321 ) ) ;
#39816=CIRCLE ( 'NONE', #54327, 9.525000000000000355 ) ;
#39832=EDGE_CURVE ( 'NONE', #69459, #37218, #57200, .T. ) ;
#39841=DIRECTION ( 'NONE',  ( 1.000000000000000000, 0.000000000000000000, 0.000000000000000000 ) ) ;
#39847=CARTESIAN_POINT ( 'NONE',  ( 117.8738102209309204, 83.38952084682853183, -12.69999999999877005 ) ) ;
#39917=DIRECTION ( 'NONE',  ( 0.000000000000000000, 0.000000000000000000, -1.000000000000000000 ) ) ;
#39921=ORIENTED_EDGE ( 'NONE', *, *, #58303, .T. ) ;
#39923=DIRECTION ( 'NONE',  ( 0.000000000000000000, 1.000000000000000000, 0.000000000000000000 ) ) ;
#39924=CARTESIAN_POINT ( 'NONE',  ( -130.4942851453020296, 94.60320878023492241, -4.086962795941524007 ) ) ;
#39938=CARTESIAN_POINT ( 'NONE',  ( 82.89895571708365196, 82.54999999999999716, -100.8594679592203818 ) ) ;
#39946=EDGE_LOOP ( 'NONE', ( #50616, #50068 ) ) ;
#39948=VECTOR ( 'NONE', #62422, 1000.000000000000114 ) ;
#39984=DIRECTION ( 'NONE',  ( 0.000000000000000000, 0.000000000000000000, 1.000000000000000000 ) ) ;
#39986=CARTESIAN_POINT ( 'NONE',  ( 0.000000000000000000, 127.0000000000000000, -103.1875000000000000 ) ) ;
#40006=CARTESIAN_POINT ( 'NONE',  ( 130.0580535164677656, 88.17609398443094904, 11.39345613591001793 ) ) ;
#40018=CIRCLE ( 'NONE', #25499, 7.143750000000004263 ) ;
#40036=FILL_AREA_STYLE_COLOUR ( '', #75374 ) ;
#40044=DIRECTION ( 'NONE',  ( 0.000000000000000000, 0.000000000000000000, 1.000000000000000000 ) ) ;
#40061=EDGE_CURVE ( 'NONE', #55274, #19496, #19267, .T. ) ;
#40063=CARTESIAN_POINT ( 'NONE',  ( 74.36911441044796334, 82.54999999999999716, -92.32962665258483526 ) ) ;
#40068=VERTEX_POINT ( 'NONE', #53300 ) ;
#40074=AXIS2_PLACEMENT_3D ( 'NONE', #40191, #82909, #67913 ) ;
#40077=VECTOR ( 'NONE', #42309, 1000.000000000000000 ) ;
#40079=PLANE ( 'NONE',  #67847 ) ;
#40086=VERTEX_POINT ( 'NONE', #75578 ) ;
#40088=CARTESIAN_POINT ( 'NONE',  ( -91.71670967179979073, 69.85063703626885001, -92.91726854070125796 ) ) ;
#40096=EDGE_CURVE ( 'NONE', #43857, #26574, #86267, .T. ) ;
#40113=PLANE ( 'NONE',  #15492 ) ;
#40128=DIRECTION ( 'NONE',  ( 0.000000000000000000, 0.000000000000000000, 1.000000000000000000 ) ) ;
#40134=EDGE_CURVE ( 'NONE', #10599, #76633, #82297, .T. ) ;
#40142=CARTESIAN_POINT ( 'NONE',  ( -72.96458098368600531, 127.0000000000000000, -80.90208098368781009 ) ) ;
#40171=CYLINDRICAL_SURFACE ( 'NONE', #22413, 7.143749999999999822 ) ;
#40173=CARTESIAN_POINT ( 'NONE',  ( 0.000000000000000000, 127.0000000000000000, 0.000000000000000000 ) ) ;
#40179=ORIENTED_EDGE ( 'NONE', *, *, #82123, .F. ) ;
#40183=DIRECTION ( 'NONE',  ( 0.000000000000000000, 0.000000000000000000, 1.000000000000000000 ) ) ;
#40191=CARTESIAN_POINT ( 'NONE',  ( -103.1875000000000000, 117.4749999999999943, -1.080832317973422076E-12 ) ) ;
#40193=CARTESIAN_POINT ( 'NONE',  ( -82.97845804870345887, 84.21348395916258767, -100.7940789023224823 ) ) ;
#40195=DIRECTION ( 'NONE',  ( 0.000000000000000000, 1.000000000000000000, 0.000000000000000000 ) ) ;
#40201=FACE_OUTER_BOUND ( 'NONE', #80189, .T. ) ;
#40213=CARTESIAN_POINT ( 'NONE',  ( 69.72411017812960665, 120.6499999999999915, 69.72411017813040246 ) ) ;
#40219=DIRECTION ( 'NONE',  ( 0.000000000000000000, 0.000000000000000000, -1.000000000000000000 ) ) ;
#40233=CARTESIAN_POINT ( 'NONE',  ( 130.2266331669276838, 73.86195533656251655, -9.272499861614344141 ) ) ;
#40242=DIRECTION ( 'NONE',  ( 0.000000000000000000, 0.000000000000000000, -1.000000000000000000 ) ) ;
#40250=CARTESIAN_POINT ( 'NONE',  ( 72.96458098368650269, 127.0000000000000000, 65.82083098368730134 ) ) ;
#40268=DIRECTION ( 'NONE',  ( 1.000000000000000000, 0.000000000000000000, 0.000000000000000000 ) ) ;
#40274=CIRCLE ( 'NONE', #28673, 7.143750000000004263 ) ;
#40277=VERTEX_POINT ( 'NONE', #53983 ) ;
#40302=DIRECTION ( 'NONE',  ( 0.000000000000000000, 1.000000000000000000, 0.000000000000000000 ) ) ;
#40327=VECTOR ( 'NONE', #78301, 1000.000000000000000 ) ;
#40332=ORIENTED_EDGE ( 'NONE', *, *, #63219, .T. ) ;
#40342=LINE ( 'NONE', #55733, #3968 ) ;
#40369=AXIS2_PLACEMENT_3D ( 'NONE', #41788, #20925, #48594 ) ;
#40375=FACE_OUTER_BOUND ( 'NONE', #7133, .T. ) ;
#40378=CARTESIAN_POINT ( 'NONE',  ( 0.000000000000000000, 117.4749999999999943, -103.1875000000000000 ) ) ;
#40379=CARTESIAN_POINT ( 'NONE',  ( -130.0906791124283473, 88.91243380484085890, 11.02261862230878720 ) ) ;
#40384=EDGE_LOOP ( 'NONE', ( #40621, #1786, #27871, #78128 ) ) ;
#40390=DIRECTION ( 'NONE',  ( 0.000000000000000000, -1.000000000000000000, 0.000000000000000000 ) ) ;
#40393=DIRECTION ( 'NONE',  ( -0.7071067811865436870, 0.000000000000000000, -0.7071067811865514585 ) ) ;
#40412=CARTESIAN_POINT ( 'NONE',  ( 103.1875000000000000, 127.0000000000000000, 3.602774393244745134E-13 ) ) ;
#40420=LINE ( 'NONE', #87681, #21164 ) ;
#40421=CARTESIAN_POINT ( 'NONE',  ( -118.5129862669514580, 94.84303900880915705, -3.295572367532775715 ) ) ;
#40430=VERTEX_POINT ( 'NONE', #6759 ) ;
#40449=EDGE_CURVE ( 'NONE', #87834, #9197, #55332, .T. ) ;
#40450=FACE_OUTER_BOUND ( 'NONE', #7014, .T. ) ;
#40458=CARTESIAN_POINT ( 'NONE',  ( 130.3279567413621862, 92.64985122628465319, 7.743850073004674428 ) ) ;
#40471=CARTESIAN_POINT ( 'NONE',  ( -9.554664674393775314, 74.17305037928137779, -130.2061759407760633 ) ) ;
#40472=DIRECTION ( 'NONE',  ( 0.000000000000000000, 0.000000000000000000, 1.000000000000000000 ) ) ;
#40480=VERTEX_POINT ( 'NONE', #391 ) ;
#40484=CARTESIAN_POINT ( 'NONE',  ( -72.96458098368600531, 117.4749999999999943, -65.82083098368781293 ) ) ;
#40489=CARTESIAN_POINT ( 'NONE',  ( 69.72411017812960665, 120.6499999999999915, 69.72411017813040246 ) ) ;
#40505=CARTESIAN_POINT ( 'NONE',  ( 3.174999999999889688, 111.1250000000000000, 31.75000000000000000 ) ) ;
#40544=CARTESIAN_POINT ( 'NONE',  ( -72.96458098368751166, 117.4749999999999943, 72.96458098368620426 ) ) ;
#40548=DIRECTION ( 'NONE',  ( 0.7071067811865536790, 0.000000000000000000, -0.7071067811865413555 ) ) ;
#40556=CYLINDRICAL_SURFACE ( 'NONE', #27440, 12.70000000000000107 ) ;
#40574=EDGE_CURVE ( 'NONE', #42410, #53519, #76431, .T. ) ;
#40598=DIRECTION ( 'NONE',  ( 0.000000000000000000, 0.000000000000000000, 1.000000000000000000 ) ) ;
#40614=LINE ( 'NONE', #46959, #63816 ) ;
#40621=ORIENTED_EDGE ( 'NONE', *, *, #79860, .T. ) ;
#40634=VECTOR ( 'NONE', #29599, 1000.000000000000000 ) ;
#40653=CARTESIAN_POINT ( 'NONE',  ( -91.73195104381140652, 95.23006786499111342, -92.89936586972014254 ) ) ;
#40659=ORIENTED_EDGE ( 'NONE', *, *, #61465, .F. ) ;
#40672=EDGE_LOOP ( 'NONE', ( #23567, #63537, #46148, #64373 ) ) ;
#40673=EDGE_LOOP ( 'NONE', ( #15618, #65330, #11661, #71691 ) ) ;
#40677=EDGE_CURVE ( 'NONE', #62184, #36627, #22647, .T. ) ;
#40683=EDGE_CURVE ( 'NONE', #2544, #54712, #50778, .T. ) ;
#40740=DIRECTION ( 'NONE',  ( 0.000000000000000000, 0.000000000000000000, 1.000000000000000000 ) ) ;
#40746=LINE ( 'NONE', #68470, #36106 ) ;
#40750=EDGE_CURVE ( 'NONE', #35831, #24268, #79275, .T. ) ;
#40757=ADVANCED_FACE ( 'NONE', ( #62511 ), #55661, .F. ) ;
#40758=AXIS2_PLACEMENT_3D ( 'NONE', #82714, #41779, #63140 ) ;
#40760=ADVANCED_FACE ( 'NONE', ( #82982, #69335 ), #47521, .F. ) ;
#40772=CARTESIAN_POINT ( 'NONE',  ( -11.39384497175739064, 88.17529471328431612, 118.0073914794113819 ) ) ;
#40781=AXIS2_PLACEMENT_3D ( 'NONE', #84975, #28640, #21846 ) ;
#40821=CARTESIAN_POINT ( 'NONE',  ( -130.5401660959919354, 95.08644067748863904, -2.073645319394354036 ) ) ;
#40830=CARTESIAN_POINT ( 'NONE',  ( 90.25311968877677771, 94.92443974548206143, -94.33669211993671411 ) ) ;
#40835=CARTESIAN_POINT ( 'NONE',  ( -4.880114330320866500, 70.80325516146916698, -118.4573640576558660 ) ) ;
#40870=ORIENTED_EDGE ( 'NONE', *, *, #3907, .T. ) ;
#40900=CARTESIAN_POINT ( 'NONE',  ( 130.2872239869710427, 92.11674985319544362, -8.393624206580007296 ) ) ;
#40911=CARTESIAN_POINT ( 'NONE',  ( -8.398107354775891764, 72.98722500879387098, -130.2869324835649536 ) ) ;
#40940=CARTESIAN_POINT ( 'NONE',  ( 12.69999999999999929, 81.71107837960109066, 117.8738102209307499 ) ) ;
#40959=CARTESIAN_POINT ( 'NONE',  ( 74.15067561874269586, 120.6499999999999915, -68.53801554307419508 ) ) ;
#40960=DIRECTION ( 'NONE',  ( -0.000000000000000000, 1.000000000000000000, 0.000000000000000000 ) ) ;
#40987=CARTESIAN_POINT ( 'NONE',  ( -89.08909376920014722, 70.66229531820913223, -95.43663006862824716 ) ) ;
#41002=CARTESIAN_POINT ( 'NONE',  ( 0.000000000000000000, 101.5999999999999943, 130.5560000000000116 ) ) ;
#41005=DIRECTION ( 'NONE',  ( 0.2588190451025154659, 0.000000000000000000, 0.9659258262890696445 ) ) ;
#41036=CARTESIAN_POINT ( 'NONE',  ( 0.000000000000000000, 95.25000000000000000, 0.000000000000000000 ) ) ;
#41048=DIRECTION ( 'NONE',  ( 0.9659258262890704216, 0.000000000000000000, -0.2588190451025129124 ) ) ;
#41056=CARTESIAN_POINT ( 'NONE',  ( 129.9388103550932669, 83.38002811471483255, 12.67976361810990760 ) ) ;
#41058=EDGE_LOOP ( 'NONE', ( #18009, #15693, #81596, #26912 ) ) ;
#41071=CARTESIAN_POINT ( 'NONE',  ( -86.12934247706235169, 70.27763793881260312, 81.47036787067852970 ) ) ;
#41075=EDGE_LOOP ( 'NONE', ( #18048, #20753 ) ) ;
#41076=ORIENTED_EDGE ( 'NONE', *, *, #52461, .T. ) ;
#41078=EDGE_CURVE ( 'NONE', #59338, #61529, #66977, .T. ) ;
#41093=CARTESIAN_POINT ( 'NONE',  ( -84.90178614994256634, 90.29814575435203494, -99.18048580889426091 ) ) ;
#41096=AXIS2_PLACEMENT_3D ( 'NONE', #77477, #83401, #7096 ) ;
#41097=AXIS2_PLACEMENT_3D ( 'NONE', #81718, #26282, #19922 ) ;
#41117=ORIENTED_EDGE ( 'NONE', *, *, #81409, .F. ) ;
#41128=CARTESIAN_POINT ( 'NONE',  ( -130.0906838859329184, 76.18750001922980175, 11.02255322708127849 ) ) ;
#41148=CARTESIAN_POINT ( 'NONE',  ( -103.1875000000000000, 101.5999999999999943, -1.080832317973422076E-12 ) ) ;
#41152=CARTESIAN_POINT ( 'NONE',  ( -76.20505178924278766, 120.6499999999999915, -76.20505178924469192 ) ) ;
#41169=CYLINDRICAL_SURFACE ( 'NONE', #327, 7.143750000000004263 ) ;
#41185=AXIS2_PLACEMENT_3D ( 'NONE', #38027, #11205, #52947 ) ;
#41191=VECTOR ( 'NONE', #11711, 1000.000000000000227 ) ;
#41196=ORIENTED_EDGE ( 'NONE', *, *, #44023, .F. ) ;
#41209=CARTESIAN_POINT ( 'NONE',  ( -11.57394144444448436, 87.79471777913512653, 117.9898073157514489 ) ) ;
#41224=DIRECTION ( 'NONE',  ( -0.7071067811865460184, 0.000000000000000000, 0.7071067811865489050 ) ) ;
#41261=CARTESIAN_POINT ( 'NONE',  ( 86.68128281353467912, 72.47310549519058043, 97.62852612868820756 ) ) ;
#41263=B_SPLINE_CURVE_WITH_KNOTS ( 'NONE', 3,
 ( #75051, #38285, #52327, #11023, #31912, #65982, #80092, #73243, #38728, #66430, #4219, #59606, #45970, #25104, #28690, #75946, #28227, #7354, #61405, #14625, #48211, #91, #49109, #82333, #49559, #985, #83219, #35043, #68242, #55468, #42297, #63208, #54567, #62305, #89135, #6025, #13719, #55919, #6454, #70031, #26892, #82782, #12836, #27787, #62753, #75503, #61844, #34146 ),
 .UNSPECIFIED., .F., .F.,
 ( 4, 2, 2, 2, 2, 2, 2, 2, 2, 1, 2, 2, 2, 2, 2, 2, 2, 2, 2, 2, 2, 1, 2, 2, 4 ),
 ( 0.05959919981814693762, 0.06208168506169071260, 0.06332292768346260703, 0.06456417030523449452, 0.06704665554877825562, 0.06828789817055014311, 0.06952914079232203060, 0.07201162603586583333, 0.07325286865763772082, 0.07449411127940962218, 0.07573535390118150967, 0.07697659652295341104, 0.07945908176649719989, 0.08194156701004098875, 0.08318280963181286236, 0.08442405225358473597, 0.08690653749712842768, 0.08814778011890027354, 0.08938902274067211939, 0.09187150798421574172, 0.09311275060598753206, 0.09435399322775930853, 0.09559523584953109887, 0.09683647847130288921, 0.09931896371484645603 ),
 .UNSPECIFIED. ) ;
#41269=VERTEX_POINT ( 'NONE', #67874 ) ;
#41270=DIRECTION ( 'NONE',  ( -0.000000000000000000, 1.000000000000000000, -0.000000000000000000 ) ) ;
#41272=CARTESIAN_POINT ( 'NONE',  ( 86.67213519546683642, 92.64237678566777845, -97.63858630140124717 ) ) ;
#41274=ADVANCED_FACE ( 'NONE', ( #27428 ), #75138, .F. ) ;
#41287=FACE_OUTER_BOUND ( 'NONE', #87214, .T. ) ;
#41293=EDGE_CURVE ( 'NONE', #12282, #30848, #34686, .T. ) ;
#41300=DIRECTION ( 'NONE',  ( 0.9659258262890670910, 0.000000000000000000, 0.2588190451025250693 ) ) ;
#41303=CARTESIAN_POINT ( 'NONE',  ( 90.66736180499694342, 74.80137413886471620, -76.38829385798599958 ) ) ;
#41321=CARTESIAN_POINT ( 'NONE',  ( 91.24829632406253666, 88.91144712388910420, -75.69222284415423019 ) ) ;
#41329=ORIENTED_EDGE ( 'NONE', *, *, #45242, .T. ) ;
#41374=CARTESIAN_POINT ( 'NONE',  ( 99.63271100832268701, 75.84295037288960373, -84.36969927706125816 ) ) ;
#41383=CARTESIAN_POINT ( 'NONE',  ( 7.760001168987765929, 72.46196594926868784, 118.3038028359265894 ) ) ;
#41388=DIRECTION ( 'NONE',  ( 0.000000000000000000, 1.000000000000000000, 0.000000000000000000 ) ) ;
#41394=DIRECTION ( 'NONE',  ( 0.000000000000000000, 1.000000000000000000, 0.000000000000000000 ) ) ;
#41400=DIRECTION ( 'NONE',  ( 0.000000000000000000, 1.000000000000000000, 0.000000000000000000 ) ) ;
#41448=VERTEX_POINT ( 'NONE', #81811 ) ;
#41460=CARTESIAN_POINT ( 'NONE',  ( 0.000000000000000000, 127.0000000000000000, -103.1875000000000000 ) ) ;
#41468=VERTEX_POINT ( 'NONE', #68173 ) ;
#41479=CARTESIAN_POINT ( 'NONE',  ( 12.29197255332129579, 85.84955738763291322, -117.9171711396470386 ) ) ;
#41497=VECTOR ( 'NONE', #32102, 1000.000000000000000 ) ;
#41509=CARTESIAN_POINT ( 'NONE',  ( -91.25368348339000590, 76.20320268897033600, 75.68572508987546144 ) ) ;
#41519=DIRECTION ( 'NONE',  ( -1.000000000000000000, 0.000000000000000000, -6.982966722218760189E-15 ) ) ;
#41532=CARTESIAN_POINT ( 'NONE',  ( -86.19814306825452377, 92.12504059357189590, -98.05663017059063691 ) ) ;
#41533=CARTESIAN_POINT ( 'NONE',  ( 0.000000000000000000, 124.9679999999999893, 0.000000000000000000 ) ) ;
#41540=ORIENTED_EDGE ( 'NONE', *, *, #2221, .T. ) ;
#41541=FACE_OUTER_BOUND ( 'NONE', #51879, .T. ) ;
#41556=EDGE_LOOP ( 'NONE', ( #73650, #55713 ) ) ;
#41562=EDGE_CURVE ( 'NONE', #75590, #83000, #82265, .T. ) ;
#41570=CARTESIAN_POINT ( 'NONE',  ( 129.9778716492872945, 79.25971567868506895, 12.27341459163532811 ) ) ;
#41581=DIRECTION ( 'NONE',  ( 0.000000000000000000, 0.000000000000000000, -1.000000000000000000 ) ) ;
#41585=DIRECTION ( 'NONE',  ( 0.000000000000000000, 1.000000000000000000, 0.000000000000000000 ) ) ;
#41588=VERTEX_POINT ( 'NONE', #6831 ) ;
#41607=AXIS2_PLACEMENT_3D ( 'NONE', #50082, #56449, #76463 ) ;
#41617=CARTESIAN_POINT ( 'NONE',  ( 3.968749999999215294, 120.6499999999999915, 105.4788588808464027 ) ) ;
#41621=EDGE_LOOP ( 'NONE', ( #63795, #83164, #18108, #83383 ) ) ;
#41631=CARTESIAN_POINT ( 'NONE',  ( 72.96458098368650269, 127.0000000000000000, 80.10833098368729566 ) ) ;
#41651=DIRECTION ( 'NONE',  ( 0.000000000000000000, 0.000000000000000000, -1.000000000000000000 ) ) ;
#41653=CARTESIAN_POINT ( 'NONE',  ( -0.4144849534825577608, 95.25000000000000000, 118.5559999999999974 ) ) ;
#41658=LINE ( 'NONE', #20354, #3360 ) ;
#41662=PLANE ( 'NONE',  #87618 ) ;
#41664=EDGE_CURVE ( 'NONE', #83340, #58908, #42676, .T. ) ;
#41674=EDGE_CURVE ( 'NONE', #81089, #8309, #58115, .T. ) ;
#41707=CARTESIAN_POINT ( 'NONE',  ( 99.17101862044538052, 74.81660785136577374, 84.91200770515706608 ) ) ;
#41714=EDGE_LOOP ( 'NONE', ( #29603, #42697, #60281, #53324 ) ) ;
#41722=DIRECTION ( 'NONE',  ( 0.000000000000000000, 1.000000000000000000, 0.000000000000000000 ) ) ;
#41735=CARTESIAN_POINT ( 'NONE',  ( 0.000000000000000000, 127.0000000000000000, 0.000000000000000000 ) ) ;
#41741=CARTESIAN_POINT ( 'NONE',  ( -90.32698471909129978, 90.93965867633430378, 76.79137032886123393 ) ) ;
#41749=CARTESIAN_POINT ( 'NONE',  ( 81.76234319299427966, 70.17658267799284033, -85.85227416678121415 ) ) ;
#41755=ORIENTED_EDGE ( 'NONE', *, *, #2698, .F. ) ;
#41767=CARTESIAN_POINT ( 'NONE',  ( 78.95047879920406331, 93.33860577356860233, -88.44471653959740820 ) ) ;
#41778=LINE ( 'NONE', #51275, #22598 ) ;
#41779=DIRECTION ( 'NONE',  ( 0.000000000000000000, 1.000000000000000000, 0.000000000000000000 ) ) ;
#41785=ORIENTED_EDGE ( 'NONE', *, *, #43636, .T. ) ;
#41788=CARTESIAN_POINT ( 'NONE',  ( 68.91674821478362389, 82.54999999999999716, 68.91674821478530077 ) ) ;
#41803=CARTESIAN_POINT ( 'NONE',  ( -82.64146475440728068, 69.93366089391892615, -85.00925061400963045 ) ) ;
#41812=EDGE_LOOP ( 'NONE', ( #22093, #52043, #87050, #70763 ) ) ;
#41816=CARTESIAN_POINT ( 'NONE',  ( 99.18073718829404584, 74.80151635532864418, -84.90151352399627172 ) ) ;
#41819=ORIENTED_EDGE ( 'NONE', *, *, #17984, .T. ) ;
#41824=CARTESIAN_POINT ( 'NONE',  ( 4.880114330320866500, 70.80325516146916698, 118.4573640576558660 ) ) ;
#41827=VECTOR ( 'NONE', #32211, 1000.000000000000114 ) ;
#41847=AXIS2_PLACEMENT_3D ( 'NONE', #34145, #34601, #28689 ) ;
#41856=LINE ( 'NONE', #7365, #77777 ) ;
#41862=ORIENTED_EDGE ( 'NONE', *, *, #1168, .T. ) ;
#41870=VECTOR ( 'NONE', #50450, 1000.000000000000000 ) ;
#41895=DIRECTION ( 'NONE',  ( 0.000000000000000000, 0.000000000000000000, 1.000000000000000000 ) ) ;
#41900=ADVANCED_FACE ( 'NONE', ( #65381 ), #11755, .F. ) ;
#41937=DIRECTION ( 'NONE',  ( 0.000000000000000000, 1.000000000000000000, 0.000000000000000000 ) ) ;
#41943=CIRCLE ( 'NONE', #86901, 7.937500000000000000 ) ;
#41948=AXIS2_PLACEMENT_3D ( 'NONE', #54498, #20473, #67714 ) ;
#41955=CARTESIAN_POINT ( 'NONE',  ( -7.941868552260229762E-13, 120.6499999999999915, 107.7702177616926065 ) ) ;
#41967=DIRECTION ( 'NONE',  ( 0.000000000000000000, 1.000000000000000000, 0.000000000000000000 ) ) ;
#41972=DIRECTION ( 'NONE',  ( 0.000000000000000000, 1.000000000000000000, 0.000000000000000000 ) ) ;
#41982=CARTESIAN_POINT ( 'NONE',  ( 4.879617406430184268, 70.80304812169737261, 130.4664555583633501 ) ) ;
#41983=CARTESIAN_POINT ( 'NONE',  ( -98.82361644294738312, 90.93081950567959382, -85.31607583734439970 ) ) ;
#41991=VERTEX_POINT ( 'NONE', #58829 ) ;
#42025=CARTESIAN_POINT ( 'NONE',  ( 130.5150461639146044, 70.27756284692561906, 3.294108455004394642 ) ) ;
#42035=CARTESIAN_POINT ( 'NONE',  ( 71.77848634863079269, 127.0000000000000000, 77.39114642429989033 ) ) ;
#42042=FACE_BOUND ( 'NONE', #80231, .T. ) ;
#42047=DIRECTION ( 'NONE',  ( 0.000000000000000000, 0.000000000000000000, 1.000000000000000000 ) ) ;
#42048=CARTESIAN_POINT ( 'NONE',  ( -72.96458098368751166, 127.0000000000000000, 80.10833098368618721 ) ) ;
#42080=LINE ( 'NONE', #62537, #43443 ) ;
#42081=LINE ( 'NONE', #14859, #20189 ) ;
#42083=CARTESIAN_POINT ( 'NONE',  ( 100.3414980266867929, 87.03008507238371294, 83.52531662946728375 ) ) ;
#42089=DIRECTION ( 'NONE',  ( 1.092739197465705130E-14, 0.000000000000000000, -1.000000000000000000 ) ) ;
#42096=CARTESIAN_POINT ( 'NONE',  ( -72.96458098368600531, 127.0000000000000000, -72.96458098368781009 ) ) ;
#42100=EDGE_CURVE ( 'NONE', #46818, #55274, #11336, .T. ) ;
#42117=CARTESIAN_POINT ( 'NONE',  ( -117.9439354154379203, 78.46407912418312947, -12.03195559056875297 ) ) ;
#42119=ORIENTED_EDGE ( 'NONE', *, *, #4083, .T. ) ;
#42125=CARTESIAN_POINT ( 'NONE',  ( 7.736705052999859333, 72.46990138899384704, -118.3037342042693325 ) ) ;
#42138=DIRECTION ( 'NONE',  ( 0.000000000000000000, 0.000000000000000000, 1.000000000000000000 ) ) ;
#42144=CARTESIAN_POINT ( 'NONE',  ( 0.000000000000000000, 101.5999999999999943, 0.000000000000000000 ) ) ;
#42147=AXIS2_PLACEMENT_3D ( 'NONE', #63144, #70873, #34981 ) ;
#42165=AXIS2_PLACEMENT_3D ( 'NONE', #3815, #67363, #45560 ) ;
#42168=ORIENTED_EDGE ( 'NONE', *, *, #17189, .F. ) ;
#42171=CARTESIAN_POINT ( 'NONE',  ( 0.000000000000000000, 92.07499999999998863, 0.000000000000000000 ) ) ;
#42175=CARTESIAN_POINT ( 'NONE',  ( -31.75000000000000000, 104.3431970271541900, -3.175000000000219647 ) ) ;
#42189=EDGE_CURVE ( 'NONE', #70164, #57201, #55164, .T. ) ;
#42197=CARTESIAN_POINT ( 'NONE',  ( -75.67533895324345394, 88.91291927174617626, 91.26325766987484656 ) ) ;
#42207=CARTESIAN_POINT ( 'NONE',  ( 12.70000000000000107, 82.54999999999999716, 97.46299999999996544 ) ) ;
#42208=DIRECTION ( 'NONE',  ( 1.000000000000000000, 0.000000000000000000, 3.491483361109385222E-15 ) ) ;
#42214=LINE ( 'NONE', #3, #5400 ) ;
#42221=CARTESIAN_POINT ( 'NONE',  ( 74.89049941105147923, 86.63388195152282378, -91.90730674524651533 ) ) ;
#42229=ORIENTED_EDGE ( 'NONE', *, *, #58147, .T. ) ;
#42258=CARTESIAN_POINT ( 'NONE',  ( -74.89107914305763813, 78.46407912418314368, -91.90683392111100147 ) ) ;
#42265=DIRECTION ( 'NONE',  ( 0.000000000000000000, 1.000000000000000000, 0.000000000000000000 ) ) ;
#42267=CARTESIAN_POINT ( 'NONE',  ( 0.000000000000000000, 82.54999999999999716, 97.46299999999996544 ) ) ;
#42289=VECTOR ( 'NONE', #56801, 1000.000000000000000 ) ;
#42295=LINE ( 'NONE', #15518, #36991 ) ;
#42297=CARTESIAN_POINT ( 'NONE',  ( -96.22129751242485440, 71.14122173980733521, 88.24354053934821707 ) ) ;
#42301=ORIENTED_EDGE ( 'NONE', *, *, #87016, .F. ) ;
#42309=DIRECTION ( 'NONE',  ( -3.491483361109385222E-15, 0.000000000000000000, 1.000000000000000000 ) ) ;
#42318=CARTESIAN_POINT ( 'NONE',  ( -84.36969927706159922, 75.84295037288958952, -99.63271100832238858 ) ) ;
#42319=CARTESIAN_POINT ( 'NONE',  ( -74.38497350661499752, 83.38015080693121206, -92.31685958143614812 ) ) ;
#42338=CARTESIAN_POINT ( 'NONE',  ( -77.39114642430010349, 120.6499999999999915, 71.77848634863050847 ) ) ;
#42341=CARTESIAN_POINT ( 'NONE',  ( 8.391666350164339150, 92.11848141222132824, 118.2600956121756752 ) ) ;
#42357=VECTOR ( 'NONE', #83922, 1000.000000000000000 ) ;
#42374=CARTESIAN_POINT ( 'NONE',  ( -0.8301116440131806051, 95.22976338641703364, 130.5540265925895085 ) ) ;
#42403=CARTESIAN_POINT ( 'NONE',  ( -3.968749999999935163, 120.6499999999999915, -100.8961411191535973 ) ) ;
#42406=CARTESIAN_POINT ( 'NONE',  ( -89.75424775947659839, 73.28361289573329884, 77.45828646618677737 ) ) ;
#42410=VERTEX_POINT ( 'NONE', #2444 ) ;
#42426=ORIENTED_EDGE ( 'NONE', *, *, #58524, .T. ) ;
#42438=ORIENTED_EDGE ( 'NONE', *, *, #71733, .F. ) ;
#42441=ORIENTED_EDGE ( 'NONE', *, *, #9559, .F. ) ;
#42466=CARTESIAN_POINT ( 'NONE',  ( 130.3273007233323710, 72.45841406287409825, -7.755409066831144393 ) ) ;
#42477=EDGE_CURVE ( 'NONE', #6827, #46578, #52026, .T. ) ;
#42502=DIRECTION ( 'NONE',  ( 0.000000000000000000, -1.000000000000000000, 0.000000000000000000 ) ) ;
#42521=VECTOR ( 'NONE', #65726, 1000.000000000000000 ) ;
#42525=CARTESIAN_POINT ( 'NONE',  ( 68.53801554307449351, 127.0000000000000000, -74.15067561874229796 ) ) ;
#42526=AXIS2_PLACEMENT_3D ( 'NONE', #76436, #12886, #41895 ) ;
#42530=FACE_OUTER_BOUND ( 'NONE', #23280, .T. ) ;
#42574=DIRECTION ( 'NONE',  ( 0.000000000000000000, 1.000000000000000000, 0.000000000000000000 ) ) ;
#42576=ADVANCED_FACE ( 'NONE', ( #56378 ), #77291, .F. ) ;
#42583=DIRECTION ( 'NONE',  ( 1.000000000000000000, 0.000000000000000000, 0.000000000000000000 ) ) ;
#42598=CARTESIAN_POINT ( 'NONE',  ( 96.70122665881119417, 71.54617234588346264, 87.71474477836368067 ) ) ;
#42620=EDGE_LOOP ( 'NONE', ( #84521, #71680, #68514, #84407 ) ) ;
#42627=CYLINDRICAL_SURFACE ( 'NONE', #5210, 12.70000000000000107 ) ;
#42631=EDGE_LOOP ( 'NONE', ( #79032, #24351, #49265, #27605 ) ) ;
#42634=CARTESIAN_POINT ( 'NONE',  ( -86.13165781700281798, 94.84303900880912863, 81.47101467905625327 ) ) ;
#42653=DIRECTION ( 'NONE',  ( 0.000000000000000000, 1.000000000000000000, 0.000000000000000000 ) ) ;
#42657=CARTESIAN_POINT ( 'NONE',  ( 83.24211534968729609, 95.24969287062863543, -84.42134122279055930 ) ) ;
#42659=ADVANCED_FACE ( 'NONE', ( #24453 ), #23575, .F. ) ;
#42676=LINE ( 'NONE', #35425, #2596 ) ;
#42681=CARTESIAN_POINT ( 'NONE',  ( -74.15067561874319324, 120.6499999999999915, 68.53801554307369770 ) ) ;
#42697=ORIENTED_EDGE ( 'NONE', *, *, #81812, .T. ) ;
#42712=CARTESIAN_POINT ( 'NONE',  ( 86.67141577317461554, 72.45841406287409825, -97.63922045723883514 ) ) ;
#42732=ORIENTED_EDGE ( 'NONE', *, *, #6009, .F. ) ;
#42734=AXIS2_PLACEMENT_3D ( 'NONE', #77744, #20982, #28225 ) ;
#42752=CARTESIAN_POINT ( 'NONE',  ( -72.96458098368751166, 117.4749999999999943, 65.82083098368619289 ) ) ;
#42758=EDGE_LOOP ( 'NONE', ( #9512, #36167, #89158, #48132 ) ) ;
#42761=CARTESIAN_POINT ( 'NONE',  ( -79.76258624986827783, 93.94553785444264804, -87.71311422381560874 ) ) ;
#42769=SHAPE_REPRESENTATION ( 'Pneumatic Workpiece Fixture Plate', ( #50656 ), #89914 ) ;
#42806=AXIS2_PLACEMENT_3D ( 'NONE', #28217, #6888, #41394 ) ;
#42819=CARTESIAN_POINT ( 'NONE',  ( 3.174999999999879918, 124.5870000000000033, 33.98325472291465132 ) ) ;
#42820=CARTESIAN_POINT ( 'NONE',  ( 0.4144849534825713055, 95.24999999999998579, -118.5559999999999832 ) ) ;
#42822=CARTESIAN_POINT ( 'NONE',  ( -12.29205751230851362, 85.84923025428281562, 129.9761558897302791 ) ) ;
#42824=CARTESIAN_POINT ( 'NONE',  ( -72.96458098368751166, 117.4749999999999943, 65.02708098368620426 ) ) ;
#42825=DIRECTION ( 'NONE',  ( 0.000000000000000000, -1.000000000000000000, 0.000000000000000000 ) ) ;
#42843=ORIENTED_EDGE ( 'NONE', *, *, #45242, .F. ) ;
#42849=CARTESIAN_POINT ( 'NONE',  ( -85.85219768521552908, 70.17671898886891313, 81.76240029069619197 ) ) ;
#42854=EDGE_CURVE ( 'NONE', #23593, #79245, #88019, .T. ) ;
#42865=EDGE_CURVE ( 'NONE', #48000, #24335, #40746, .T. ) ;
#42868=LINE ( 'NONE', #1566, #20228 ) ;
#42872=EDGE_LOOP ( 'NONE', ( #47462, #53032 ) ) ;
#42875=CARTESIAN_POINT ( 'NONE',  ( 10.33379165269208499, 75.15577250977247559, 130.1465911299492006 ) ) ;
#42902=AXIS2_PLACEMENT_3D ( 'NONE', #26155, #46572, #45666 ) ;
#42917=ORIENTED_EDGE ( 'NONE', *, *, #30213, .F. ) ;
#42936=FACE_OUTER_BOUND ( 'NONE', #77189, .T. ) ;
#42972=CARTESIAN_POINT ( 'NONE',  ( 92.90667244829660376, 95.24968527363473925, 91.72735010416711532 ) ) ;
#42974=DIRECTION ( 'NONE',  ( 0.000000000000000000, 0.000000000000000000, -1.000000000000000000 ) ) ;
#42978=ORIENTED_EDGE ( 'NONE', *, *, #88178, .T. ) ;
#42985=AXIS2_PLACEMENT_3D ( 'NONE', #79552, #30050, #65889 ) ;
#43014=CARTESIAN_POINT ( 'NONE',  ( -103.1875000000000000, 127.0000000000000000, -7.143750000001079847 ) ) ;
#43034=LINE ( 'NONE', #57116, #39422 ) ;
#43050=CARTESIAN_POINT ( 'NONE',  ( 100.8594679592200976, 81.71102547120852932, 82.89895571708400723 ) ) ;
#43054=AXIS2_PLACEMENT_3D ( 'NONE', #58797, #19712, #76471 ) ;
#43086=CARTESIAN_POINT ( 'NONE',  ( -90.66710916952438026, 90.29828471680512791, 76.38857008573013729 ) ) ;
#43093=CARTESIAN_POINT ( 'NONE',  ( 88.90442867305986852, 72.22378176823140450, -78.43243611888054545 ) ) ;
#43096=EDGE_CURVE ( 'NONE', #62096, #12394, #20457, .T. ) ;
#43107=FACE_BOUND ( 'NONE', #83608, .T. ) ;
#43111=CARTESIAN_POINT ( 'NONE',  ( 81.46927207886297140, 94.82191660594808980, -86.13037352894103549 ) ) ;
#43146=CARTESIAN_POINT ( 'NONE',  ( 0.000000000000000000, 111.1250000000000000, 0.000000000000000000 ) ) ;
#43168=CARTESIAN_POINT ( 'NONE',  ( 98.05713019660848317, 73.00415124681448731, -86.19613171056641932 ) ) ;
#43182=ORIENTED_EDGE ( 'NONE', *, *, #32220, .F. ) ;
#43208=DIRECTION ( 'NONE',  ( 0.000000000000000000, 1.000000000000000000, 0.000000000000000000 ) ) ;
#43218=CARTESIAN_POINT ( 'NONE',  ( -78.17826422383528495, 92.64969027323469675, -89.13001032377188437 ) ) ;
#43226=CARTESIAN_POINT ( 'NONE',  ( 1.451892259197136103E-14, 61.59999999999999432, -118.5560000000000116 ) ) ;
#43232=CARTESIAN_POINT ( 'NONE',  ( 0.000000000000000000, 61.59999999999999432, 0.000000000000000000 ) ) ;
#43245=VERTEX_POINT ( 'NONE', #70603 ) ;
#43264=PRODUCT_DEFINITION_CONTEXT ( 'detailed design', #86420, 'design' ) ;
#43266=LINE ( 'NONE', #7419, #74672 ) ;
#43273=CARTESIAN_POINT ( 'NONE',  ( -74.15067561874319324, 120.6499999999999915, 68.53801554307369770 ) ) ;
#43274=CIRCLE ( 'NONE', #30197, 7.937500000000000000 ) ;
#43278=DIRECTION ( 'NONE',  ( 0.000000000000000000, 1.000000000000000000, 0.000000000000000000 ) ) ;
#43284=VECTOR ( 'NONE', #18655, 1000.000000000000000 ) ;
#43326=ORIENTED_EDGE ( 'NONE', *, *, #60537, .T. ) ;
#43328=EDGE_CURVE ( 'NONE', #70137, #73627, #42868, .T. ) ;
#43363=DIRECTION ( 'NONE',  ( 0.000000000000000000, 1.000000000000000000, 0.000000000000000000 ) ) ;
#43377=DIRECTION ( 'NONE',  ( 0.7071067811865533459, 0.000000000000000000, -0.7071067811865416886 ) ) ;
#43396=CARTESIAN_POINT ( 'NONE',  ( 2.314288535156699577E-14, 127.0000000000000000, 188.9759999999999991 ) ) ;
#43402=CARTESIAN_POINT ( 'NONE',  ( -77.39114642429849766, 127.0000000000000000, -71.77848634863219957 ) ) ;
#43411=CARTESIAN_POINT ( 'NONE',  ( -72.96458098368600531, 117.4749999999999943, -78.00648098368779415 ) ) ;
#43419=EDGE_LOOP ( 'NONE', ( #31795, #13420, #66340, #47321 ) ) ;
#43424=CARTESIAN_POINT ( 'NONE',  ( 100.8069756963035530, 84.21449860606321636, 82.96293804092898938 ) ) ;
#43438=ADVANCED_BREP_SHAPE_REPRESENTATION ( '', ( #79963, #50656 ), #89914 ) ;
#43443=VECTOR ( 'NONE', #15748, 1000.000000000000000 ) ;
#43463=CARTESIAN_POINT ( 'NONE',  ( 12.37524867428841091, 79.66590588004265783, -117.9083757119989428 ) ) ;
#43476=LINE ( 'NONE', #84854, #28623 ) ;
#43486=VERTEX_POINT ( 'NONE', #36966 ) ;
#43502=ORIENTED_EDGE ( 'NONE', *, *, #24046, .F. ) ;
#43512=DIRECTION ( 'NONE',  ( 0.000000000000000000, 1.000000000000000000, 0.000000000000000000 ) ) ;
#43519=DIRECTION ( 'NONE',  ( 0.000000000000000000, 0.000000000000000000, -1.000000000000000000 ) ) ;
#43522=ORIENTED_EDGE ( 'NONE', *, *, #12894, .F. ) ;
#43536=PLANE ( 'NONE',  #77711 ) ;
#43540=CARTESIAN_POINT ( 'NONE',  ( -92.32962665258560264, 82.54999999999999716, 74.36911441044701121 ) ) ;
#43545=ORIENTED_EDGE ( 'NONE', *, *, #78329, .F. ) ;
#43549=CARTESIAN_POINT ( 'NONE',  ( 97.46299999999982333, 82.54999999999999716, 12.70000000000102069 ) ) ;
#43562=EDGE_CURVE ( 'NONE', #42410, #60191, #8835, .T. ) ;
#43611=DIRECTION ( 'NONE',  ( 0.000000000000000000, 0.000000000000000000, -1.000000000000000000 ) ) ;
#43612=VERTEX_POINT ( 'NONE', #37868 ) ;
#43626=ADVANCED_FACE ( 'NONE', ( #66899 ), #87798, .F. ) ;
#43636=EDGE_CURVE ( 'NONE', #36627, #27899, #32824, .T. ) ;
#43656=CARTESIAN_POINT ( 'NONE',  ( -89.95770503246842509, 94.82199753261677699, 94.61838531165750510 ) ) ;
#43661=VECTOR ( 'NONE', #64986, 1000.000000000000000 ) ;
#43662=EDGE_LOOP ( 'NONE', ( #16925, #15682 ) ) ;
#43706=AXIS2_PLACEMENT_3D ( 'NONE', #68426, #75688, #5755 ) ;
#43707=EDGE_LOOP ( 'NONE', ( #64004, #7570, #81836, #73022 ) ) ;
#43728=CARTESIAN_POINT ( 'NONE',  ( -6.359443759653452766, 93.55095829381066608, 130.4015408541779379 ) ) ;
#43737=AXIS2_PLACEMENT_3D ( 'NONE', #2305, #49975, #43611 ) ;
#43743=ORIENTED_EDGE ( 'NONE', *, *, #8871, .T. ) ;
#43774=LINE ( 'NONE', #30156, #86463 ) ;
#43815=CARTESIAN_POINT ( 'NONE',  ( -130.5149182481443404, 70.27892663483460467, 3.298988752046296380 ) ) ;
#43849=CARTESIAN_POINT ( 'NONE',  ( 0.000000000000000000, 95.25000000000000000, 42.54500000000000171 ) ) ;
#43857=VERTEX_POINT ( 'NONE', #7367 ) ;
#43877=CARTESIAN_POINT ( 'NONE',  ( 93.48397507443749532, 95.16896684734908263, 91.13883569058539535 ) ) ;
#43890=CARTESIAN_POINT ( 'NONE',  ( -72.96458098368751166, 117.4749999999999943, 80.90208098368620426 ) ) ;
#43895=DIRECTION ( 'NONE',  ( 0.000000000000000000, 1.000000000000000000, 0.000000000000000000 ) ) ;
#43899=DIRECTION ( 'NONE',  ( 0.000000000000000000, 0.000000000000000000, 1.000000000000000000 ) ) ;
#43916=CARTESIAN_POINT ( 'NONE',  ( 31.75000000000000000, 111.1250000000000000, -3.174999999999999822 ) ) ;
#43924=CARTESIAN_POINT ( 'NONE',  ( 0.000000000000000000, 111.1250000000000000, 0.000000000000000000 ) ) ;
#43934=EDGE_CURVE ( 'NONE', #64009, #84699, #60855, .T. ) ;
#43941=PLANE ( 'NONE',  #15470 ) ;
#43954=CIRCLE ( 'NONE', #42526, 88.90000000000000568 ) ;
#43960=DIRECTION ( 'NONE',  ( 1.000000000000000000, 0.000000000000000000, 0.000000000000000000 ) ) ;
#43966=CARTESIAN_POINT ( 'NONE',  ( 89.55818655986067256, 72.98405218941671535, 77.68655577178756744 ) ) ;
#43994=VERTEX_POINT ( 'NONE', #78220 ) ;
#44023=EDGE_CURVE ( 'NONE', #28006, #76633, #3242, .T. ) ;
#44027=EDGE_CURVE ( 'NONE', #23091, #87954, #64126, .T. ) ;
#44031=AXIS2_PLACEMENT_3D ( 'NONE', #69004, #22659, #56239 ) ;
#44065=CARTESIAN_POINT ( 'NONE',  ( 100.1374281256146901, 87.79544278253752054, -83.76986456925365587 ) ) ;
#44094=CARTESIAN_POINT ( 'NONE',  ( -96.70275196374414861, 93.55256755804781221, 87.71306776503882929 ) ) ;
#44100=ORIENTED_EDGE ( 'NONE', *, *, #61915, .F. ) ;
#44111=LINE ( 'NONE', #39092, #68891 ) ;
#44127=ORIENTED_EDGE ( 'NONE', *, *, #79574, .T. ) ;
#44131=ORIENTED_EDGE ( 'NONE', *, *, #9873, .T. ) ;
#44192=CARTESIAN_POINT ( 'NONE',  ( -74.15067561874319324, 127.0000000000000000, 68.53801554307369770 ) ) ;
#44202=AXIS2_PLACEMENT_3D ( 'NONE', #13909, #54310, #20288 ) ;
#44205=CARTESIAN_POINT ( 'NONE',  ( 118.0433965939932364, 76.18740257834568297, -11.02250383333830541 ) ) ;
#44225=ORIENTED_EDGE ( 'NONE', *, *, #84676, .F. ) ;
#44229=AXIS2_PLACEMENT_3D ( 'NONE', #70261, #36188, #64347 ) ;
#44230=ADVANCED_FACE ( 'NONE', ( #67690 ), #18193, .T. ) ;
#44265=CARTESIAN_POINT ( 'NONE',  ( -31.75000000000000000, 124.5870000000000033, 3.174999999999779998 ) ) ;
#44274=DIRECTION ( 'NONE',  ( -1.000000000000000000, 0.000000000000000000, -3.491483361109385222E-15 ) ) ;
#44308=AXIS2_PLACEMENT_3D ( 'NONE', #44421, #51234, #44878 ) ;
#44312=ORIENTED_EDGE ( 'NONE', *, *, #50039, .T. ) ;
#44332=ADVANCED_FACE ( 'NONE', ( #34046, #33615 ), #68592, .F. ) ;
#44348=AXIS2_PLACEMENT_3D ( 'NONE', #64447, #78548, #71279 ) ;
#44358=ORIENTED_EDGE ( 'NONE', *, *, #59308, .T. ) ;
#44366=DIRECTION ( 'NONE',  ( -0.000000000000000000, 1.000000000000000000, 0.000000000000000000 ) ) ;
#44369=CYLINDRICAL_SURFACE ( 'NONE', #51762, 7.937500000000000000 ) ;
#44385=DIRECTION ( 'NONE',  ( 0.000000000000000000, 1.000000000000000000, 0.000000000000000000 ) ) ;
#44386=DIRECTION ( 'NONE',  ( 0.000000000000000000, 0.000000000000000000, -1.000000000000000000 ) ) ;
#44394=CARTESIAN_POINT ( 'NONE',  ( 83.63178471058820662, 77.68489675156565966, 100.2530235599243440 ) ) ;
#44395=EDGE_CURVE ( 'NONE', #68997, #61226, #69935, .T. ) ;
#44402=CARTESIAN_POINT ( 'NONE',  ( 72.96458098368650269, 117.4749999999999943, 72.96458098368729850 ) ) ;
#44407=CARTESIAN_POINT ( 'NONE',  ( 91.81719692706791136, 78.06989712577869511, 75.00102098090833636 ) ) ;
#44421=CARTESIAN_POINT ( 'NONE',  ( 0.000000000000000000, 101.5999999999999943, 0.000000000000000000 ) ) ;
#44428=AXIS2_PLACEMENT_3D ( 'NONE', #88299, #81488, #87388 ) ;
#44431=B_SPLINE_CURVE_WITH_KNOTS ( 'NONE', 3,
 ( #22571, #31143, #79324, #24345, #45208, #72926, #77979, #66106, #18862, #12051, #54240, #24785, #73372, #45640, #87017, #46091, #67903, #19313, #88369, #67449, #17958, #31585, #82004, #46985, #39740 ),
 .UNSPECIFIED., .F., .F.,
 ( 4, 2, 2, 2, 2, 2, 2, 2, 2, 1, 2, 2, 4 ),
 ( 2.608264963112508895E-18, 0.002483666291998854608, 0.003725499437998279744, 0.004967332583997703145, 0.007450998875996568162, 0.008692832021995991129, 0.009934665167995411494, 0.01241833145999425222, 0.01366016460599367086, 0.01490199775199309122, 0.01614383089799251159, 0.01738566404399193022, 0.01986933033599076748 ),
 .UNSPECIFIED. ) ;
#44455=DIRECTION ( 'NONE',  ( -0.7071067811865414665, 0.000000000000000000, -0.7071067811865534569 ) ) ;
#44472=CARTESIAN_POINT ( 'NONE',  ( -7.937500000000730083, 120.6499999999999915, 103.1875000000000000 ) ) ;
#44483=FACE_OUTER_BOUND ( 'NONE', #88586, .T. ) ;
#44488=DIRECTION ( 'NONE',  ( 1.000000000000000000, 0.000000000000000000, 0.000000000000000000 ) ) ;
#44499=DIRECTION ( 'NONE',  ( 0.000000000000000000, 0.000000000000000000, 1.000000000000000000 ) ) ;
#44510=CARTESIAN_POINT ( 'NONE',  ( 4.163101094985349692E-14, 120.6499999999999915, -107.7702177616926065 ) ) ;
#44516=DIRECTION ( 'NONE',  ( 0.000000000000000000, -1.000000000000000000, 0.000000000000000000 ) ) ;
#44521=EDGE_CURVE ( 'NONE', #62133, #34136, #24027, .T. ) ;
#44525=VERTEX_POINT ( 'NONE', #84480 ) ;
#44531=ORIENTED_EDGE ( 'NONE', *, *, #57440, .T. ) ;
#44542=CARTESIAN_POINT ( 'NONE',  ( -100.7940789023221697, 84.21348395916260188, 82.97845804870382835 ) ) ;
#44552=EDGE_LOOP ( 'NONE', ( #71999, #7281, #85749, #79065, #70956, #954 ) ) ;
#44554=DIRECTION ( 'NONE',  ( 3.491483361109385222E-15, 0.000000000000000000, -1.000000000000000000 ) ) ;
#44555=DIRECTION ( 'NONE',  ( 0.000000000000000000, 0.000000000000000000, 1.000000000000000000 ) ) ;
#44557=AXIS2_PLACEMENT_3D ( 'NONE', #55586, #13841, #26132 ) ;
#44577=CARTESIAN_POINT ( 'NONE',  ( -72.96458098368751166, 127.0000000000000000, 80.10833098368618721 ) ) ;
#44590=CARTESIAN_POINT ( 'NONE',  ( -0.8398470015645936870, 69.84999999999999432, 130.5559999999999832 ) ) ;
#44597=CARTESIAN_POINT ( 'NONE',  ( -107.7702177616926065, 120.6499999999999915, -1.170464777364108012E-12 ) ) ;
#44623=DIRECTION ( 'NONE',  ( 0.000000000000000000, 0.000000000000000000, -1.000000000000000000 ) ) ;
#44629=CARTESIAN_POINT ( 'NONE',  ( 0.000000000000000000, 111.1250000000000000, 0.000000000000000000 ) ) ;
#44630=ORIENTED_EDGE ( 'NONE', *, *, #3745, .T. ) ;
#44634=ORIENTED_EDGE ( 'NONE', *, *, #51902, .F. ) ;
#44637=CARTESIAN_POINT ( 'NONE',  ( -100.8961411191535973, 120.6499999999999915, 3.968749999998880451 ) ) ;
#44642=EDGE_CURVE ( 'NONE', #36469, #27929, #32601, .T. ) ;
#44658=CARTESIAN_POINT ( 'NONE',  ( 118.4241986436612279, 71.14137858619481847, 5.641441481139795044 ) ) ;
#44689=ORIENTED_EDGE ( 'NONE', *, *, #87422, .T. ) ;
#44707=CARTESIAN_POINT ( 'NONE',  ( -130.0261942349058586, 77.68489670259145896, -11.75299076262979447 ) ) ;
#44711=AXIS2_PLACEMENT_3D ( 'NONE', #67154, #86276, #79477 ) ;
#44723=DIRECTION ( 'NONE',  ( -3.491483361109385222E-15, 0.000000000000000000, 1.000000000000000000 ) ) ;
#44740=ORIENTED_EDGE ( 'NONE', *, *, #3664, .F. ) ;
#44813=DIRECTION ( 'NONE',  ( 0.000000000000000000, 1.000000000000000000, 0.000000000000000000 ) ) ;
#44816=CARTESIAN_POINT ( 'NONE',  ( 0.000000000000000000, 127.0000000000000000, 0.000000000000000000 ) ) ;
#44818=AXIS2_PLACEMENT_3D ( 'NONE', #84870, #14476, #28524 ) ;
#44833=DIRECTION ( 'NONE',  ( 0.000000000000000000, 1.000000000000000000, 0.000000000000000000 ) ) ;
#44846=CARTESIAN_POINT ( 'NONE',  ( 0.4144590284063602859, 95.24999999999994316, -130.5559999999999832 ) ) ;
#44854=EDGE_CURVE ( 'NONE', #20813, #22549, #8393, .T. ) ;
#44865=CARTESIAN_POINT ( 'NONE',  ( 81.47036787067760599, 70.27763793881258891, 86.12934247706320434 ) ) ;
#44875=DIRECTION ( 'NONE',  ( 0.000000000000000000, 1.000000000000000000, 0.000000000000000000 ) ) ;
#44878=DIRECTION ( 'NONE',  ( 0.000000000000000000, 0.000000000000000000, -1.000000000000000000 ) ) ;
#44881=CARTESIAN_POINT ( 'NONE',  ( -3.968750000000770051, 127.0000000000000000, 105.4788588808462038 ) ) ;
#44899=FACE_OUTER_BOUND ( 'NONE', #84380, .T. ) ;
#44903=VECTOR ( 'NONE', #79219, 1000.000000000000000 ) ;
#44913=CIRCLE ( 'NONE', #7205, 5.041900000000001825 ) ;
#44948=DIRECTION ( 'NONE',  ( 0.000000000000000000, -1.000000000000000000, 0.000000000000000000 ) ) ;
#44956=DIRECTION ( 'NONE',  ( 0.000000000000000000, 1.000000000000000000, 0.000000000000000000 ) ) ;
#44977=AXIS2_PLACEMENT_3D ( 'NONE', #84918, #17204, #2684 ) ;
#44985=ORIENTED_EDGE ( 'NONE', *, *, #10468, .T. ) ;
#44986=ORIENTED_EDGE ( 'NONE', *, *, #25552, .T. ) ;
#45005=CYLINDRICAL_SURFACE ( 'NONE', #33142, 34.13125000000000142 ) ;
#45008=DIRECTION ( 'NONE',  ( -0.8660254037844387076, 0.000000000000000000, 0.4999999999999998890 ) ) ;
#45031=VERTEX_POINT ( 'NONE', #30169 ) ;
#45038=CARTESIAN_POINT ( 'NONE',  ( -12.37530111100094743, 79.66613297688917328, 129.9681797613511947 ) ) ;
#45049=ORIENTED_EDGE ( 'NONE', *, *, #40096, .T. ) ;
#45100=CARTESIAN_POINT ( 'NONE',  ( 117.9190617242381194, 79.25941250729452747, 12.27333445685097502 ) ) ;
#45103=CARTESIAN_POINT ( 'NONE',  ( 3.174999999999879918, 104.3431970271541900, 33.98325472291465132 ) ) ;
#45132=EDGE_CURVE ( 'NONE', #4380, #16856, #10286, .T. ) ;
#45139=AXIS2_PLACEMENT_3D ( 'NONE', #8237, #21874, #62289 ) ;
#45150=VECTOR ( 'NONE', #4387, 1000.000000000000000 ) ;
#45192=DIRECTION ( 'NONE',  ( 0.000000000000000000, 0.000000000000000000, -1.000000000000000000 ) ) ;
#45202=ORIENTED_EDGE ( 'NONE', *, *, #65396, .T. ) ;
#45208=CARTESIAN_POINT ( 'NONE',  ( 3.286472755014015146, 70.27551020174914242, -130.5152393712291428 ) ) ;
#45215=CARTESIAN_POINT ( 'NONE',  ( 12.27464498081148214, 85.83590841536246785, 129.9777558447946149 ) ) ;
#45223=ORIENTED_EDGE ( 'NONE', *, *, #82554, .F. ) ;
#45228=DIRECTION ( 'NONE',  ( 0.000000000000000000, -1.000000000000000000, 0.000000000000000000 ) ) ;
#45239=ADVANCED_FACE ( 'NONE', ( #28254 ), #75974, .F. ) ;
#45242=EDGE_CURVE ( 'NONE', #84780, #23774, #63240, .T. ) ;
#45256=ORIENTED_EDGE ( 'NONE', *, *, #57810, .F. ) ;
#45261=EDGE_CURVE ( 'NONE', #64426, #69399, #30652, .T. ) ;
#45267=ADVANCED_FACE ( 'NONE', ( #1954, #29647 ), #65510, .T. ) ;
#45272=DIRECTION ( 'NONE',  ( -0.000000000000000000, 1.000000000000000000, 0.000000000000000000 ) ) ;
#45273=LINE ( 'NONE', #2631, #80041 ) ;
#45275=CARTESIAN_POINT ( 'NONE',  ( 0.000000000000000000, 103.1240000000000236, -190.5000000000000000 ) ) ;
#45297=DIRECTION ( 'NONE',  ( -0.9659258262890675351, 0.000000000000000000, -0.2588190451025234595 ) ) ;
#45299=AXIS2_PLACEMENT_3D ( 'NONE', #41533, #56054, #63799 ) ;
#45302=CARTESIAN_POINT ( 'NONE',  ( 90.31351860656735653, 74.16967745525860778, 76.80536679343944684 ) ) ;
#45314=CARTESIAN_POINT ( 'NONE',  ( 117.8738102209306362, 82.96450994655477018, 12.70000000000123208 ) ) ;
#45338=EDGE_CURVE ( 'NONE', #6564, #59781, #37359, .T. ) ;
#45345=CARTESIAN_POINT ( 'NONE',  ( -117.9083666784912481, 79.66685870724431595, 12.37533002638040180 ) ) ;
#45351=EDGE_CURVE ( 'NONE', #48000, #41588, #23314, .T. ) ;
#45368=DIRECTION ( 'NONE',  ( 0.000000000000000000, 0.000000000000000000, -1.000000000000000000 ) ) ;
#45374=FACE_BOUND ( 'NONE', #25688, .T. ) ;
#45383=FACE_OUTER_BOUND ( 'NONE', #87092, .T. ) ;
#45407=DIRECTION ( 'NONE',  ( -0.000000000000000000, 1.000000000000000000, -0.000000000000000000 ) ) ;
#45418=ORIENTED_EDGE ( 'NONE', *, *, #65102, .F. ) ;
#45421=ORIENTED_EDGE ( 'NONE', *, *, #34811, .F. ) ;
#45427=CARTESIAN_POINT ( 'NONE',  ( -100.5986936721440230, 85.85000629251467785, 83.21537498884013928 ) ) ;
#45451=ORIENTED_EDGE ( 'NONE', *, *, #41674, .T. ) ;
#45460=ORIENTED_EDGE ( 'NONE', *, *, #8266, .T. ) ;
#45461=EDGE_CURVE ( 'NONE', #30848, #78871, #12338, .T. ) ;
#45470=FACE_OUTER_BOUND ( 'NONE', #71791, .T. ) ;
#45478=CARTESIAN_POINT ( 'NONE',  ( 4.163101094985349692E-14, 120.6499999999999915, -98.60478223830740774 ) ) ;
#45514=CYLINDRICAL_SURFACE ( 'NONE', #83804, 7.143750000000004263 ) ;
#45526=ADVANCED_FACE ( 'NONE', ( #67750 ), #87302, .F. ) ;
#45532=CARTESIAN_POINT ( 'NONE',  ( 118.0639734269499854, 75.84278307195158675, 10.79247489890550682 ) ) ;
#45538=EDGE_LOOP ( 'NONE', ( #25693, #24275, #53505, #3934 ) ) ;
#45539=LINE ( 'NONE', #11504, #22731 ) ;
#45552=CARTESIAN_POINT ( 'NONE',  ( -8.690994986491583418, 73.28026231907210786, 118.2373793989773247 ) ) ;
#45554=ADVANCED_FACE ( 'NONE', ( #26419 ), #13678, .F. ) ;
#45560=DIRECTION ( 'NONE',  ( 0.000000000000000000, -1.000000000000000000, 0.000000000000000000 ) ) ;
#45568=ORIENTED_EDGE ( 'NONE', *, *, #44027, .T. ) ;
#45582=ORIENTED_EDGE ( 'NONE', *, *, #49597, .F. ) ;
#45583=DIRECTION ( 'NONE',  ( 0.000000000000000000, 0.000000000000000000, 1.000000000000000000 ) ) ;
#45601=ORIENTED_EDGE ( 'NONE', *, *, #48104, .F. ) ;
#45617=ORIENTED_EDGE ( 'NONE', *, *, #69947, .T. ) ;
#45620=CARTESIAN_POINT ( 'NONE',  ( -5.616699032889719945, 93.94804372660796332, -130.4356411629705121 ) ) ;
#45640=CARTESIAN_POINT ( 'NONE',  ( 9.569027000640168978, 74.15895453169299856, -130.2061718688152610 ) ) ;
#45644=CARTESIAN_POINT ( 'NONE',  ( 74.49778344313774880, 84.62843115047674303, 92.22587532767886387 ) ) ;
#45649=ADVANCED_FACE ( 'NONE', ( #5537 ), #69099, .F. ) ;
#45650=CARTESIAN_POINT ( 'NONE',  ( 12.70000000000000107, 82.54999999999999716, 129.9368274816650910 ) ) ;
#45666=DIRECTION ( 'NONE',  ( 0.000000000000000000, 0.000000000000000000, 1.000000000000000000 ) ) ;
#45690=ORIENTED_EDGE ( 'NONE', *, *, #56377, .F. ) ;
#45703=DIRECTION ( 'NONE',  ( 0.7071067811865398012, 0.000000000000000000, 0.7071067811865552333 ) ) ;
#45719=CARTESIAN_POINT ( 'NONE',  ( 12.59759614370980785, 84.21308071816548591, -129.9468022370901679 ) ) ;
#45723=ORIENTED_EDGE ( 'NONE', *, *, #24921, .T. ) ;
#45738=AXIS2_PLACEMENT_3D ( 'NONE', #37568, #58876, #39341 ) ;
#45747=CARTESIAN_POINT ( 'NONE',  ( 118.5129862669514296, 94.84303900880917126, 3.295572367533603497 ) ) ;
#45756=LINE ( 'NONE', #24015, #69903 ) ;
#45787=CARTESIAN_POINT ( 'NONE',  ( -118.5559323284755067, 69.85063172184842983, -0.8489616598194429375 ) ) ;
#45789=VECTOR ( 'NONE', #56807, 1000.000000000000114 ) ;
#45800=ORIENTED_EDGE ( 'NONE', *, *, #52461, .F. ) ;
#45849=ADVANCED_FACE ( 'NONE', ( #22300 ), #4586, .T. ) ;
#45868=CARTESIAN_POINT ( 'NONE',  ( -118.1705221151483443, 90.93965867633437483, -9.571124722858089129 ) ) ;
#45878=ORIENTED_EDGE ( 'NONE', *, *, #69796, .F. ) ;
#45897=ORIENTED_EDGE ( 'NONE', *, *, #15554, .T. ) ;
#45913=ORIENTED_EDGE ( 'NONE', *, *, #80119, .F. ) ;
#45919=EDGE_LOOP ( 'NONE', ( #24835, #20743, #57000, #64484 ) ) ;
#45921=ORIENTED_EDGE ( 'NONE', *, *, #70243, .F. ) ;
#45928=ADVANCED_FACE ( 'NONE', ( #59021 ), #31777, .F. ) ;
#45930=VERTEX_POINT ( 'NONE', #24969 ) ;
#45933=SURFACE_STYLE_USAGE ( .BOTH. , #5542 ) ;
#45935=LINE ( 'NONE', #46836, #59313 ) ;
#45970=CARTESIAN_POINT ( 'NONE',  ( -85.52748787272784625, 73.86195533656251655, 98.64078293412708831 ) ) ;
#45996=VECTOR ( 'NONE', #57588, 1000.000000000000000 ) ;
#46021=DIRECTION ( 'NONE',  ( 0.000000000000000000, 0.000000000000000000, 1.000000000000000000 ) ) ;
#46027=DIRECTION ( 'NONE',  ( 0.8660254037844381525, 0.000000000000000000, 0.5000000000000007772 ) ) ;
#46037=ORIENTED_EDGE ( 'NONE', *, *, #9680, .F. ) ;
#46091=CARTESIAN_POINT ( 'NONE',  ( 10.79079172156231081, 75.84006377869074811, -130.1095006741098530 ) ) ;
#46101=CARTESIAN_POINT ( 'NONE',  ( 11.02183147610883829, 88.91382474694671600, 130.0907465706570179 ) ) ;
#46136=CYLINDRICAL_SURFACE ( 'NONE', #29135, 5.041900000000001825 ) ;
#46138=CARTESIAN_POINT ( 'NONE',  ( 130.0134586223094288, 78.07027470200929997, -11.89097723361176762 ) ) ;
#46139=EDGE_LOOP ( 'NONE', ( #34730, #87603, #46037, #88757 ) ) ;
#46148=ORIENTED_EDGE ( 'NONE', *, *, #62505, .T. ) ;
#46155=CARTESIAN_POINT ( 'NONE',  ( -72.96458098368600531, 101.5999999999999943, -67.92268098368781182 ) ) ;
#46158=DIRECTION ( 'NONE',  ( 0.000000000000000000, 0.000000000000000000, 1.000000000000000000 ) ) ;
#46173=CARTESIAN_POINT ( 'NONE',  ( 12.29205751230852073, 85.84923025428284404, -129.9761558897303644 ) ) ;
#46179=VECTOR ( 'NONE', #4501, 1000.000000000000000 ) ;
#46187=CARTESIAN_POINT ( 'NONE',  ( 100.8961411191535973, 127.0000000000000000, 3.968750000000400124 ) ) ;
#46195=DIRECTION ( 'NONE',  ( -0.000000000000000000, 1.000000000000000000, 0.000000000000000000 ) ) ;
#46198=CARTESIAN_POINT ( 'NONE',  ( 118.3860192952350161, 93.55239623846827612, 6.356965277240638201 ) ) ;
#46206=CARTESIAN_POINT ( 'NONE',  ( -103.1875000000000000, 127.0000000000000000, -5.041900000001080073 ) ) ;
#46233=CARTESIAN_POINT ( 'NONE',  ( -118.0433965939931653, 76.18740257834569718, 11.02250383333912787 ) ) ;
#46238=ORIENTED_EDGE ( 'NONE', *, *, #77372, .T. ) ;
#46291=DIRECTION ( 'NONE',  ( 0.000000000000000000, -1.000000000000000000, 0.000000000000000000 ) ) ;
#46294=CARTESIAN_POINT ( 'NONE',  ( -69.72411017812909506, 120.6499999999999915, -69.72411017813089984 ) ) ;
#46320=CARTESIAN_POINT ( 'NONE',  ( -85.31607583734405864, 90.93081950567957961, 98.82361644294769576 ) ) ;
#46324=CIRCLE ( 'NONE', #4347, 7.143750000000004263 ) ;
#46334=DIRECTION ( 'NONE',  ( -0.9659258262890706437, 0.000000000000000000, 0.2588190451025119132 ) ) ;
#46364=CARTESIAN_POINT ( 'NONE',  ( 68.53801554307389665, 120.6499999999999915, 74.15067561874289481 ) ) ;
#46375=EDGE_CURVE ( 'NONE', #64021, #3056, #30350, .T. ) ;
#46390=DIRECTION ( 'NONE',  ( 0.000000000000000000, 1.000000000000000000, 0.000000000000000000 ) ) ;
#46391=DIRECTION ( 'NONE',  ( -1.000000000000000000, 0.000000000000000000, 3.596091637922019804E-15 ) ) ;
#46395=DIRECTION ( 'NONE',  ( -0.2588190451025170757, 0.000000000000000000, 0.9659258262890693114 ) ) ;
#46398=AXIS2_PLACEMENT_3D ( 'NONE', #60598, #47860, #75598 ) ;
#46408=DIRECTION ( 'NONE',  ( 0.000000000000000000, 0.000000000000000000, 1.000000000000000000 ) ) ;
#46411=VECTOR ( 'NONE', #28730, 1000.000000000000000 ) ;
#46441=ORIENTED_EDGE ( 'NONE', *, *, #78833, .T. ) ;
#46443=CARTESIAN_POINT ( 'NONE',  ( -95.69968022530730423, 70.80031561532538831, -88.80809839403329420 ) ) ;
#46501=DIRECTION ( 'NONE',  ( 0.000000000000000000, 1.000000000000000000, 0.000000000000000000 ) ) ;
#46507=CARTESIAN_POINT ( 'NONE',  ( -6.710838307577465578, 93.34022857041043153, -118.3664257206621784 ) ) ;
#46515=VECTOR ( 'NONE', #84261, 1000.000000000000114 ) ;
#46534=CARTESIAN_POINT ( 'NONE',  ( -75.00102098090737002, 78.06989712577870932, 91.81719692706870717 ) ) ;
#46545=DIRECTION ( 'NONE',  ( 0.000000000000000000, 1.000000000000000000, 0.000000000000000000 ) ) ;
#46557=CARTESIAN_POINT ( 'NONE',  ( -88.53717826876616925, 94.12569442554142540, -95.94886839522614252 ) ) ;
#46572=DIRECTION ( 'NONE',  ( 0.000000000000000000, 1.000000000000000000, 0.000000000000000000 ) ) ;
#46578=VERTEX_POINT ( 'NONE', #25751 ) ;
#46599=CYLINDRICAL_SURFACE ( 'NONE', #12749, 12.70000000000000107 ) ;
#46603=CARTESIAN_POINT ( 'NONE',  ( -72.96458098368600531, 127.0000000000000000, -80.10833098368780725 ) ) ;
#46631=EDGE_LOOP ( 'NONE', ( #87401, #57101, #60306, #12829, #35742, #54084 ) ) ;
#46659=VECTOR ( 'NONE', #2455, 1000.000000000000000 ) ;
#46687=EDGE_LOOP ( 'NONE', ( #52347, #6842, #29320, #70499 ) ) ;
#46688=CARTESIAN_POINT ( 'NONE',  ( -118.4576332894986166, 70.80054595721396993, 4.873637472995685727 ) ) ;
#46712=DIRECTION ( 'NONE',  ( 1.000000000000000000, 0.000000000000000000, 1.047445008332813989E-14 ) ) ;
#46726=ORIENTED_EDGE ( 'NONE', *, *, #17189, .T. ) ;
#46727=AXIS2_PLACEMENT_3D ( 'NONE', #17541, #79783, #57967 ) ;
#46732=CARTESIAN_POINT ( 'NONE',  ( -129.9468070739258110, 84.21348395916261609, -12.59754631664223723 ) ) ;
#46740=AXIS2_PLACEMENT_3D ( 'NONE', #36140, #1178, #84315 ) ;
#46743=CARTESIAN_POINT ( 'NONE',  ( 99.62873342662678056, 89.26666702275855414, -84.37439091330300300 ) ) ;
#46747=CARTESIAN_POINT ( 'NONE',  ( -12.70000000000000107, 82.54999999999999716, -117.8738102209307641 ) ) ;
#46760=EDGE_LOOP ( 'NONE', ( #54955, #19950, #14158, #48686 ) ) ;
#46761=CARTESIAN_POINT ( 'NONE',  ( -71.77848634863190114, 120.6499999999999915, 77.39114642429879609 ) ) ;
#46768=CARTESIAN_POINT ( 'NONE',  ( -84.91247172076023730, 90.28418055714726620, 99.17062120112684909 ) ) ;
#46777=EDGE_LOOP ( 'NONE', ( #75054, #62308 ) ) ;
#46787=CARTESIAN_POINT ( 'NONE',  ( 89.13001032377211175, 92.64969027323468254, -78.17826422383492968 ) ) ;
#46799=EDGE_CURVE ( 'NONE', #79245, #87954, #28439, .T. ) ;
#46804=CARTESIAN_POINT ( 'NONE',  ( 130.5560151749589295, 95.25015599858943460, 0.4097429349709048596 ) ) ;
#46817=EDGE_CURVE ( 'NONE', #7174, #64426, #8921, .T. ) ;
#46818=VERTEX_POINT ( 'NONE', #62957 ) ;
#46835=PRESENTATION_STYLE_ASSIGNMENT (( #45933 ) ) ;
#46836=CARTESIAN_POINT ( 'NONE',  ( -7.205548786489490269E-13, 127.0000000000000000, 108.2293999999999983 ) ) ;
#46837=CARTESIAN_POINT ( 'NONE',  ( -72.96458098368600531, 117.4749999999999943, -67.92268098368781182 ) ) ;
#46863=FACE_BOUND ( 'NONE', #84169, .T. ) ;
#46874=ADVANCED_FACE ( 'NONE', ( #28906 ), #2090, .F. ) ;
#46885=ADVANCED_FACE ( 'NONE', ( #55665 ), #77954, .F. ) ;
#46913=VERTEX_POINT ( 'NONE', #31561 ) ;
#46915=LINE ( 'NONE', #18332, #19812 ) ;
#46951=CARTESIAN_POINT ( 'NONE',  ( -7.752335291937824557, 92.64399975678504973, -118.3043120271755413 ) ) ;
#46952=EDGE_LOOP ( 'NONE', ( #5910, #45451, #56230, #42168 ) ) ;
#46959=CARTESIAN_POINT ( 'NONE',  ( 76.20505178924339873, 120.6499999999999915, 76.20505178924419454 ) ) ;
#46966=CARTESIAN_POINT ( 'NONE',  ( 68.53801554307449351, 120.6499999999999915, -74.15067561874229796 ) ) ;
#46985=CARTESIAN_POINT ( 'NONE',  ( 12.70000000000000462, 81.72090770373000623, -129.9368274816651194 ) ) ;
#46996=CARTESIAN_POINT ( 'NONE',  ( -83.02643542998004023, 84.62817240485476589, -100.7545871043107581 ) ) ;
#47021=ORIENTED_EDGE ( 'NONE', *, *, #49953, .F. ) ;
#47028=CARTESIAN_POINT ( 'NONE',  ( 68.91674821478362389, 82.54999999999999716, 68.91674821478530077 ) ) ;
#47042=LINE ( 'NONE', #12555, #10188 ) ;
#47055=DIRECTION ( 'NONE',  ( 0.000000000000000000, 1.000000000000000000, 0.000000000000000000 ) ) ;
#47075=AXIS2_PLACEMENT_3D ( 'NONE', #41036, #62376, #67394 ) ;
#47083=CARTESIAN_POINT ( 'NONE',  ( 33.98325472291465132, 104.3431970271542042, 3.174999999999999822 ) ) ;
#47093=CARTESIAN_POINT ( 'NONE',  ( -7.205548786489490269E-13, 127.0000000000000000, 103.1875000000000000 ) ) ;
#47098=EDGE_CURVE ( 'NONE', #68997, #37445, #74156, .T. ) ;
#47099=CARTESIAN_POINT ( 'NONE',  ( 118.3862315815644450, 93.55466788070661721, -6.352948492896714150 ) ) ;
#47173=VERTEX_POINT ( 'NONE', #44577 ) ;
#47175=CARTESIAN_POINT ( 'NONE',  ( -130.1098569802758504, 89.26666702275855414, -10.78644903371280961 ) ) ;
#47186=CARTESIAN_POINT ( 'NONE',  ( 93.77212533081413426, 95.08644067748868167, -90.83954799657421120 ) ) ;
#47190=CARTESIAN_POINT ( 'NONE',  ( -2.899925867002088431, 70.17843955035350234, -118.5212385615275252 ) ) ;
#47213=LINE ( 'NONE', #89020, #53003 ) ;
#47220=CARTESIAN_POINT ( 'NONE',  ( -118.1262036371152533, 90.29828471680515634, -10.09645181158828287 ) ) ;
#47221=CIRCLE ( 'NONE', #16781, 5.041900000000001825 ) ;
#47222=DIRECTION ( 'NONE',  ( -0.8660254037844351549, 0.000000000000000000, -0.5000000000000061062 ) ) ;
#47228=ORIENTED_EDGE ( 'NONE', *, *, #25695, .T. ) ;
#47250=DIRECTION ( 'NONE',  ( 0.7071067811865389130, 0.000000000000000000, 0.7071067811865561215 ) ) ;
#47256=CARTESIAN_POINT ( 'NONE',  ( 129.9989688714891827, 86.64186789594792515, 12.05153810119577251 ) ) ;
#47265=EDGE_LOOP ( 'NONE', ( #65006, #44100, #71617, #30282 ) ) ;
#47277=CARTESIAN_POINT ( 'NONE',  ( -91.51265874544272094, 76.91656954603719498, -75.37281393334477286 ) ) ;
#47297=DIRECTION ( 'NONE',  ( 0.000000000000000000, 1.000000000000000000, 0.000000000000000000 ) ) ;
#47317=DIRECTION ( 'NONE',  ( 0.000000000000000000, 0.000000000000000000, 1.000000000000000000 ) ) ;
#47321=ORIENTED_EDGE ( 'NONE', *, *, #70178, .T. ) ;
#47330=AXIS2_PLACEMENT_3D ( 'NONE', #66333, #79998, #85924 ) ;
#47342=CARTESIAN_POINT ( 'NONE',  ( -99.17101862044600580, 74.81660785136578795, -84.91200770515642660 ) ) ;
#47360=DIRECTION ( 'NONE',  ( 0.000000000000000000, 1.000000000000000000, 0.000000000000000000 ) ) ;
#47368=ADVANCED_FACE ( 'NONE', ( #32176 ), #59872, .F. ) ;
#47392=DIRECTION ( 'NONE',  ( 1.000000000000000000, 0.000000000000000000, 0.000000000000000000 ) ) ;
#47415=EDGE_CURVE ( 'NONE', #60807, #72752, #27608, .T. ) ;
#47442=CARTESIAN_POINT ( 'NONE',  ( 91.81710919847640184, 87.03046781249440755, 75.00112839233788975 ) ) ;
#47454=DIRECTION ( 'NONE',  ( -0.7071067811865410224, 0.000000000000000000, -0.7071067811865540120 ) ) ;
#47462=ORIENTED_EDGE ( 'NONE', *, *, #50284, .F. ) ;
#47476=PLANE ( 'NONE',  #34777 ) ;
#47489=ORIENTED_EDGE ( 'NONE', *, *, #42854, .T. ) ;
#47495=DIRECTION ( 'NONE',  ( -0.8660254037844390407, 0.000000000000000000, -0.4999999999999995004 ) ) ;
#47508=ADVANCED_FACE ( 'NONE', ( #13536 ), #41662, .F. ) ;
#47521=PLANE ( 'NONE',  #38753 ) ;
#47550=CARTESIAN_POINT ( 'NONE',  ( 0.000000000000000000, 92.07499999999998863, 88.90000000000000568 ) ) ;
#47610=DIRECTION ( 'NONE',  ( 0.000000000000000000, -1.000000000000000000, 0.000000000000000000 ) ) ;
#47627=CARTESIAN_POINT ( 'NONE',  ( -129.9989688714893248, 86.64186789594789673, -12.05153810119486124 ) ) ;
#47639=CARTESIAN_POINT ( 'NONE',  ( 89.95770503246907879, 94.82199753261677699, -94.61838531165687982 ) ) ;
#47666=EDGE_LOOP ( 'NONE', ( #71325, #77194 ) ) ;
#47670=CARTESIAN_POINT ( 'NONE',  ( -118.0058645681207281, 88.18374315479978520, 11.41243735079867250 ) ) ;
#47696=PLANE ( 'NONE',  #41948 ) ;
#47704=CARTESIAN_POINT ( 'NONE',  ( 130.2060295542615904, 90.93932679091003024, 9.571439627455211152 ) ) ;
#47726=CARTESIAN_POINT ( 'NONE',  ( -86.13269706310892104, 70.27900073646854651, -81.46681417397479663 ) ) ;
#47734=DIRECTION ( 'NONE',  ( -0.7071067811865410224, 0.000000000000000000, -0.7071067811865540120 ) ) ;
#47748=CARTESIAN_POINT ( 'NONE',  ( 12.61759658107631665, 80.88542946572127335, 117.8827710199055048 ) ) ;
#47770=ORIENTED_EDGE ( 'NONE', *, *, #74708, .F. ) ;
#47789=CARTESIAN_POINT ( 'NONE',  ( -100.5877059554739361, 79.26455342200334542, -83.22858459372935158 ) ) ;
#47799=EDGE_LOOP ( 'NONE', ( #38680, #69381 ) ) ;
#47813=CARTESIAN_POINT ( 'NONE',  ( 9.270368442002547837, 91.24032474172571483, 118.1933656790130129 ) ) ;
#47824=CARTESIAN_POINT ( 'NONE',  ( 71.77848634863140376, 120.6499999999999915, -77.39114642429929347 ) ) ;
#47845=CARTESIAN_POINT ( 'NONE',  ( 4.090931056105404195, 94.60184303864159006, -118.4878965444427621 ) ) ;
#47854=LINE ( 'NONE', #13361, #13302 ) ;
#47860=DIRECTION ( 'NONE',  ( 0.000000000000000000, 1.000000000000000000, 0.000000000000000000 ) ) ;
#47874=DIRECTION ( 'NONE',  ( 0.000000000000000000, -1.000000000000000000, 0.000000000000000000 ) ) ;
#47875=CARTESIAN_POINT ( 'NONE',  ( -90.66736180499643183, 74.80137413886471620, 76.38829385798661065 ) ) ;
#47880=VERTEX_POINT ( 'NONE', #86676 ) ;
#47896=CARTESIAN_POINT ( 'NONE',  ( -95.69832483115250454, 94.30053025434479252, -88.80956239834407029 ) ) ;
#47913=ORIENTED_EDGE ( 'NONE', *, *, #89114, .T. ) ;
#47916=ORIENTED_EDGE ( 'NONE', *, *, #40683, .F. ) ;
#47950=LINE ( 'NONE', #14817, #81775 ) ;
#47961=ORIENTED_EDGE ( 'NONE', *, *, #2124, .F. ) ;
#47994=VECTOR ( 'NONE', #73291, 1000.000000000000000 ) ;
#47995=DIRECTION ( 'NONE',  ( -0.9659258262890690894, 0.000000000000000000, -0.2588190451025180749 ) ) ;
#47999=DIRECTION ( 'NONE',  ( 0.000000000000000000, -1.000000000000000000, 0.000000000000000000 ) ) ;
#48000=VERTEX_POINT ( 'NONE', #53901 ) ;
#48013=ORIENTED_EDGE ( 'NONE', *, *, #26762, .T. ) ;
#48079=EDGE_LOOP ( 'NONE', ( #64118, #62584 ) ) ;
#48083=CARTESIAN_POINT ( 'NONE',  ( 92.89936586972048360, 95.23006786499112764, -91.73195104381109388 ) ) ;
#48104=EDGE_CURVE ( 'NONE', #80081, #89588, #34376, .T. ) ;
#48108=CARTESIAN_POINT ( 'NONE',  ( -76.20505178924449297, 120.6499999999999915, 76.20505178924310030 ) ) ;
#48112=CARTESIAN_POINT ( 'NONE',  ( 89.75424775947713840, 73.28361289573331305, -77.45828646618613789 ) ) ;
#48119=ORIENTED_EDGE ( 'NONE', *, *, #39616, .F. ) ;
#48132=ORIENTED_EDGE ( 'NONE', *, *, #28055, .T. ) ;
#48139=ORIENTED_EDGE ( 'NONE', *, *, #58609, .F. ) ;
#48151=CARTESIAN_POINT ( 'NONE',  ( 129.9777364973648162, 85.83513192049079521, -12.27484926614918237 ) ) ;
#48156=AXIS2_PLACEMENT_3D ( 'NONE', #44816, #44366, #2611 ) ;
#48161=CARTESIAN_POINT ( 'NONE',  ( -3.306647731859349904, 70.28099577563533273, -130.5147235605103617 ) ) ;
#48162=DIRECTION ( 'NONE',  ( 0.000000000000000000, 1.000000000000000000, 0.000000000000000000 ) ) ;
#48188=PLANE ( 'NONE',  #2564 ) ;
#48190=CARTESIAN_POINT ( 'NONE',  ( 11.02404012120765842, 76.19011824550719325, 118.0432514857309911 ) ) ;
#48207=FACE_BOUND ( 'NONE', #28358, .T. ) ;
#48211=CARTESIAN_POINT ( 'NONE',  ( -89.95524642164049567, 70.27892663483464730, 94.62072105690099022 ) ) ;
#48245=DIRECTION ( 'NONE',  ( -0.7071067811865437980, 0.000000000000000000, -0.7071067811865512365 ) ) ;
#48256=CARTESIAN_POINT ( 'NONE',  ( -33.98325472291465132, 111.1250000000000000, 3.174999999999764899 ) ) ;
#48283=CARTESIAN_POINT ( 'NONE',  ( 92.32962665258612844, 82.54999999999999716, -74.36911441044637172 ) ) ;
#48286=CARTESIAN_POINT ( 'NONE',  ( 0.000000000000000000, 125.4759999999999991, -190.5000000000000000 ) ) ;
#48290=EDGE_LOOP ( 'NONE', ( #64768, #36636, #20356, #54614 ) ) ;
#48303=CARTESIAN_POINT ( 'NONE',  ( 31.75000000000000000, 104.3431970271542042, 3.174999999999999822 ) ) ;
#48313=CARTESIAN_POINT ( 'NONE',  ( -76.80536679343852313, 74.16967745525863620, 90.31351860656819497 ) ) ;
#48337=CARTESIAN_POINT ( 'NONE',  ( -96.20559720633563927, 93.94653598907719072, -88.25806911646377273 ) ) ;
#48338=PLANE ( 'NONE',  #70029 ) ;
#48349=EDGE_LOOP ( 'NONE', ( #52914, #86159 ) ) ;
#48363=ORIENTED_EDGE ( 'NONE', *, *, #83984, .T. ) ;
#48377=DIRECTION ( 'NONE',  ( -0.000000000000000000, 1.000000000000000000, 0.000000000000000000 ) ) ;
#48405=CARTESIAN_POINT ( 'NONE',  ( -72.96458098368751166, 127.0000000000000000, 72.96458098368620426 ) ) ;
#48443=CARTESIAN_POINT ( 'NONE',  ( -103.1875000000000000, 127.0000000000000000, -1.080832317973422076E-12 ) ) ;
#48449=ORIENTED_EDGE ( 'NONE', *, *, #41293, .F. ) ;
#48455=CARTESIAN_POINT ( 'NONE',  ( -6.359675246477835664, 93.55082578214793898, 118.3858732848555775 ) ) ;
#48461=CARTESIAN_POINT ( 'NONE',  ( -118.3250318368775567, 72.22378176823141871, -7.404816947594603960 ) ) ;
#48474=PRODUCT_DEFINITION_SHAPE ( 'NONE', 'NONE',  #61649 ) ;
#48483=CARTESIAN_POINT ( 'NONE',  ( 72.96458098368701428, 101.5999999999999943, -72.96458098368670164 ) ) ;
#48496=AXIS2_PLACEMENT_3D ( 'NONE', #17898, #73305, #57446 ) ;
#48503=DIRECTION ( 'NONE',  ( -0.000000000000000000, 1.000000000000000000, 0.000000000000000000 ) ) ;
#48553=CARTESIAN_POINT ( 'NONE',  ( 75.67519899969724406, 76.18740257834571139, -91.26337341211403498 ) ) ;
#48575=CARTESIAN_POINT ( 'NONE',  ( 82.65294504194743297, 95.16897323824362331, -84.99816483510849707 ) ) ;
#48592=EDGE_LOOP ( 'NONE', ( #42229, #6221 ) ) ;
#48594=DIRECTION ( 'NONE',  ( 0.7071067811865560104, 0.000000000000000000, -0.7071067811865391350 ) ) ;
#48595=EDGE_LOOP ( 'NONE', ( #75965, #3118, #71196, #54330 ) ) ;
#48602=CARTESIAN_POINT ( 'NONE',  ( -11.02410282832817856, 76.19023921641802133, -130.0905510769329965 ) ) ;
#48609=CARTESIAN_POINT ( 'NONE',  ( -83.23139715273258332, 69.85063172184842983, -84.43201024598432980 ) ) ;
#48613=CARTESIAN_POINT ( 'NONE',  ( -72.96458098368751166, 117.4749999999999943, 78.00648098368618832 ) ) ;
#48616=DIRECTION ( 'NONE',  ( -0.000000000000000000, -0.000000000000000000, 1.000000000000000000 ) ) ;
#48625=CARTESIAN_POINT ( 'NONE',  ( 83.41556370846545576, 78.46683822716995849, -100.4327019155581979 ) ) ;
#48628=DIRECTION ( 'NONE',  ( 0.000000000000000000, -1.000000000000000000, 0.000000000000000000 ) ) ;
#48635=CARTESIAN_POINT ( 'NONE',  ( 12.27510648567648133, 79.26588701359587219, 117.9188774285743762 ) ) ;
#48640=CARTESIAN_POINT ( 'NONE',  ( -76.20505178924278766, 120.6499999999999915, -76.20505178924469192 ) ) ;
#48642=PLANE ( 'NONE',  #45139 ) ;
#48644=EDGE_CURVE ( 'NONE', #31262, #88514, #21557, .T. ) ;
#48660=DIRECTION ( 'NONE',  ( -0.9659258262890686453, 0.000000000000000000, 0.2588190451025194072 ) ) ;
#48667=CARTESIAN_POINT ( 'NONE',  ( -7.205548786489490269E-13, 127.0000000000000000, 103.1875000000000000 ) ) ;
#48680=CARTESIAN_POINT ( 'NONE',  ( -92.27768215249976436, 84.21498941703525531, -74.43373480440716605 ) ) ;
#48686=ORIENTED_EDGE ( 'NONE', *, *, #10710, .F. ) ;
#48703=EDGE_LOOP ( 'NONE', ( #34199, #80363, #8635, #77193 ) ) ;
#48705=CARTESIAN_POINT ( 'NONE',  ( 10.33011338239549737, 89.94938708489701185, 118.1053235025621433 ) ) ;
#48707=ORIENTED_EDGE ( 'NONE', *, *, #38806, .T. ) ;
#48735=EDGE_CURVE ( 'NONE', #68783, #4380, #73249, .T. ) ;
#48756=CIRCLE ( 'NONE', #42985, 5.041900000000000048 ) ;
#48773=VERTEX_POINT ( 'NONE', #36956 ) ;
#48797=ORIENTED_EDGE ( 'NONE', *, *, #53651, .T. ) ;
#48803=DIRECTION ( 'NONE',  ( 0.8660254037844379305, 0.000000000000000000, -0.5000000000000011102 ) ) ;
#48805=CARTESIAN_POINT ( 'NONE',  ( 0.000000000000000000, 101.5999999999999943, 188.9759999999999991 ) ) ;
#48809=B_SPLINE_CURVE_WITH_KNOTS ( 'NONE', 3,
 ( #81363, #12752, #11, #6369, #88614, #74067, #34060, #60422, #61764, #41321, #6816, #34519, #88169, #19104, #46787, #77662, #84034, #14988, #21810, #49927, #69502, #8629, #56751, #28602, #56290, #42657, #48575, #84940, #43111, #15443, #29062, #76309, #8170, #41767, #36323, #21349, #7277, #905, #14543, #55388, #49480, #83585, #20902, #42221, #49023, #14082, #69950, #70857, #84497 ),
 .UNSPECIFIED., .F., .F.,
 ( 4, 2, 2, 2, 2, 2, 2, 2, 2, 2, 2, 2, 2, 2, 2, 1, 2, 2, 2, 2, 2, 2, 2, 2, 4 ),
 ( 0.01987186023414421951, 0.02111356671950570182, 0.02235527320486718761, 0.02483868617559015918, 0.02608039266095162761, 0.02732209914631309605, 0.02980551211703602946, 0.03228892508775896286, 0.03353063157312041048, 0.03477233805848185116, 0.03725575102920475334, 0.03849745751456622178, 0.03973916399992768328, 0.04222257697065066873, 0.04346428345601213716, 0.04470598994137360560, 0.04594769642673506710, 0.04718940291209652860, 0.04967281588281945159, 0.05091452236818091309, 0.05215622885354237459, 0.05463964182426531146, 0.05588134830962682154, 0.05712305479498831773, 0.05960646776571126848 ),
 .UNSPECIFIED. ) ;
#48812=ORIENTED_EDGE ( 'NONE', *, *, #28939, .T. ) ;
#48814=VECTOR ( 'NONE', #44554, 1000.000000000000000 ) ;
#48828=CARTESIAN_POINT ( 'NONE',  ( 130.4363378768869381, 71.14122173980733521, 5.641126054321851768 ) ) ;
#48838=DIRECTION ( 'NONE',  ( 0.000000000000000000, -1.000000000000000000, 0.000000000000000000 ) ) ;
#48860=CARTESIAN_POINT ( 'NONE',  ( -7.941868552260229762E-13, 120.6499999999999915, 107.7702177616926065 ) ) ;
#48881=VECTOR ( 'NONE', #63637, 1000.000000000000114 ) ;
#48888=CARTESIAN_POINT ( 'NONE',  ( 83.40142812120517135, 86.64186789594788252, 100.4448767513726466 ) ) ;
#48890=DIRECTION ( 'NONE',  ( 0.7071067811865510144, 0.000000000000000000, -0.7071067811865441310 ) ) ;
#48902=CARTESIAN_POINT ( 'NONE',  ( 3.968749999999229949, 120.6499999999999915, 100.8961411191535973 ) ) ;
#48911=CARTESIAN_POINT ( 'NONE',  ( -9.572570118836543074, 90.93799233918605296, 118.1704038715884053 ) ) ;
#48920=CARTESIAN_POINT ( 'NONE',  ( -72.96458098368751166, 127.0000000000000000, 65.02708098368620426 ) ) ;
#48925=DIRECTION ( 'NONE',  ( 0.000000000000000000, 0.000000000000000000, -1.000000000000000000 ) ) ;
#48954=VECTOR ( 'NONE', #52944, 1000.000000000000000 ) ;
#48988=CARTESIAN_POINT ( 'NONE',  ( -7.301849239715819957E-13, 120.6499999999999915, 98.60478223830740774 ) ) ;
#48997=CARTESIAN_POINT ( 'NONE',  ( -86.67392531623309537, 94.60304557064715425, 80.89343850130832436 ) ) ;
#49002=CARTESIAN_POINT ( 'NONE',  ( -118.1709372608868875, 90.93089219781630561, 9.551212252129760216 ) ) ;
#49005=CARTESIAN_POINT ( 'NONE',  ( 91.11526841082624628, 75.84278307195158675, -75.85240403722320934 ) ) ;
#49023=CARTESIAN_POINT ( 'NONE',  ( 74.70172715947563802, 85.83559868056556752, -92.06080542007434531 ) ) ;
#49079=CARTESIAN_POINT ( 'NONE',  ( 95.16559702356694572, 70.52006616879377532, -89.37861919290396884 ) ) ;
#49090=CARTESIAN_POINT ( 'NONE',  ( 12.03342778677654934, 78.46830267626332045, 117.9437853765525404 ) ) ;
#49097=EDGE_LOOP ( 'NONE', ( #84250, #88316, #4252, #501 ) ) ;
#49109=CARTESIAN_POINT ( 'NONE',  ( -91.13743891206615899, 69.93117631934792655, 93.48535127324173288 ) ) ;
#49113=VECTOR ( 'NONE', #53907, 1000.000000000000000 ) ;
#49124=EDGE_LOOP ( 'NONE', ( #78012, #50676, #58169, #71982 ) ) ;
#49133=AXIS2_PLACEMENT_3D ( 'NONE', #11508, #4694, #19656 ) ;
#49155=ORIENTED_EDGE ( 'NONE', *, *, #45351, .F. ) ;
#49157=CARTESIAN_POINT ( 'NONE',  ( 12.70000000000000284, 83.38971874880476776, 117.8738102209307783 ) ) ;
#49172=CARTESIAN_POINT ( 'NONE',  ( 77.39114642429960611, 127.0000000000000000, -71.77848634863110533 ) ) ;
#49178=VERTEX_POINT ( 'NONE', #1452 ) ;
#49188=CARTESIAN_POINT ( 'NONE',  ( 7.746212673614271793, 92.64801822704204426, -118.3046725678181446 ) ) ;
#49189=CARTESIAN_POINT ( 'NONE',  ( -1.663881452865377808, 95.14749909259209915, 130.5460625349953432 ) ) ;
#49192=ADVANCED_FACE ( 'NONE', ( #83673 ), #20990, .F. ) ;
#49253=EDGE_LOOP ( 'NONE', ( #45878, #51689, #36988, #88832 ) ) ;
#49254=VERTEX_POINT ( 'NONE', #21894 ) ;
#49256=ADVANCED_FACE ( 'NONE', ( #35050 ), #35957, .F. ) ;
#49265=ORIENTED_EDGE ( 'NONE', *, *, #82925, .T. ) ;
#49283=CARTESIAN_POINT ( 'NONE',  ( -118.1052286201201298, 89.94786999841839759, 10.33119577496824526 ) ) ;
#49285=DIRECTION ( 'NONE',  ( 0.000000000000000000, 1.000000000000000000, 0.000000000000000000 ) ) ;
#49288=CARTESIAN_POINT ( 'NONE',  ( 130.4017839623309953, 71.54617234588344843, -6.354402276674679939 ) ) ;
#49293=FACE_BOUND ( 'NONE', #28192, .T. ) ;
#49299=LINE ( 'NONE', #63392, #68822 ) ;
#49319=AXIS2_PLACEMENT_3D ( 'NONE', #73605, #88596, #74953 ) ;
#49320=LINE ( 'NONE', #43849, #50704 ) ;
#49329=ORIENTED_EDGE ( 'NONE', *, *, #70020, .F. ) ;
#49338=ORIENTED_EDGE ( 'NONE', *, *, #62002, .F. ) ;
#49348=CARTESIAN_POINT ( 'NONE',  ( 100.0339087179658577, 88.18319050751493648, 83.89391322244469507 ) ) ;
#49355=DIRECTION ( 'NONE',  ( 0.000000000000000000, 1.000000000000000000, 0.000000000000000000 ) ) ;
#49359=EDGE_CURVE ( 'NONE', #40480, #58480, #58187, .T. ) ;
#49371=ADVANCED_FACE ( 'NONE', ( #22793 ), #57739, .F. ) ;
#49372=CARTESIAN_POINT ( 'NONE',  ( -6.715083999775230517, 93.33742752469728998, 118.3661748111209704 ) ) ;
#49384=CARTESIAN_POINT ( 'NONE',  ( 12.61957378781718297, 80.89607376620493540, -117.8825615626982994 ) ) ;
#49387=CIRCLE ( 'NONE', #13164, 190.5000000000000000 ) ;
#49411=ORIENTED_EDGE ( 'NONE', *, *, #48735, .T. ) ;
#49418=DIRECTION ( 'NONE',  ( 0.000000000000000000, 0.000000000000000000, 1.000000000000000000 ) ) ;
#49480=CARTESIAN_POINT ( 'NONE',  ( 75.67533895324405080, 88.91291927174617626, -91.26325766987429233 ) ) ;
#49499=ORIENTED_EDGE ( 'NONE', *, *, #22843, .F. ) ;
#49503=ORIENTED_EDGE ( 'NONE', *, *, #77024, .T. ) ;
#49504=ORIENTED_EDGE ( 'NONE', *, *, #69822, .F. ) ;
#49508=CARTESIAN_POINT ( 'NONE',  ( -5.627553765716396761, 71.15732062108085643, -130.4351721735936280 ) ) ;
#49513=CARTESIAN_POINT ( 'NONE',  ( -71.77848634863029531, 127.0000000000000000, -77.39114642430038771 ) ) ;
#49516=CYLINDRICAL_SURFACE ( 'NONE', #40781, 7.937500000000000000 ) ;
#49532=CARTESIAN_POINT ( 'NONE',  ( 85.52748787272849995, 73.86195533656248813, -98.64078293412647724 ) ) ;
#49547=CARTESIAN_POINT ( 'NONE',  ( -77.89700433585329620, 82.54999999999999716, -59.93649209371570663 ) ) ;
#49559=CARTESIAN_POINT ( 'NONE',  ( -92.91726854070100217, 69.85063703626886422, 91.71670967180014600 ) ) ;
#49573=DIRECTION ( 'NONE',  ( -3.576143065239989638E-15, 0.000000000000000000, 1.000000000000000000 ) ) ;
#49581=CARTESIAN_POINT ( 'NONE',  ( -76.38857008572975360, 90.29828471680511370, -90.66710916952459343 ) ) ;
#49597=EDGE_CURVE ( 'NONE', #36775, #24180, #40420, .T. ) ;
#49640=CARTESIAN_POINT ( 'NONE',  ( 11.39384497175739064, 88.17529471328433033, -118.0073914794113961 ) ) ;
#49652=CARTESIAN_POINT ( 'NONE',  ( 3.063943826786759644E-15, 125.7300000000000040, 24.63800000000000168 ) ) ;
#49678=ORIENTED_EDGE ( 'NONE', *, *, #63491, .T. ) ;
#49698=CARTESIAN_POINT ( 'NONE',  ( 12.03356702080700202, 78.46872568947895843, 130.0002966128845969 ) ) ;
#49699=CARTESIAN_POINT ( 'NONE',  ( -99.78216974382876003, 88.91243380484087311, -84.19383299529374654 ) ) ;
#49710=CARTESIAN_POINT ( 'NONE',  ( 71.77848634863079269, 120.6499999999999915, 77.39114642429989033 ) ) ;
#49712=ORIENTED_EDGE ( 'NONE', *, *, #67648, .T. ) ;
#49725=CARTESIAN_POINT ( 'NONE',  ( -7.941868552260229762E-13, 120.6499999999999915, 107.7702177616926065 ) ) ;
#49738=CARTESIAN_POINT ( 'NONE',  ( 130.0004344034681765, 78.46444036551649504, 12.03207709110674806 ) ) ;
#49753=CIRCLE ( 'NONE', #83109, 130.5560000000000116 ) ;
#49768=DIRECTION ( 'NONE',  ( 0.7071067811865441310, 0.000000000000000000, 0.7071067811865510144 ) ) ;
#49782=EDGE_CURVE ( 'NONE', #12034, #61226, #19589, .T. ) ;
#49790=EDGE_LOOP ( 'NONE', ( #50797, #27997, #26534, #89729 ) ) ;
#49796=CARTESIAN_POINT ( 'NONE',  ( 82.97845804870276254, 84.21348395916255924, 100.7940789023230508 ) ) ;
#49805=DIRECTION ( 'NONE',  ( 0.000000000000000000, 0.000000000000000000, -1.000000000000000000 ) ) ;
#49811=DIRECTION ( 'NONE',  ( 0.8660254037844392627, 0.000000000000000000, -0.4999999999999990008 ) ) ;
#49835=EDGE_LOOP ( 'NONE', ( #43545, #70199, #82842, #89839 ) ) ;
#49836=CARTESIAN_POINT ( 'NONE',  ( 0.000000000000000000, 125.7300000000000040, -24.63800000000000168 ) ) ;
#49854=FACE_BOUND ( 'NONE', #86199, .T. ) ;
#49863=ORIENTED_EDGE ( 'NONE', *, *, #8810, .T. ) ;
#49871=AXIS2_PLACEMENT_3D ( 'NONE', #56275, #42208, #892 ) ;
#49898=CARTESIAN_POINT ( 'NONE',  ( -68.91674821478457602, 82.54999999999999716, 68.91674821478434865 ) ) ;
#49909=CARTESIAN_POINT ( 'NONE',  ( 103.1875000000000000, 101.5999999999999943, -5.041899999999640336 ) ) ;
#49927=CARTESIAN_POINT ( 'NONE',  ( 86.67392531623372065, 94.60304557064719688, -80.89343850130777014 ) ) ;
#49953=EDGE_CURVE ( 'NONE', #51660, #9633, #76334, .T. ) ;
#49975=DIRECTION ( 'NONE',  ( 0.000000000000000000, -1.000000000000000000, 0.000000000000000000 ) ) ;
#49980=CARTESIAN_POINT ( 'NONE',  ( 82.96304607088339367, 80.88456863959029874, -100.8068867829400688 ) ) ;
#50028=CARTESIAN_POINT ( 'NONE',  ( -74.68844285250172277, 85.85031469618034805, -92.07164801315032321 ) ) ;
#50035=VERTEX_POINT ( 'NONE', #15194 ) ;
#50039=EDGE_CURVE ( 'NONE', #61226, #46913, #81404, .T. ) ;
#50068=ORIENTED_EDGE ( 'NONE', *, *, #74813, .T. ) ;
#50078=DIRECTION ( 'NONE',  ( 0.000000000000000000, 0.000000000000000000, 1.000000000000000000 ) ) ;
#50082=CARTESIAN_POINT ( 'NONE',  ( 0.000000000000000000, 124.5870000000000033, 0.000000000000000000 ) ) ;
#50102=AXIS2_PLACEMENT_3D ( 'NONE', #46364, #17790, #3715 ) ;
#50105=CARTESIAN_POINT ( 'NONE',  ( -76.20505178924278766, 127.0000000000000000, -76.20505178924469192 ) ) ;
#50140=CARTESIAN_POINT ( 'NONE',  ( 6.359898342742077659, 71.54935466043629333, 130.4015153071888733 ) ) ;
#50166=EDGE_CURVE ( 'NONE', #81111, #2816, #45539, .T. ) ;
#50168=ORIENTED_EDGE ( 'NONE', *, *, #52165, .F. ) ;
#50177=DIRECTION ( 'NONE',  ( -0.9659258262890686453, 0.000000000000000000, 0.2588190451025194072 ) ) ;
#50192=LINE ( 'NONE', #42035, #19555 ) ;
#50215=CIRCLE ( 'NONE', #76287, 7.143750000000001599 ) ;
#50216=CARTESIAN_POINT ( 'NONE',  ( -3.174999999999664979, 104.3431970271541616, -31.75000000000000000 ) ) ;
#50238=ORIENTED_EDGE ( 'NONE', *, *, #24921, .F. ) ;
#50242=DIRECTION ( 'NONE',  ( 0.000000000000000000, 1.000000000000000000, 0.000000000000000000 ) ) ;
#50243=CARTESIAN_POINT ( 'NONE',  ( 98.82361644294680048, 90.93081950567960803, 85.31607583734509603 ) ) ;
#50264=DIRECTION ( 'NONE',  ( 0.000000000000000000, 1.000000000000000000, 0.000000000000000000 ) ) ;
#50284=EDGE_CURVE ( 'NONE', #2396, #76220, #15528, .T. ) ;
#50289=AXIS2_PLACEMENT_3D ( 'NONE', #73057, #58095, #16324 ) ;
#50292=EDGE_CURVE ( 'NONE', #14878, #70474, #24900, .T. ) ;
#50293=CARTESIAN_POINT ( 'NONE',  ( -59.93649209371543662, 82.54999999999999716, 77.89700433585352357 ) ) ;
#50308=CARTESIAN_POINT ( 'NONE',  ( -77.39114642429849766, 120.6499999999999915, -71.77848634863219957 ) ) ;
#50317=VECTOR ( 'NONE', #7624, 1000.000000000000114 ) ;
#50318=CARTESIAN_POINT ( 'NONE',  ( 85.30119219530003249, 74.16222525595215131, 98.83784439188701754 ) ) ;
#50355=CARTESIAN_POINT ( 'NONE',  ( -76.80574412431003850, 90.93089219781633403, 90.31319802837631983 ) ) ;
#50362=ORIENTED_EDGE ( 'NONE', *, *, #17250, .F. ) ;
#50390=DIRECTION ( 'NONE',  ( 0.000000000000000000, 1.000000000000000000, 0.000000000000000000 ) ) ;
#50407=EDGE_CURVE ( 'NONE', #49254, #43486, #51811, .T. ) ;
#50415=DIRECTION ( 'NONE',  ( 0.000000000000000000, 0.000000000000000000, 1.000000000000000000 ) ) ;
#50419=VERTEX_POINT ( 'NONE', #38640 ) ;
#50450=DIRECTION ( 'NONE',  ( 1.000000000000000000, 0.000000000000000000, 1.047444401652940007E-14 ) ) ;
#50472=CARTESIAN_POINT ( 'NONE',  ( -97.63151088911699560, 92.64985122628468162, 86.68005309089153343 ) ) ;
#50486=DIRECTION ( 'NONE',  ( 0.000000000000000000, -1.000000000000000000, 0.000000000000000000 ) ) ;
#50500=FACE_OUTER_BOUND ( 'NONE', #847, .T. ) ;
#50505=LINE ( 'NONE', #36888, #46411 ) ;
#50507=EDGE_CURVE ( 'NONE', #68541, #73425, #53131, .T. ) ;
#50590=ORIENTED_EDGE ( 'NONE', *, *, #46817, .T. ) ;
#50591=ORIENTED_EDGE ( 'NONE', *, *, #78325, .T. ) ;
#50595=CARTESIAN_POINT ( 'NONE',  ( 9.275599959524004845, 73.86527412294591954, 130.2264118494045420 ) ) ;
#50596=DIRECTION ( 'NONE',  ( 0.000000000000000000, 1.000000000000000000, 0.000000000000000000 ) ) ;
#50616=ORIENTED_EDGE ( 'NONE', *, *, #81613, .T. ) ;
#50654=AXIS2_PLACEMENT_3D ( 'NONE', #76770, #14557, #20914 ) ;
#50656=AXIS2_PLACEMENT_3D ( 'NONE', #89656, #19265, #5642 ) ;
#50666=AXIS2_PLACEMENT_3D ( 'NONE', #10225, #80617, #37930 ) ;
#50675=ORIENTED_EDGE ( 'NONE', *, *, #9694, .F. ) ;
#50676=ORIENTED_EDGE ( 'NONE', *, *, #8871, .F. ) ;
#50704=VECTOR ( 'NONE', #70227, 1000.000000000000000 ) ;
#50720=STYLED_ITEM ( 'NONE', ( #46835 ), #43438 ) ;
#50729=EDGE_LOOP ( 'NONE', ( #1659, #60375 ) ) ;
#50738=EDGE_CURVE ( 'NONE', #65614, #16533, #42214, .T. ) ;
#50745=FACE_BOUND ( 'NONE', #12075, .T. ) ;
#50770=AXIS2_PLACEMENT_3D ( 'NONE', #38372, #51109, #59698 ) ;
#50778=LINE ( 'NONE', #22199, #45996 ) ;
#50779=DIRECTION ( 'NONE',  ( 0.000000000000000000, 1.000000000000000000, 0.000000000000000000 ) ) ;
#50785=VERTEX_POINT ( 'NONE', #13628 ) ;
#50792=CARTESIAN_POINT ( 'NONE',  ( 78.17938156622449242, 72.47328848629021536, 89.12695577293618499 ) ) ;
#50797=ORIENTED_EDGE ( 'NONE', *, *, #42189, .T. ) ;
#50811=EDGE_CURVE ( 'NONE', #73425, #76987, #52140, .T. ) ;
#50813=EDGE_LOOP ( 'NONE', ( #62660, #34171, #30146, #79045, #69754, #44127 ) ) ;
#50824=CARTESIAN_POINT ( 'NONE',  ( 72.96458098368650269, 127.0000000000000000, 72.96458098368729850 ) ) ;
#50834=DIRECTION ( 'NONE',  ( -0.7071067811865487940, 0.000000000000000000, 0.7071067811865463515 ) ) ;
#50852=CARTESIAN_POINT ( 'NONE',  ( -33.98325472291465132, 104.3431970271541900, 3.174999999999764899 ) ) ;
#50854=FACE_OUTER_BOUND ( 'NONE', #81041, .T. ) ;
#50897=DIRECTION ( 'NONE',  ( 3.491483361109385222E-15, 0.000000000000000000, -1.000000000000000000 ) ) ;
#50913=AXIS2_PLACEMENT_3D ( 'NONE', #42144, #9434, #42583 ) ;
#50914=EDGE_CURVE ( 'NONE', #3056, #76987, #36765, .T. ) ;
#50921=CARTESIAN_POINT ( 'NONE',  ( -12.70000000000000107, 82.54999999999999716, 97.46299999999996544 ) ) ;
#50923=CARTESIAN_POINT ( 'NONE',  ( -93.77212533081346635, 95.08644067748863904, 90.83954799657482226 ) ) ;
#50943=ORIENTED_EDGE ( 'NONE', *, *, #21826, .F. ) ;
#51020=AXIS2_PLACEMENT_3D ( 'NONE', #58074, #66216, #85366 ) ;
#51027=VECTOR ( 'NONE', #41270, 1000.000000000000000 ) ;
#51038=CARTESIAN_POINT ( 'NONE',  ( -7.199374239792870816E-13, 127.0000000000000000, 98.14560000000000173 ) ) ;
#51079=CARTESIAN_POINT ( 'NONE',  ( -130.2266331669275985, 73.86195533656248813, 9.272499861615250083 ) ) ;
#51081=CIRCLE ( 'NONE', #29321, 7.937500000000000000 ) ;
#51082=ORIENTED_EDGE ( 'NONE', *, *, #74527, .T. ) ;
#51083=AXIS2_PLACEMENT_3D ( 'NONE', #15832, #57599, #43960 ) ;
#51107=LINE ( 'NONE', #43396, #12655 ) ;
#51109=DIRECTION ( 'NONE',  ( 0.000000000000000000, 1.000000000000000000, 0.000000000000000000 ) ) ;
#51128=ADVANCED_FACE ( 'NONE', ( #13971, #83462 ), #61650, .F. ) ;
#51179=CARTESIAN_POINT ( 'NONE',  ( 0.000000000000000000, 124.5870000000000033, -25.39999999999999858 ) ) ;
#51195=DIRECTION ( 'NONE',  ( 0.000000000000000000, 1.000000000000000000, 0.000000000000000000 ) ) ;
#51198=FACE_OUTER_BOUND ( 'NONE', #79237, .T. ) ;
#51207=CARTESIAN_POINT ( 'NONE',  ( 83.41622542100820681, 78.46444036551646661, 100.4321520267703249 ) ) ;
#51212=VECTOR ( 'NONE', #36000, 1000.000000000000114 ) ;
#51216=B_SPLINE_CURVE_WITH_KNOTS ( 'NONE', 3,
 ( #10488, #30492, #85921, #44542, #85027, #45427, #38188, #65885, #3673, #59060, #24566, #23691, #17751, #85480, #50472, #2794, #44094, #36422, #51355, #3236, #9157, #50923, #22797, #78214, #36856, #30930, #58619, #15976, #43656, #9597, #37305, #79100, #65010, #16862, #52673, #73145, #4115, #46320, #46768, #25451, #32710, #88591, #39074, #53117, #74499, #60860, #80889, #4569, #31814 ),
 .UNSPECIFIED., .F., .F.,
 ( 4, 2, 2, 2, 2, 2, 2, 2, 2, 2, 2, 2, 2, 2, 2, 1, 2, 2, 2, 2, 2, 2, 2, 2, 4 ),
 ( 0.01986933033599076748, 0.02111088875730818271, 0.02235244717862559446, 0.02483556402126041798, 0.02607712244257780546, 0.02731868086389519293, 0.02980179770652992971, 0.03228491454916466996, 0.03352647297048201580, 0.03476803139179936164, 0.03725114823443406720, 0.03849270665575145467, 0.03973426507706884214, 0.04221738191970363097, 0.04345894034102103232, 0.04470049876233841979, 0.04594205718365582114, 0.04718361560497322249, 0.04966673244760801131, 0.05090829086892539879, 0.05214984929024277238, 0.05463296613287750569, 0.05587452455419486541, 0.05711608297551221819, 0.05959919981814693762 ),
 .UNSPECIFIED. ) ;
#51224=CARTESIAN_POINT ( 'NONE',  ( 78.43243611888021860, 72.22378176823139029, 88.90442867306012431 ) ) ;
#51234=DIRECTION ( 'NONE',  ( 0.000000000000000000, -1.000000000000000000, 0.000000000000000000 ) ) ;
#51275=CARTESIAN_POINT ( 'NONE',  ( 69.72411017812960665, 120.6499999999999915, 69.72411017813040246 ) ) ;
#51298=ORIENTED_EDGE ( 'NONE', *, *, #62048, .F. ) ;
#51307=EDGE_CURVE ( 'NONE', #32868, #62133, #9749, .T. ) ;
#51329=DIRECTION ( 'NONE',  ( 0.000000000000000000, 1.000000000000000000, 0.000000000000000000 ) ) ;
#51331=AXIS2_PLACEMENT_3D ( 'NONE', #81070, #46501, #74237 ) ;
#51349=ORIENTED_EDGE ( 'NONE', *, *, #9694, .T. ) ;
#51355=CARTESIAN_POINT ( 'NONE',  ( -95.94886839522581568, 94.12569442554139698, 88.53717826876649610 ) ) ;
#51369=DIRECTION ( 'NONE',  ( 0.000000000000000000, -1.000000000000000000, 0.000000000000000000 ) ) ;
#51413=ORIENTED_EDGE ( 'NONE', *, *, #80457, .F. ) ;
#51424=CYLINDRICAL_SURFACE ( 'NONE', #75875, 25.39999999999999858 ) ;
#51441=DIRECTION ( 'NONE',  ( 1.000000000000000000, 0.000000000000000000, 0.000000000000000000 ) ) ;
#51459=VECTOR ( 'NONE', #82874, 1000.000000000000000 ) ;
#51467=CARTESIAN_POINT ( 'NONE',  ( 118.5108917117887160, 70.27763793881258891, 3.294392537550968392 ) ) ;
#51569=ORIENTED_EDGE ( 'NONE', *, *, #39725, .F. ) ;
#51571=VERTEX_POINT ( 'NONE', #3325 ) ;
#51583=ORIENTED_EDGE ( 'NONE', *, *, #9680, .T. ) ;
#51591=ADVANCED_FACE ( 'NONE', ( #10573 ), #45514, .T. ) ;
#51592=AXIS2_PLACEMENT_3D ( 'NONE', #67373, #5164, #46021 ) ;
#51643=CARTESIAN_POINT ( 'NONE',  ( 0.000000000000000000, 61.59999999999999432, 0.000000000000000000 ) ) ;
#51660=VERTEX_POINT ( 'NONE', #72777 ) ;
#51669=CARTESIAN_POINT ( 'NONE',  ( 80.88853703239254855, 70.52018178143200089, 86.67600044576384732 ) ) ;
#51682=EDGE_CURVE ( 'NONE', #29480, #67802, #31421, .T. ) ;
#51689=ORIENTED_EDGE ( 'NONE', *, *, #27667, .F. ) ;
#51738=AXIS2_PLACEMENT_3D ( 'NONE', #22146, #49811, #23921 ) ;
#51762=AXIS2_PLACEMENT_3D ( 'NONE', #2615, #86624, #72098 ) ;
#51776=ORIENTED_EDGE ( 'NONE', *, *, #16463, .T. ) ;
#51780=DIRECTION ( 'NONE',  ( 0.2588190451025154659, 0.000000000000000000, 0.9659258262890696445 ) ) ;
#51783=CARTESIAN_POINT ( 'NONE',  ( 72.96458098368650269, 101.5999999999999943, 67.92268098368730023 ) ) ;
#51789=CIRCLE ( 'NONE', #8312, 5.041900000000001825 ) ;
#51809=CIRCLE ( 'NONE', #72142, 5.041900000000001825 ) ;
#51810=EDGE_CURVE ( 'NONE', #29308, #7172, #85974, .T. ) ;
#51811=LINE ( 'NONE', #65465, #48814 ) ;
#51845=CARTESIAN_POINT ( 'NONE',  ( -12.03144885753538595, 78.46257116061715919, 130.0004926519013111 ) ) ;
#51847=EDGE_CURVE ( 'NONE', #54367, #5023, #32312, .T. ) ;
#51863=DIRECTION ( 'NONE',  ( 0.000000000000000000, 0.000000000000000000, -1.000000000000000000 ) ) ;
#51879=EDGE_LOOP ( 'NONE', ( #69986, #3693, #40332, #68788 ) ) ;
#51882=ORIENTED_EDGE ( 'NONE', *, *, #88673, .T. ) ;
#51900=CARTESIAN_POINT ( 'NONE',  ( -103.1875000000000000, 127.0000000000000000, -7.937500000001080913 ) ) ;
#51902=EDGE_CURVE ( 'NONE', #81089, #49254, #11286, .T. ) ;
#51903=CARTESIAN_POINT ( 'NONE',  ( 118.5469577077832497, 69.93366089391886931, 1.674277437723032502 ) ) ;
#51924=ORIENTED_EDGE ( 'NONE', *, *, #6749, .F. ) ;
#51940=PLANE ( 'NONE',  #44428 ) ;
#51951=DIRECTION ( 'NONE',  ( -1.000000000000000000, 0.000000000000000000, -3.491483361109380094E-15 ) ) ;
#51962=LINE ( 'NONE', #9005, #56623 ) ;
#51992=VECTOR ( 'NONE', #84716, 1000.000000000000000 ) ;
#51993=CARTESIAN_POINT ( 'NONE',  ( -10.33024153997673089, 89.94921403597288645, -130.1468737228267685 ) ) ;
#52004=ORIENTED_EDGE ( 'NONE', *, *, #10710, .T. ) ;
#52015=LINE ( 'NONE', #4792, #53222 ) ;
#52017=CARTESIAN_POINT ( 'NONE',  ( 78.17826422383464546, 92.64969027323469675, 89.13001032377241017 ) ) ;
#52026=CIRCLE ( 'NONE', #56384, 5.041900000000001825 ) ;
#52043=ORIENTED_EDGE ( 'NONE', *, *, #44642, .T. ) ;
#52084=EDGE_LOOP ( 'NONE', ( #81377, #37547 ) ) ;
#52103=CARTESIAN_POINT ( 'NONE',  ( 88.44575049335495009, 71.76236341258000095, 78.94931995840828165 ) ) ;
#52116=CARTESIAN_POINT ( 'NONE',  ( 118.0645351272586510, 89.26692529358290074, 10.78628659036793813 ) ) ;
#52128=CYLINDRICAL_SURFACE ( 'NONE', #63882, 12.70000000000000107 ) ;
#52132=CARTESIAN_POINT ( 'NONE',  ( 92.05992619857352111, 79.25941250729452747, -74.70281015415415027 ) ) ;
#52140=LINE ( 'NONE', #31270, #59058 ) ;
#52161=EDGE_LOOP ( 'NONE', ( #87733, #35653, #66378, #31898 ) ) ;
#52165=EDGE_CURVE ( 'NONE', #82562, #8401, #17205, .T. ) ;
#52202=ORIENTED_EDGE ( 'NONE', *, *, #69170, .T. ) ;
#52207=CARTESIAN_POINT ( 'NONE',  ( 2.323620343766204915E-14, 127.0000000000000000, 188.9759999999999991 ) ) ;
#52216=LINE ( 'NONE', #24996, #57416 ) ;
#52222=EDGE_CURVE ( 'NONE', #57775, #76254, #56268, .T. ) ;
#52236=CYLINDRICAL_SURFACE ( 'NONE', #47330, 7.937500000000000000 ) ;
#52254=ORIENTED_EDGE ( 'NONE', *, *, #13297, .T. ) ;
#52263=ORIENTED_EDGE ( 'NONE', *, *, #50738, .F. ) ;
#52271=ORIENTED_EDGE ( 'NONE', *, *, #11484, .F. ) ;
#52273=CARTESIAN_POINT ( 'NONE',  ( -12.70000000000000107, 82.54999999999999716, -129.9368274816650910 ) ) ;
#52274=EDGE_CURVE ( 'NONE', #1981, #9843, #73491, .T. ) ;
#52280=VECTOR ( 'NONE', #65663, 1000.000000000000000 ) ;
#52315=CARTESIAN_POINT ( 'NONE',  ( -31.75000000000000000, 124.5870000000000033, -3.175000000000219647 ) ) ;
#52316=VERTEX_POINT ( 'NONE', #9899 ) ;
#52327=CARTESIAN_POINT ( 'NONE',  ( -82.96304607088271155, 80.88456863959031296, 100.8068867829406514 ) ) ;
#52339=CARTESIAN_POINT ( 'NONE',  ( 118.5107509192928887, 70.27900073646854651, -3.299277431128419202 ) ) ;
#52343=DIRECTION ( 'NONE',  ( 1.000000000000000000, 0.000000000000000000, 0.000000000000000000 ) ) ;
#52347=ORIENTED_EDGE ( 'NONE', *, *, #52721, .F. ) ;
#52355=AXIS2_PLACEMENT_3D ( 'NONE', #38473, #17160, #79845 ) ;
#52363=CARTESIAN_POINT ( 'NONE',  ( -7.736705052999859333, 72.46990138899384704, 118.3037342042693325 ) ) ;
#52385=CYLINDRICAL_SURFACE ( 'NONE', #48496, 7.937500000000000000 ) ;
#52389=CARTESIAN_POINT ( 'NONE',  ( 0.000000000000000000, 125.7300000000000040, -24.63800000000000168 ) ) ;
#52455=FACE_OUTER_BOUND ( 'NONE', #5710, .T. ) ;
#52461=EDGE_CURVE ( 'NONE', #24254, #45930, #38476, .T. ) ;
#52484=VERTEX_POINT ( 'NONE', #38927 ) ;
#52485=VERTEX_POINT ( 'NONE', #66634 ) ;
#52494=FACE_BOUND ( 'NONE', #41556, .T. ) ;
#52496=CARTESIAN_POINT ( 'NONE',  ( 129.9368274816652331, 82.54999999999999716, -12.69999999999864038 ) ) ;
#52497=ORIENTED_EDGE ( 'NONE', *, *, #3565, .T. ) ;
#52507=EDGE_CURVE ( 'NONE', #72426, #8076, #70225, .T. ) ;
#52512=CARTESIAN_POINT ( 'NONE',  ( -72.96458098368600531, 127.0000000000000000, -72.96458098368781009 ) ) ;
#52516=ORIENTED_EDGE ( 'NONE', *, *, #20254, .F. ) ;
#52545=CIRCLE ( 'NONE', #1828, 7.937500000000000000 ) ;
#52552=ORIENTED_EDGE ( 'NONE', *, *, #86485, .T. ) ;
#52553=ORIENTED_EDGE ( 'NONE', *, *, #77372, .F. ) ;
#52554=CIRCLE ( 'NONE', #9097, 7.937500000000000000 ) ;
#52560=CARTESIAN_POINT ( 'NONE',  ( 117.8848147242575237, 84.21376545118702950, 12.59751181725513014 ) ) ;
#52573=EDGE_LOOP ( 'NONE', ( #69725, #33604 ) ) ;
#52587=PLANE ( 'NONE',  #7529 ) ;
#52593=CARTESIAN_POINT ( 'NONE',  ( -118.2598914205052409, 72.98405218941672956, 8.394510633990522663 ) ) ;
#52626=ADVANCED_FACE ( 'NONE', ( #72465 ), #78406, .F. ) ;
#52630=CARTESIAN_POINT ( 'NONE',  ( 103.1875000000000000, 127.0000000000000000, 3.602774393244745134E-13 ) ) ;
#52648=CARTESIAN_POINT ( 'NONE',  ( 100.7545871043110424, 84.62817240485476589, -83.02643542997968495 ) ) ;
#52650=PLANE ( 'NONE',  #35634 ) ;
#52673=CARTESIAN_POINT ( 'NONE',  ( -86.67213519546623957, 92.64237678566782108, 97.63858630140191508 ) ) ;
#52687=LINE ( 'NONE', #54485, #43284 ) ;
#52713=ORIENTED_EDGE ( 'NONE', *, *, #70922, .T. ) ;
#52721=EDGE_CURVE ( 'NONE', #82989, #5511, #51107, .T. ) ;
#52723=ADVANCED_FACE ( 'NONE', ( #22990 ), #15270, .F. ) ;
#52774=DIRECTION ( 'NONE',  ( 0.000000000000000000, -1.000000000000000000, 0.000000000000000000 ) ) ;
#52775=DIRECTION ( 'NONE',  ( 0.000000000000000000, 1.000000000000000000, 0.000000000000000000 ) ) ;
#52776=DIRECTION ( 'NONE',  ( 0.000000000000000000, -1.000000000000000000, 0.000000000000000000 ) ) ;
#52778=CARTESIAN_POINT ( 'NONE',  ( 117.9582931081851029, 78.06989712577870932, -11.89083204515574721 ) ) ;
#52787=FACE_OUTER_BOUND ( 'NONE', #64258, .T. ) ;
#52796=CARTESIAN_POINT ( 'NONE',  ( -12.03133265694088294, 78.46222587235902779, 117.9439990761035943 ) ) ;
#52807=AXIS2_PLACEMENT_3D ( 'NONE', #75075, #40548, #89157 ) ;
#52846=CARTESIAN_POINT ( 'NONE',  ( -9.270368442002537179, 91.24032474172570062, -118.1933656790129987 ) ) ;
#52858=CYLINDRICAL_SURFACE ( 'NONE', #54358, 7.937500000000000000 ) ;
#52873=VERTEX_POINT ( 'NONE', #18831 ) ;
#52886=CARTESIAN_POINT ( 'NONE',  ( 91.90730674524625954, 86.63388195152282378, 74.89049941105180608 ) ) ;
#52891=CARTESIAN_POINT ( 'NONE',  ( 0.8293186434173880350, 95.25000000000001421, 130.5560000000000116 ) ) ;
#52904=ORIENTED_EDGE ( 'NONE', *, *, #48104, .T. ) ;
#52914=ORIENTED_EDGE ( 'NONE', *, *, #62048, .T. ) ;
#52930=ORIENTED_EDGE ( 'NONE', *, *, #76554, .T. ) ;
#52944=DIRECTION ( 'NONE',  ( 0.000000000000000000, -1.000000000000000000, 0.000000000000000000 ) ) ;
#52947=DIRECTION ( 'NONE',  ( 0.000000000000000000, -0.000000000000000000, -1.000000000000000000 ) ) ;
#52957=FACE_OUTER_BOUND ( 'NONE', #21261, .T. ) ;
#52970=CARTESIAN_POINT ( 'NONE',  ( 12.69999999999999929, 82.96435431876524547, -129.9368274816650626 ) ) ;
#52975=CIRCLE ( 'NONE', #13856, 7.937500000000000000 ) ;
#53000=DIRECTION ( 'NONE',  ( 0.000000000000000000, 1.000000000000000000, 0.000000000000000000 ) ) ;
#53003=VECTOR ( 'NONE', #82672, 1000.000000000000114 ) ;
#53006=FACE_OUTER_BOUND ( 'NONE', #48703, .T. ) ;
#53030=EDGE_LOOP ( 'NONE', ( #80738, #56079, #78921, #58026 ) ) ;
#53031=CARTESIAN_POINT ( 'NONE',  ( -118.5560669097358897, 69.84937538953988678, 0.8299548590975466267 ) ) ;
#53032=ORIENTED_EDGE ( 'NONE', *, *, #34069, .F. ) ;
#53047=DIRECTION ( 'NONE',  ( 0.000000000000000000, 1.000000000000000000, 0.000000000000000000 ) ) ;
#53052=LINE ( 'NONE', #73987, #30991 ) ;
#53076=CARTESIAN_POINT ( 'NONE',  ( -130.4018701889608565, 93.55484823631827851, 6.352633250518059604 ) ) ;
#53090=CARTESIAN_POINT ( 'NONE',  ( 83.52531662946692848, 87.03008507238372715, -100.3414980266870913 ) ) ;
#53094=CARTESIAN_POINT ( 'NONE',  ( -10.08473622792051039, 74.81935728795534146, -118.1266015380916912 ) ) ;
#53117=CARTESIAN_POINT ( 'NONE',  ( -83.41565754067454463, 86.63355734047004830, 100.4326241145872984 ) ) ;
#53131=LINE ( 'NONE', #19096, #60426 ) ;
#53158=CARTESIAN_POINT ( 'NONE',  ( 129.9368274816652331, 82.54999999999999716, -12.69999999999864038 ) ) ;
#53163=AXIS2_PLACEMENT_3D ( 'NONE', #85302, #79374, #23078 ) ;
#53181=CARTESIAN_POINT ( 'NONE',  ( -68.53801554307339927, 127.0000000000000000, -74.15067561874339219 ) ) ;
#53202=AXIS2_PLACEMENT_3D ( 'NONE', #40412, #88583, #74491 ) ;
#53221=CARTESIAN_POINT ( 'NONE',  ( 0.000000000000000000, 61.59999999999999432, 0.000000000000000000 ) ) ;
#53222=VECTOR ( 'NONE', #86577, 1000.000000000000000 ) ;
#53245=CARTESIAN_POINT ( 'NONE',  ( -100.8068867829403956, 80.88456863959032717, -82.96304607088309524 ) ) ;
#53256=ORIENTED_EDGE ( 'NONE', *, *, #73835, .T. ) ;
#53265=VERTEX_POINT ( 'NONE', #38602 ) ;
#53276=ORIENTED_EDGE ( 'NONE', *, *, #16672, .F. ) ;
#53288=AXIS2_PLACEMENT_3D ( 'NONE', #10489, #16863, #25011 ) ;
#53300=CARTESIAN_POINT ( 'NONE',  ( 72.96458098368650269, 117.4749999999999943, 80.10833098368729566 ) ) ;
#53305=DIRECTION ( 'NONE',  ( 0.000000000000000000, 0.000000000000000000, 1.000000000000000000 ) ) ;
#53309=CARTESIAN_POINT ( 'NONE',  ( -12.69999999999999929, 83.38971874880475355, -117.8738102209307641 ) ) ;
#53310=ORIENTED_EDGE ( 'NONE', *, *, #55005, .F. ) ;
#53317=CARTESIAN_POINT ( 'NONE',  ( -72.96458098368751166, 117.4749999999999943, 72.96458098368620426 ) ) ;
#53324=ORIENTED_EDGE ( 'NONE', *, *, #81206, .F. ) ;
#53335=AXIS2_PLACEMENT_3D ( 'NONE', #43146, #64951, #78605 ) ;
#53341=VECTOR ( 'NONE', #2849, 1000.000000000000000 ) ;
#53350=CARTESIAN_POINT ( 'NONE',  ( 82.35292268805442006, 95.08639429146515454, 85.28591416242430512 ) ) ;
#53356=AXIS2_PLACEMENT_3D ( 'NONE', #18128, #72220, #44488 ) ;
#53359=CARTESIAN_POINT ( 'NONE',  ( -83.90854149456433220, 88.17609398443094904, -100.0213216842702906 ) ) ;
#53398=EDGE_LOOP ( 'NONE', ( #88649, #46726, #81026, #36160 ) ) ;
#53426=CARTESIAN_POINT ( 'NONE',  ( 100.2530235599239887, 77.68489675156567387, -83.63178471058850505 ) ) ;
#53429=ORIENTED_EDGE ( 'NONE', *, *, #34876, .F. ) ;
#53444=ORIENTED_EDGE ( 'NONE', *, *, #67423, .T. ) ;
#53446=VERTEX_POINT ( 'NONE', #34016 ) ;
#53449=DIRECTION ( 'NONE',  ( 0.000000000000000000, 1.000000000000000000, 0.000000000000000000 ) ) ;
#53454=CARTESIAN_POINT ( 'NONE',  ( 118.1705221151482164, 90.93965867633431799, 9.571124722858908029 ) ) ;
#53478=ADVANCED_FACE ( 'NONE', ( #8121 ), #84890, .F. ) ;
#53481=CARTESIAN_POINT ( 'NONE',  ( 0.000000000000000000, 127.0000000000000000, -103.1875000000000000 ) ) ;
#53505=ORIENTED_EDGE ( 'NONE', *, *, #76526, .T. ) ;
#53509=CARTESIAN_POINT ( 'NONE',  ( 3.968750000000000000, 120.6499999999999915, -105.4788588808464027 ) ) ;
#53510=CARTESIAN_POINT ( 'NONE',  ( 72.96458098368650269, 117.4749999999999943, 67.92268098368730023 ) ) ;
#53519=VERTEX_POINT ( 'NONE', #63074 ) ;
#53530=CARTESIAN_POINT ( 'NONE',  ( -130.1658227983198515, 90.29814575435200652, -10.09656535537057209 ) ) ;
#53546=CARTESIAN_POINT ( 'NONE',  ( 91.13883569058506851, 95.16896684734909684, -93.48397507443779375 ) ) ;
#53552=CARTESIAN_POINT ( 'NONE',  ( -10.33363185139394957, 75.15554654547490543, -118.1050150300115007 ) ) ;
#53574=CARTESIAN_POINT ( 'NONE',  ( 72.96458098368650269, 127.0000000000000000, 80.90208098368729850 ) ) ;
#53612=CARTESIAN_POINT ( 'NONE',  ( 130.4354318373310946, 93.94566094357732311, 5.621620364687625937 ) ) ;
#53651=EDGE_CURVE ( 'NONE', #5415, #8910, #3985, .T. ) ;
#53656=DIRECTION ( 'NONE',  ( 0.000000000000000000, 1.000000000000000000, 0.000000000000000000 ) ) ;
#53675=CARTESIAN_POINT ( 'NONE',  ( 0.000000000000000000, 117.4749999999999943, -103.1875000000000000 ) ) ;
#53680=EDGE_LOOP ( 'NONE', ( #18241, #14584, #4026, #45723 ) ) ;
#53692=CARTESIAN_POINT ( 'NONE',  ( 3.968749999999215294, 120.6499999999999915, 105.4788588808464027 ) ) ;
#53696=CARTESIAN_POINT ( 'NONE',  ( -87.70409100286360626, 71.53177522571070313, -96.71266027437734181 ) ) ;
#53723=EDGE_CURVE ( 'NONE', #15453, #65492, #33024, .T. ) ;
#53736=ORIENTED_EDGE ( 'NONE', *, *, #56985, .T. ) ;
#53738=CARTESIAN_POINT ( 'NONE',  ( 0.000000000000000000, 124.9679999999999893, 0.000000000000000000 ) ) ;
#53740=ORIENTED_EDGE ( 'NONE', *, *, #73261, .F. ) ;
#53743=CARTESIAN_POINT ( 'NONE',  ( 0.000000000000000000, 61.59999999999999432, 118.5560000000000116 ) ) ;
#53756=LINE ( 'NONE', #54647, #70428 ) ;
#53786=DIRECTION ( 'NONE',  ( 0.000000000000000000, 0.000000000000000000, 1.000000000000000000 ) ) ;
#53807=CARTESIAN_POINT ( 'NONE',  ( -7.205548786489490269E-13, 117.4749999999999943, 103.1875000000000000 ) ) ;
#53808=CARTESIAN_POINT ( 'NONE',  ( -68.53801554307339927, 120.6499999999999915, -74.15067561874339219 ) ) ;
#53878=CARTESIAN_POINT ( 'NONE',  ( 33.98325472291465132, 124.5870000000000033, 3.174999999999999822 ) ) ;
#53901=CARTESIAN_POINT ( 'NONE',  ( 3.968750000000050182, 120.6499999999999915, -100.8961411191535973 ) ) ;
#53903=CYLINDRICAL_SURFACE ( 'NONE', #68765, 5.041900000000001825 ) ;
#53906=CARTESIAN_POINT ( 'NONE',  ( 118.5538584119706798, 95.23005795263746620, 0.8256312046399985061 ) ) ;
#53907=DIRECTION ( 'NONE',  ( 0.000000000000000000, 1.000000000000000000, 0.000000000000000000 ) ) ;
#53940=CARTESIAN_POINT ( 'NONE',  ( -117.9438495704237795, 78.46643079253874475, 12.03279974799046848 ) ) ;
#53947=CARTESIAN_POINT ( 'NONE',  ( 11.39816346244706580, 76.93354734096725167, -118.0069729841872146 ) ) ;
#53981=DIRECTION ( 'NONE',  ( 0.000000000000000000, 0.000000000000000000, 1.000000000000000000 ) ) ;
#53982=CARTESIAN_POINT ( 'NONE',  ( -130.5150051272322571, 94.82199753261677699, 3.295598630356760150 ) ) ;
#53983=CARTESIAN_POINT ( 'NONE',  ( -3.968750000000770051, 120.6499999999999915, 105.4788588808462038 ) ) ;
#53994=CARTESIAN_POINT ( 'NONE',  ( 82.96293804092860569, 84.21449860606320215, -100.8069756963038657 ) ) ;
#53999=CARTESIAN_POINT ( 'NONE',  ( -12.61759658107631665, 80.88542946572127335, -117.8827710199055048 ) ) ;
#54001=B_SPLINE_CURVE_WITH_KNOTS ( 'NONE', 3,
 ( #83308, #35133, #41056, #62844, #621, #6389, #47256, #74985, #40006, #61340, #26386, #19568, #47704, #19125, #40458, #89068, #82270, #53612, #54507, #67721, #12769, #87717, #26826, #11870, #46804, #74537, #27278, #32289, #34079, #66820, #59987, #25943, #82720, #20028, #75885, #40900, #68625, #5507, #20481, #61783, #33202, #5961, #60903, #88631, #48151, #89522, #25486, #5048, #53158 ),
 .UNSPECIFIED., .F., .F.,
 ( 4, 2, 2, 2, 2, 2, 2, 2, 2, 2, 2, 2, 2, 2, 2, 1, 2, 2, 2, 2, 2, 2, 2, 2, 4 ),
 ( 0.01986933033599076401, 0.02111088875730814801, 0.02235244717862552855, 0.02483556402126029655, 0.02607712244257766321, 0.02731868086389502639, 0.02980179770652975624, 0.03228491454916448261, 0.03352647297048184927, 0.03476803139179920898, 0.03725114823443395617, 0.03849270665575132977, 0.03973426507706870336, 0.04221738191970343668, 0.04345894034102081721, 0.04470049876233818387, 0.04594205718365555746, 0.04718361560497292412, 0.04966673244760769212, 0.05090829086892509348, 0.05214984929024249483, 0.05463296613287729753, 0.05587452455419468500, 0.05711608297551208635, 0.05959919981814688905 ),
 .UNSPECIFIED. ) ;
#54006=ORIENTED_EDGE ( 'NONE', *, *, #26762, .F. ) ;
#54010=LINE ( 'NONE', #19520, #23910 ) ;
#54014=ORIENTED_EDGE ( 'NONE', *, *, #80119, .T. ) ;
#54017=VECTOR ( 'NONE', #9967, 1000.000000000000114 ) ;
#54023=ORIENTED_EDGE ( 'NONE', *, *, #84999, .T. ) ;
#54039=ORIENTED_EDGE ( 'NONE', *, *, #63736, .F. ) ;
#54059=SURFACE_STYLE_FILL_AREA ( #32747 ) ;
#54062=ORIENTED_EDGE ( 'NONE', *, *, #7251, .F. ) ;
#54070=CARTESIAN_POINT ( 'NONE',  ( -11.89174298505462524, 78.07232539501590907, -130.0133884065672589 ) ) ;
#54071=EDGE_CURVE ( 'NONE', #43245, #65614, #62782, .T. ) ;
#54080=CARTESIAN_POINT ( 'NONE',  ( -91.90737012895647240, 78.46643079253875896, -74.89042153202906604 ) ) ;
#54081=EDGE_CURVE ( 'NONE', #6564, #52316, #49753, .T. ) ;
#54084=ORIENTED_EDGE ( 'NONE', *, *, #31297, .T. ) ;
#54126=VERTEX_POINT ( 'NONE', #43411 ) ;
#54145=CARTESIAN_POINT ( 'NONE',  ( -72.96458098368751166, 117.4749999999999943, 72.96458098368620426 ) ) ;
#54150=ADVANCED_FACE ( 'NONE', ( #9359 ), #86118, .F. ) ;
#54162=ORIENTED_EDGE ( 'NONE', *, *, #5297, .F. ) ;
#54169=CARTESIAN_POINT ( 'NONE',  ( 7.752335291937837880, 92.64399975678504973, 118.3043120271755413 ) ) ;
#54240=CARTESIAN_POINT ( 'NONE',  ( 7.736432051520609754, 72.46968852267782779, -130.3269799747974957 ) ) ;
#54242=CARTESIAN_POINT ( 'NONE',  ( 84.42134122279030350, 95.24969287062864964, 83.24211534968756609 ) ) ;
#54253=AXIS2_PLACEMENT_3D ( 'NONE', #9387, #79339, #18766 ) ;
#54258=ORIENTED_EDGE ( 'NONE', *, *, #69796, .T. ) ;
#54259=ORIENTED_EDGE ( 'NONE', *, *, #39048, .T. ) ;
#54270=ADVANCED_FACE ( 'NONE', ( #25656 ), #73811, .F. ) ;
#54274=ORIENTED_EDGE ( 'NONE', *, *, #89818, .T. ) ;
#54279=ORIENTED_EDGE ( 'NONE', *, *, #70938, .F. ) ;
#54291=ORIENTED_EDGE ( 'NONE', *, *, #68598, .F. ) ;
#54310=DIRECTION ( 'NONE',  ( 0.000000000000000000, -1.000000000000000000, 0.000000000000000000 ) ) ;
#54327=AXIS2_PLACEMENT_3D ( 'NONE', #23667, #51329, #38168 ) ;
#54330=ORIENTED_EDGE ( 'NONE', *, *, #21220, .T. ) ;
#54347=DIRECTION ( 'NONE',  ( 0.000000000000000000, 1.000000000000000000, 0.000000000000000000 ) ) ;
#54358=AXIS2_PLACEMENT_3D ( 'NONE', #59702, #80629, #73344 ) ;
#54367=VERTEX_POINT ( 'NONE', #20646 ) ;
#54379=CIRCLE ( 'NONE', #22544, 38.10000000000000142 ) ;
#54426=CARTESIAN_POINT ( 'NONE',  ( -130.3273610158207134, 92.64237678566782108, 7.754451942557587074 ) ) ;
#54438=CARTESIAN_POINT ( 'NONE',  ( 98.83759631548541336, 90.93932679091000182, -85.30153658290333851 ) ) ;
#54445=CIRCLE ( 'NONE', #12399, 7.937500000000000000 ) ;
#54459=DIRECTION ( 'NONE',  ( 1.000000000000000000, 0.000000000000000000, 1.047444401652940007E-14 ) ) ;
#54469=CARTESIAN_POINT ( 'NONE',  ( -118.5559670995752697, 95.24969287062862122, 0.8338386114225508905 ) ) ;
#54480=EDGE_CURVE ( 'NONE', #50419, #37237, #63771, .T. ) ;
#54485=CARTESIAN_POINT ( 'NONE',  ( -7.195828152521259823E-13, 127.0000000000000000, 95.25000000000000000 ) ) ;
#54498=CARTESIAN_POINT ( 'NONE',  ( -72.96458098368600531, 127.0000000000000000, -72.96458098368781009 ) ) ;
#54507=CARTESIAN_POINT ( 'NONE',  ( 130.4513346304067340, 94.12569442554139698, 5.240856348473897697 ) ) ;
#54526=CARTESIAN_POINT ( 'NONE',  ( -75.85240403722346514, 75.84278307195158675, -91.11526841082596206 ) ) ;
#54538=AXIS2_PLACEMENT_3D ( 'NONE', #4543, #10464, #67203 ) ;
#54547=CARTESIAN_POINT ( 'NONE',  ( 3.306873253463332496, 70.28105300984509540, 118.5105382607468130 ) ) ;
#54551=DIRECTION ( 'NONE',  ( 0.000000000000000000, -1.000000000000000000, 0.000000000000000000 ) ) ;
#54562=DIRECTION ( 'NONE',  ( 1.000000000000000000, 0.000000000000000000, 0.000000000000000000 ) ) ;
#54567=CARTESIAN_POINT ( 'NONE',  ( -97.40459591070860768, 72.22361908171434663, 86.93292302958646189 ) ) ;
#54581=LINE ( 'NONE', #60516, #85265 ) ;
#54583=DIRECTION ( 'NONE',  ( -0.8660254037844394848, 0.000000000000000000, 0.4999999999999985567 ) ) ;
#54588=ORIENTED_EDGE ( 'NONE', *, *, #35960, .F. ) ;
#54591=CARTESIAN_POINT ( 'NONE',  ( -94.33976020835963539, 70.17656663518266669, -90.24991642302057926 ) ) ;
#54604=CARTESIAN_POINT ( 'NONE',  ( -72.96458098368751166, 101.5999999999999943, 72.96458098368620426 ) ) ;
#54611=ADVANCED_FACE ( 'NONE', ( #16956 ), #85124, .F. ) ;
#54614=ORIENTED_EDGE ( 'NONE', *, *, #30631, .F. ) ;
#54617=CARTESIAN_POINT ( 'NONE',  ( 2.883928177975687124, 94.92528396209716846, 118.5216277020858229 ) ) ;
#54641=DIRECTION ( 'NONE',  ( 0.000000000000000000, 1.000000000000000000, 0.000000000000000000 ) ) ;
#54646=CARTESIAN_POINT ( 'NONE',  ( 10.09762896578686941, 90.29673011329585108, -118.1261022283270705 ) ) ;
#54647=CARTESIAN_POINT ( 'NONE',  ( 3.968750000000050182, 127.0000000000000000, -100.8961411191535973 ) ) ;
#54650=CARTESIAN_POINT ( 'NONE',  ( -8.391666350164323163, 92.11848141222131403, -118.2600956121756610 ) ) ;
#54707=VECTOR ( 'NONE', #71297, 1000.000000000000000 ) ;
#54712=VERTEX_POINT ( 'NONE', #73237 ) ;
#54722=ADVANCED_FACE ( 'NONE', ( #66424 ), #39612, .F. ) ;
#54727=ORIENTED_EDGE ( 'NONE', *, *, #65756, .F. ) ;
#54728=AXIS2_PLACEMENT_3D ( 'NONE', #70656, #48377, #27960 ) ;
#54729=DIRECTION ( 'NONE',  ( 1.000000000000000000, 0.000000000000000000, 8.465970413060558704E-17 ) ) ;
#54740=CARTESIAN_POINT ( 'NONE',  ( -130.0134586223093436, 78.07027470200928576, 11.89097723361267178 ) ) ;
#54741=ORIENTED_EDGE ( 'NONE', *, *, #70243, .T. ) ;
#54745=ORIENTED_EDGE ( 'NONE', *, *, #77992, .F. ) ;
#54747=DIRECTION ( 'NONE',  ( -1.000000000000000000, 0.000000000000000000, 0.000000000000000000 ) ) ;
#54764=DIRECTION ( 'NONE',  ( -0.9659258262890663138, 0.000000000000000000, -0.2588190451025281225 ) ) ;
#54777=AXIS2_PLACEMENT_3D ( 'NONE', #31681, #85784, #23116 ) ;
#54785=EDGE_LOOP ( 'NONE', ( #63840, #89021, #55804, #70742 ) ) ;
#54803=CARTESIAN_POINT ( 'NONE',  ( 3.017284783739249916E-15, 125.7300000000000040, 24.63800000000000168 ) ) ;
#54806=LINE ( 'NONE', #34836, #5228 ) ;
#54809=CARTESIAN_POINT ( 'NONE',  ( 72.96458098368701428, 117.4749999999999943, -72.96458098368670164 ) ) ;
#54812=DIRECTION ( 'NONE',  ( 0.000000000000000000, 1.000000000000000000, 0.000000000000000000 ) ) ;
#54837=CARTESIAN_POINT ( 'NONE',  ( 71.77848634863140376, 120.6499999999999915, -77.39114642429929347 ) ) ;
#54845=EDGE_LOOP ( 'NONE', ( #673, #28999 ) ) ;
#54849=VECTOR ( 'NONE', #74282, 1000.000000000000000 ) ;
#54854=CARTESIAN_POINT ( 'NONE',  ( 105.4788588808462038, 120.6499999999999915, -3.968749999999580336 ) ) ;
#54860=DIRECTION ( 'NONE',  ( 0.000000000000000000, 0.000000000000000000, 1.000000000000000000 ) ) ;
#54875=CARTESIAN_POINT ( 'NONE',  ( 89.95878776288157042, 70.27756284692560484, 94.61736061587697577 ) ) ;
#54889=CARTESIAN_POINT ( 'NONE',  ( 96.20686424029936745, 93.94566094357729469, -88.25669247804565032 ) ) ;
#54917=LINE ( 'NONE', #48108, #71149 ) ;
#54920=CARTESIAN_POINT ( 'NONE',  ( 74.43377912862210621, 80.88465057165900873, -92.27764637677437065 ) ) ;
#54922=CARTESIAN_POINT ( 'NONE',  ( -67.92268098368749918, 117.4749999999999943, 72.96458098368620426 ) ) ;
#54924=ORIENTED_EDGE ( 'NONE', *, *, #23416, .F. ) ;
#54938=EDGE_LOOP ( 'NONE', ( #83541, #50590, #5777, #38544 ) ) ;
#54954=CARTESIAN_POINT ( 'NONE',  ( 76.20505178924339873, 127.0000000000000000, 76.20505178924419454 ) ) ;
#54955=ORIENTED_EDGE ( 'NONE', *, *, #16374, .F. ) ;
#54972=CARTESIAN_POINT ( 'NONE',  ( -78.43243611888087230, 72.22378176823139029, -88.90442867305952745 ) ) ;
#54984=CARTESIAN_POINT ( 'NONE',  ( 83.15068351451354545, 79.66695435136418268, -100.6520717229715842 ) ) ;
#54994=CARTESIAN_POINT ( 'NONE',  ( 6.720192613126054759, 71.76561204655834558, 118.3658933525135524 ) ) ;
#54999=CYLINDRICAL_SURFACE ( 'NONE', #7931, 25.39999999999999858 ) ;
#55005=EDGE_CURVE ( 'NONE', #79094, #35450, #35942, .T. ) ;
#55047=DIRECTION ( 'NONE',  ( -0.000000000000000000, 1.000000000000000000, -0.000000000000000000 ) ) ;
#55052=VECTOR ( 'NONE', #17143, 1000.000000000000000 ) ;
#55065=LINE ( 'NONE', #48256, #70590 ) ;
#55110=DIRECTION ( 'NONE',  ( 0.000000000000000000, 0.000000000000000000, 1.000000000000000000 ) ) ;
#55112=CARTESIAN_POINT ( 'NONE',  ( -105.4788588808464027, 127.0000000000000000, 3.968749999998844924 ) ) ;
#55145=EDGE_LOOP ( 'NONE', ( #38077, #85561, #58051, #10141, #57162, #73069 ) ) ;
#55148=CARTESIAN_POINT ( 'NONE',  ( -82.91466710319176059, 83.38002811471483255, -100.8465607796068184 ) ) ;
#55164=B_SPLINE_CURVE_WITH_KNOTS ( 'NONE', 3,
 ( #89244, #80201, #59718, #87451, #18391, #81104, #46534, #39726, #5225, #32915, #60614, #48313, #76046, #62858, #75615, #63775, #82442, #35601, #83776, #634, #27896, #63318, #56488, #34711, #76951, #1094, #42849, #41071, #56027, #20204, #14735, #28333, #61960, #13825, #14282, #42406, #22002, #47875, #21091, #41509, #6560, #70133, #13384, #68793, #7902, #34259, #89697, #28806 ),
 .UNSPECIFIED., .F., .F.,
 ( 4, 2, 2, 2, 2, 2, 2, 2, 2, 1, 2, 2, 2, 2, 2, 2, 2, 2, 2, 2, 2, 1, 2, 2, 4 ),
 ( 0.05960646776571128236, 0.06208927922045071740, 0.06333068494782043145, 0.06457209067519015244, 0.06705490212992962218, 0.06829630785729937092, 0.06953771358466910579, 0.07202052503940861716, 0.07326193076677835203, 0.07450333649414807302, 0.07574474222151779401, 0.07698614794888751500, 0.07946895940362699862, 0.08195177085836648223, 0.08319317658573623098, 0.08443458231310599360, 0.08691739376784550497, 0.08815879949521525372, 0.08940020522258501634, 0.09188301667732445832, 0.09312442240469415156, 0.09436582813206384479, 0.09560723385943353803, 0.09684863958680323126, 0.09933145104154257610 ),
 .UNSPECIFIED. ) ;
#55168=ORIENTED_EDGE ( 'NONE', *, *, #19166, .F. ) ;
#55186=CARTESIAN_POINT ( 'NONE',  ( 130.0575199856853885, 76.93632333215538210, 11.39952500586094253 ) ) ;
#55187=EDGE_CURVE ( 'NONE', #66271, #27158, #68912, .T. ) ;
#55212=AXIS2_PLACEMENT_3D ( 'NONE', #74722, #6573, #67004 ) ;
#55213=EDGE_CURVE ( 'NONE', #27806, #71309, #30917, .T. ) ;
#55219=PLANE ( 'NONE',  #27755 ) ;
#55234=ADVANCED_FACE ( 'NONE', ( #17299 ), #53903, .F. ) ;
#55248=EDGE_LOOP ( 'NONE', ( #49863, #63434, #75991, #9291 ) ) ;
#55274=VERTEX_POINT ( 'NONE', #51783 ) ;
#55278=CARTESIAN_POINT ( 'NONE',  ( -12.53573128184445373, 84.62794568765839642, 117.8914214560859790 ) ) ;
#55284=EDGE_LOOP ( 'NONE', ( #32679, #79470 ) ) ;
#55309=EDGE_CURVE ( 'NONE', #26574, #89290, #56151, .T. ) ;
#55328=DIRECTION ( 'NONE',  ( 1.000000000000000000, 0.000000000000000000, 0.000000000000000000 ) ) ;
#55332=LINE ( 'NONE', #68544, #6793 ) ;
#55335=VERTEX_POINT ( 'NONE', #1676 ) ;
#55371=CARTESIAN_POINT ( 'NONE',  ( -72.96458098368751166, 127.0000000000000000, 72.96458098368620426 ) ) ;
#55388=CARTESIAN_POINT ( 'NONE',  ( 76.20774946062907418, 89.94786999841842601, -90.81826664111991931 ) ) ;
#55408=CARTESIAN_POINT ( 'NONE',  ( -72.96458098368751166, 127.0000000000000000, 65.02708098368620426 ) ) ;
#55448=CARTESIAN_POINT ( 'NONE',  ( 4.101352651117800896, 70.52330563318118095, 118.4857037620892726 ) ) ;
#55468=CARTESIAN_POINT ( 'NONE',  ( -95.43663006862796294, 70.66229531820913223, 89.08909376920047407 ) ) ;
#55477=DIRECTION ( 'NONE',  ( 0.000000000000000000, 1.000000000000000000, 0.000000000000000000 ) ) ;
#55488=CARTESIAN_POINT ( 'NONE',  ( -92.12450916458696781, 85.43299024555682308, -74.62309654709174822 ) ) ;
#55512=CARTESIAN_POINT ( 'NONE',  ( 10.08084112162954682, 90.28574336371693221, 118.1269349842563088 ) ) ;
#55515=LINE ( 'NONE', #575, #23692 ) ;
#55536=CARTESIAN_POINT ( 'NONE',  ( -105.4788588808462038, 120.6499999999999915, -3.968750000001139977 ) ) ;
#55541=CARTESIAN_POINT ( 'NONE',  ( 1.451892247740217613E-14, 95.25000000000000000, -118.5560000000000116 ) ) ;
#55552=DIRECTION ( 'NONE',  ( -0.8660254037844387076, 0.000000000000000000, -0.4999999999999998890 ) ) ;
#55586=CARTESIAN_POINT ( 'NONE',  ( 0.000000000000000000, 111.1250000000000000, 0.000000000000000000 ) ) ;
#55594=CARTESIAN_POINT ( 'NONE',  ( 12.69999999999999929, 81.71142461540233626, 129.9368274816650626 ) ) ;
#55607=ORIENTED_EDGE ( 'NONE', *, *, #5297, .T. ) ;
#55622=EDGE_CURVE ( 'NONE', #33210, #5885, #88426, .T. ) ;
#55632=CARTESIAN_POINT ( 'NONE',  ( 4.163101094985349692E-14, 120.6499999999999915, -107.7702177616926065 ) ) ;
#55634=CARTESIAN_POINT ( 'NONE',  ( 130.4354319819074419, 71.15434825076366110, -5.621545387652600922 ) ) ;
#55661=PLANE ( 'NONE',  #59100 ) ;
#55665=FACE_OUTER_BOUND ( 'NONE', #20420, .T. ) ;
#55671=ORIENTED_EDGE ( 'NONE', *, *, #21948, .T. ) ;
#55688=AXIS2_PLACEMENT_3D ( 'NONE', #76578, #68863, #41581 ) ;
#55690=CARTESIAN_POINT ( 'NONE',  ( 92.02731164704593425, 95.25015599858943460, 92.60677566276864070 ) ) ;
#55697=PLANE ( 'NONE',  #69014 ) ;
#55713=ORIENTED_EDGE ( 'NONE', *, *, #12679, .F. ) ;
#55717=CARTESIAN_POINT ( 'NONE',  ( -5.624880194777449383, 93.94404932077412695, 118.4230601929072435 ) ) ;
#55732=CARTESIAN_POINT ( 'NONE',  ( 4.085245964383497075, 70.51776014978250373, -118.4862668242151358 ) ) ;
#55733=CARTESIAN_POINT ( 'NONE',  ( 72.96458098368650269, 127.0000000000000000, 80.90208098368729850 ) ) ;
#55760=DIRECTION ( 'NONE',  ( 0.000000000000000000, 0.000000000000000000, -1.000000000000000000 ) ) ;
#55804=ORIENTED_EDGE ( 'NONE', *, *, #50166, .F. ) ;
#55805=CARTESIAN_POINT ( 'NONE',  ( -88.20661029664569242, 93.55239623846826191, 79.21650378603861498 ) ) ;
#55812=CARTESIAN_POINT ( 'NONE',  ( -118.5215310810514495, 94.92435932957491218, 2.887881501069120116 ) ) ;
#55816=CARTESIAN_POINT ( 'NONE',  ( 76.80536679343914841, 74.16967745525862199, -90.31351860656764075 ) ) ;
#55838=EDGE_LOOP ( 'NONE', ( #56298, #67106, #77873, #698 ) ) ;
#55854=ORIENTED_EDGE ( 'NONE', *, *, #78527, .T. ) ;
#55858=VERTEX_POINT ( 'NONE', #73324 ) ;
#55862=CARTESIAN_POINT ( 'NONE',  ( -3.968750000000754508, 120.6499999999999915, 100.8961411191535973 ) ) ;
#55872=DIRECTION ( 'NONE',  ( 0.000000000000000000, -1.000000000000000000, 0.000000000000000000 ) ) ;
#55883=AXIS2_PLACEMENT_3D ( 'NONE', #26889, #40960, #54562 ) ;
#55895=CARTESIAN_POINT ( 'NONE',  ( -129.9368274816650626, 82.54999999999999716, -12.70000000000045404 ) ) ;
#55900=FACE_OUTER_BOUND ( 'NONE', #52573, .T. ) ;
#55901=CIRCLE ( 'NONE', #44308, 118.5560000000000116 ) ;
#55919=CARTESIAN_POINT ( 'NONE',  ( -99.18073718829342056, 74.80151635532867260, 84.90151352399695384 ) ) ;
#55920=B_SPLINE_CURVE_WITH_KNOTS ( 'NONE', 3,
 ( #82017, #27473, #55148, #40193, #46996, #89268, #74734, #12964, #53359, #74289, #67914, #41093, #18872, #41532, #34735, #88380, #13850, #33395, #46557, #5703, #61096, #61984, #75639, #40653, #6151, #82468, #20225, #76070, #89723, #39749, #47896, #48337, #69262, #1118, #657, #84255, #14307, #41983, #29276, #22029, #49699, #84703, #64242, #85149, #71071, #77421, #35170, #28363, #8386 ),
 .UNSPECIFIED., .F., .F.,
 ( 4, 2, 2, 2, 2, 2, 2, 2, 2, 2, 2, 2, 2, 2, 2, 1, 2, 2, 2, 2, 2, 2, 2, 2, 4 ),
 ( 0.01986933033599077442, 0.02111088875730818271, 0.02235244717862559100, 0.02483556402126041451, 0.02607712244257780546, 0.02731868086389519640, 0.02980179770652996440, 0.03228491454916473241, 0.03352647297048211295, 0.03476803139179950042, 0.03725114823443430312, 0.03849270665575170447, 0.03973426507706910582, 0.04221738191970388077, 0.04345894034102125436, 0.04470049876233862796, 0.04594205718365600155, 0.04718361560497337515, 0.04966673244760812234, 0.05090829086892548205, 0.05214984929024284871, 0.05463296613287755427, 0.05587452455419490011, 0.05711608297551223901, 0.05959919981814693069 ),
 .UNSPECIFIED. ) ;
#55935=LINE ( 'NONE', #105, #67646 ) ;
#55938=ORIENTED_EDGE ( 'NONE', *, *, #45132, .F. ) ;
#55941=CARTESIAN_POINT ( 'NONE',  ( -83.22961976134699569, 79.25971567868506895, -100.5868491334645825 ) ) ;
#55942=CARTESIAN_POINT ( 'NONE',  ( -92.06080542007461531, 85.83559868056556752, -74.70172715947531117 ) ) ;
#55976=CYLINDRICAL_SURFACE ( 'NONE', #64208, 12.70000000000000107 ) ;
#55991=DIRECTION ( 'NONE',  ( 0.000000000000000000, 1.000000000000000000, 0.000000000000000000 ) ) ;
#55992=DIRECTION ( 'NONE',  ( 0.9659258262890693114, 0.000000000000000000, 0.2588190451025170757 ) ) ;
#55996=CARTESIAN_POINT ( 'NONE',  ( -3.298961202091059697, 94.84210650921832553, 130.5168528568578097 ) ) ;
#56008=DIRECTION ( 'NONE',  ( 0.000000000000000000, 1.000000000000000000, 0.000000000000000000 ) ) ;
#56020=ORIENTED_EDGE ( 'NONE', *, *, #30619, .T. ) ;
#56027=CARTESIAN_POINT ( 'NONE',  ( -86.67600044576296625, 70.52018178143200089, 80.88853703239344384 ) ) ;
#56029=CARTESIAN_POINT ( 'NONE',  ( -76.20505178924278766, 127.0000000000000000, -76.20505178924469192 ) ) ;
#56051=CARTESIAN_POINT ( 'NONE',  ( 12.27515439545620701, 79.26608163778621474, 129.9777074703579842 ) ) ;
#56054=DIRECTION ( 'NONE',  ( 0.000000000000000000, -1.000000000000000000, 0.000000000000000000 ) ) ;
#56061=ORIENTED_EDGE ( 'NONE', *, *, #65783, .F. ) ;
#56063=DIRECTION ( 'NONE',  ( 0.4999999999999998890, 0.000000000000000000, -0.8660254037844387076 ) ) ;
#56079=ORIENTED_EDGE ( 'NONE', *, *, #63491, .F. ) ;
#56087=DIRECTION ( 'NONE',  ( 0.000000000000000000, 1.000000000000000000, 0.000000000000000000 ) ) ;
#56107=ORIENTED_EDGE ( 'NONE', *, *, #87529, .T. ) ;
#56127=ORIENTED_EDGE ( 'NONE', *, *, #36493, .F. ) ;
#56151=LINE ( 'NONE', #35723, #29597 ) ;
#56152=CARTESIAN_POINT ( 'NONE',  ( 91.13664476550619042, 95.14808745951974345, 93.48344774443376082 ) ) ;
#56154=ADVANCED_FACE ( 'NONE', ( #26082 ), #33783, .F. ) ;
#56167=CONICAL_SURFACE ( 'NONE', #80850, 188.9759999999999991, 0.7853981633974758125 ) ;
#56230=ORIENTED_EDGE ( 'NONE', *, *, #68472, .T. ) ;
#56239=DIRECTION ( 'NONE',  ( 0.000000000000000000, -1.000000000000000000, 0.000000000000000000 ) ) ;
#56252=EDGE_CURVE ( 'NONE', #26653, #32576, #12907, .T. ) ;
#56264=CARTESIAN_POINT ( 'NONE',  ( -78.95047879920342382, 93.33860577356860233, 88.44471653959794821 ) ) ;
#56268=CIRCLE ( 'NONE', #8464, 188.9759999999999991 ) ;
#56269=CARTESIAN_POINT ( 'NONE',  ( -117.9583070260532764, 87.03046781249437913, 11.89069406032439247 ) ) ;
#56275=CARTESIAN_POINT ( 'NONE',  ( 3.174999999999879918, 104.3431970271541900, 33.98325472291465132 ) ) ;
#56290=CARTESIAN_POINT ( 'NONE',  ( 84.12159398442716451, 95.25015226514366873, -83.54193218351822736 ) ) ;
#56298=ORIENTED_EDGE ( 'NONE', *, *, #19109, .F. ) ;
#56318=CARTESIAN_POINT ( 'NONE',  ( -6.359898342742077659, 71.54935466043629333, -130.4015153071888733 ) ) ;
#56329=CARTESIAN_POINT ( 'NONE',  ( -80.59807192910929530, 70.66242608954388515, -86.94609723791364786 ) ) ;
#56335=ORIENTED_EDGE ( 'NONE', *, *, #34811, .T. ) ;
#56377=EDGE_CURVE ( 'NONE', #58908, #80081, #83291, .T. ) ;
#56378=FACE_OUTER_BOUND ( 'NONE', #13320, .T. ) ;
#56384=AXIS2_PLACEMENT_3D ( 'NONE', #53675, #4666, #47317 ) ;
#56413=PLANE ( 'NONE',  #29555 ) ;
#56445=DIRECTION ( 'NONE',  ( 0.000000000000000000, 1.000000000000000000, 0.000000000000000000 ) ) ;
#56449=DIRECTION ( 'NONE',  ( 0.000000000000000000, 1.000000000000000000, 0.000000000000000000 ) ) ;
#56462=VECTOR ( 'NONE', #3633, 1000.000000000000000 ) ;
#56481=EDGE_LOOP ( 'NONE', ( #84713, #50238, #39297, #12601 ) ) ;
#56488=CARTESIAN_POINT ( 'NONE',  ( -82.65143893653566920, 69.93120980984942037, 84.99964240976949270 ) ) ;
#56491=EDGE_CURVE ( 'NONE', #83766, #59751, #80057, .T. ) ;
#56494=ORIENTED_EDGE ( 'NONE', *, *, #82123, .T. ) ;
#56511=CARTESIAN_POINT ( 'NONE',  ( 12.37565694608801437, 79.66829940370548968, 129.9681453810340770 ) ) ;
#56517=EDGE_CURVE ( 'NONE', #41269, #11232, #36926, .T. ) ;
#56527=CARTESIAN_POINT ( 'NONE',  ( 72.96458098368701428, 127.0000000000000000, -65.82083098368670449 ) ) ;
#56536=CIRCLE ( 'NONE', #78298, 7.143749999999999822 ) ;
#56542=EDGE_CURVE ( 'NONE', #12790, #55335, #11903, .T. ) ;
#56554=VERTEX_POINT ( 'NONE', #46837 ) ;
#56568=CARTESIAN_POINT ( 'NONE',  ( 0.000000000000000000, 124.5870000000000033, 0.000000000000000000 ) ) ;
#56614=CARTESIAN_POINT ( 'NONE',  ( 83.76986456925334323, 87.79544278253753475, 100.1374281256150169 ) ) ;
#56617=DIRECTION ( 'NONE',  ( 0.000000000000000000, -1.000000000000000000, 0.000000000000000000 ) ) ;
#56623=VECTOR ( 'NONE', #59677, 1000.000000000000000 ) ;
#56627=FACE_OUTER_BOUND ( 'NONE', #20210, .T. ) ;
#56636=CARTESIAN_POINT ( 'NONE',  ( -12.67976775996874572, 83.37995484863287743, 117.8759955821573158 ) ) ;
#56693=ORIENTED_EDGE ( 'NONE', *, *, #13872, .F. ) ;
#56717=CYLINDRICAL_SURFACE ( 'NONE', #19729, 12.70000000000000462 ) ;
#56725=CARTESIAN_POINT ( 'NONE',  ( -91.24829632406202506, 88.91144712388911842, 75.69222284415488389 ) ) ;
#56734=CARTESIAN_POINT ( 'NONE',  ( 85.85219768521609751, 70.17671898886894155, -81.76240029069555248 ) ) ;
#56743=EDGE_CURVE ( 'NONE', #9318, #32614, #68505, .T. ) ;
#56751=CARTESIAN_POINT ( 'NONE',  ( 84.99753727674156778, 95.14807216649714405, -82.65057572782293960 ) ) ;
#56753=LINE ( 'NONE', #21351, #61784 ) ;
#56760=DIRECTION ( 'NONE',  ( 0.000000000000000000, 0.000000000000000000, -1.000000000000000000 ) ) ;
#56801=DIRECTION ( 'NONE',  ( -0.000000000000000000, 1.000000000000000000, -0.000000000000000000 ) ) ;
#56807=DIRECTION ( 'NONE',  ( -0.7071067811865460184, 0.000000000000000000, 0.7071067811865489050 ) ) ;
#56822=DIRECTION ( 'NONE',  ( -1.000000000000000000, 0.000000000000000000, 1.046082768126375896E-16 ) ) ;
#56834=FACE_OUTER_BOUND ( 'NONE', #16108, .T. ) ;
#56839=CARTESIAN_POINT ( 'NONE',  ( -72.96458098368600531, 101.5999999999999943, -72.96458098368781009 ) ) ;
#56849=CARTESIAN_POINT ( 'NONE',  ( -91.51255889651575615, 88.18374315479977099, -75.37293521528332008 ) ) ;
#56856=ORIENTED_EDGE ( 'NONE', *, *, #38915, .F. ) ;
#56859=CARTESIAN_POINT ( 'NONE',  ( 0.000000000000000000, 101.5999999999999943, 118.5560000000000116 ) ) ;
#56912=CARTESIAN_POINT ( 'NONE',  ( -0.4144590284063416896, 95.25000000000001421, 130.5560000000000400 ) ) ;
#56922=PLANE ( 'NONE',  #81269 ) ;
#56958=ORIENTED_EDGE ( 'NONE', *, *, #19225, .F. ) ;
#56964=CARTESIAN_POINT ( 'NONE',  ( 77.39114642429899504, 120.6499999999999915, 71.77848634863160271 ) ) ;
#56975=CARTESIAN_POINT ( 'NONE',  ( 71.77848634863079269, 120.6499999999999915, 77.39114642429989033 ) ) ;
#56979=DIRECTION ( 'NONE',  ( -1.000000000000000000, 0.000000000000000000, 1.046082768126375896E-16 ) ) ;
#56985=EDGE_CURVE ( 'NONE', #27806, #43612, #89794, .T. ) ;
#56997=FACE_OUTER_BOUND ( 'NONE', #41058, .T. ) ;
#57000=ORIENTED_EDGE ( 'NONE', *, *, #10253, .F. ) ;
#57002=ORIENTED_EDGE ( 'NONE', *, *, #41664, .T. ) ;
#57023=VERTEX_POINT ( 'NONE', #21190 ) ;
#57036=EDGE_CURVE ( 'NONE', #9719, #20160, #67534, .T. ) ;
#57057=CARTESIAN_POINT ( 'NONE',  ( 100.4326241145864032, 86.63355734047006251, 83.41565754067561045 ) ) ;
#57101=ORIENTED_EDGE ( 'NONE', *, *, #66652, .T. ) ;
#57105=FACE_OUTER_BOUND ( 'NONE', #59444, .T. ) ;
#57116=CARTESIAN_POINT ( 'NONE',  ( -72.96458098368751166, 127.0000000000000000, 78.00648098368618832 ) ) ;
#57122=CYLINDRICAL_SURFACE ( 'NONE', #44818, 5.041900000000001825 ) ;
#57137=ORIENTED_EDGE ( 'NONE', *, *, #84722, .F. ) ;
#57162=ORIENTED_EDGE ( 'NONE', *, *, #53651, .F. ) ;
#57163=FACE_OUTER_BOUND ( 'NONE', #32944, .T. ) ;
#57168=CARTESIAN_POINT ( 'NONE',  ( -91.91945768840186304, 86.64222086580515736, 74.87617104506270493 ) ) ;
#57200=CIRCLE ( 'NONE', #20967, 7.143749999999999822 ) ;
#57201=VERTEX_POINT ( 'NONE', #87434 ) ;
#57229=EDGE_LOOP ( 'NONE', ( #6866, #78778 ) ) ;
#57296=CARTESIAN_POINT ( 'NONE',  ( -86.67541640318120244, 94.58006533271586136, -80.88915705228883724 ) ) ;
#57320=DIRECTION ( 'NONE',  ( 0.000000000000000000, 0.7071067811865600072, 0.7071067811865350272 ) ) ;
#57336=DIRECTION ( 'NONE',  ( -0.2588190451025219607, 0.000000000000000000, -0.9659258262890678681 ) ) ;
#57382=DIRECTION ( 'NONE',  ( 0.000000000000000000, 1.000000000000000000, 0.000000000000000000 ) ) ;
#57416=VECTOR ( 'NONE', #6336, 1000.000000000000114 ) ;
#57419=AXIS2_PLACEMENT_3D ( 'NONE', #64097, #36830, #85455 ) ;
#57428=DIRECTION ( 'NONE',  ( 0.000000000000000000, 1.000000000000000000, 0.000000000000000000 ) ) ;
#57440=EDGE_CURVE ( 'NONE', #80299, #13859, #60246, .T. ) ;
#57446=DIRECTION ( 'NONE',  ( 0.000000000000000000, 0.000000000000000000, 1.000000000000000000 ) ) ;
#57449=CARTESIAN_POINT ( 'NONE',  ( -130.3463096697863079, 72.22361908171431821, -7.404590904609003488 ) ) ;
#57457=EDGE_LOOP ( 'NONE', ( #1034, #66739, #16452, #75530 ) ) ;
#57490=CARTESIAN_POINT ( 'NONE',  ( -71.77848634863190114, 120.6499999999999915, 77.39114642429879609 ) ) ;
#57513=CARTESIAN_POINT ( 'NONE',  ( 83.21537498883908768, 85.85000629251467785, 100.5986936721449467 ) ) ;
#57519=EDGE_CURVE ( 'NONE', #8309, #23727, #34179, .T. ) ;
#57557=FACE_OUTER_BOUND ( 'NONE', #17280, .T. ) ;
#57564=CARTESIAN_POINT ( 'NONE',  ( -98.60478223830740774, 120.6499999999999915, -1.074461880482445986E-12 ) ) ;
#57576=ADVANCED_FACE ( 'NONE', ( #80512 ), #65531, .T. ) ;
#57583=AXIS2_PLACEMENT_3D ( 'NONE', #30237, #16606, #22535 ) ;
#57587=CARTESIAN_POINT ( 'NONE',  ( 84.90151352399593065, 74.80151635532864418, 99.18073718829431584 ) ) ;
#57588=DIRECTION ( 'NONE',  ( 0.000000000000000000, 1.000000000000000000, 0.000000000000000000 ) ) ;
#57596=ADVANCED_FACE ( 'NONE', ( #57822 ), #10775, .T. ) ;
#57599=DIRECTION ( 'NONE',  ( -0.000000000000000000, 1.000000000000000000, 0.000000000000000000 ) ) ;
#57606=CARTESIAN_POINT ( 'NONE',  ( 81.76240029069523985, 70.17671898886891313, 85.85219768521638173 ) ) ;
#57625=CARTESIAN_POINT ( 'NONE',  ( -74.36911441044730964, 82.54999999999999716, 92.32962665258534685 ) ) ;
#57672=DIRECTION ( 'NONE',  ( 0.000000000000000000, 0.000000000000000000, 1.000000000000000000 ) ) ;
#57692=CARTESIAN_POINT ( 'NONE',  ( 0.000000000000000000, 111.1250000000000000, 42.54500000000000171 ) ) ;
#57697=ORIENTED_EDGE ( 'NONE', *, *, #26734, .T. ) ;
#57717=VECTOR ( 'NONE', #45297, 1000.000000000000000 ) ;
#57736=ADVANCED_FACE ( 'NONE', ( #25987 ), #54999, .T. ) ;
#57739=PLANE ( 'NONE',  #74846 ) ;
#57755=DIRECTION ( 'NONE',  ( 0.000000000000000000, 1.000000000000000000, 0.000000000000000000 ) ) ;
#57775=VERTEX_POINT ( 'NONE', #33248 ) ;
#57789=CARTESIAN_POINT ( 'NONE',  ( -7.736432051520609754, 72.46968852267782779, 130.3269799747974957 ) ) ;
#57794=ORIENTED_EDGE ( 'NONE', *, *, #65981, .T. ) ;
#57810=EDGE_CURVE ( 'NONE', #43486, #16565, #75032, .T. ) ;
#57822=FACE_OUTER_BOUND ( 'NONE', #31619, .T. ) ;
#57829=CARTESIAN_POINT ( 'NONE',  ( -72.96458098368600531, 117.4749999999999943, -65.02708098368781009 ) ) ;
#57844=VECTOR ( 'NONE', #78196, 999.9999999999998863 ) ;
#57854=AXIS2_PLACEMENT_3D ( 'NONE', #61106, #6597, #27928 ) ;
#57875=AXIS2_PLACEMENT_3D ( 'NONE', #63155, #48162, #937 ) ;
#57907=ORIENTED_EDGE ( 'NONE', *, *, #39725, .T. ) ;
#57958=CARTESIAN_POINT ( 'NONE',  ( -97.46300000000000807, 82.54999999999999716, 12.69999999999966178 ) ) ;
#57960=FACE_OUTER_BOUND ( 'NONE', #85523, .T. ) ;
#57962=CARTESIAN_POINT ( 'NONE',  ( 74.36911441044605908, 82.96450994655477018, 92.32962665258638424 ) ) ;
#57967=DIRECTION ( 'NONE',  ( 0.000000000000000000, 0.000000000000000000, 1.000000000000000000 ) ) ;
#57970=VECTOR ( 'NONE', #48803, 1000.000000000000114 ) ;
#57971=EDGE_CURVE ( 'NONE', #46578, #6827, #33978, .T. ) ;
#57993=EDGE_CURVE ( 'NONE', #21337, #41991, #64101, .T. ) ;
#58004=CARTESIAN_POINT ( 'NONE',  ( 0.000000000000000000, 92.07499999999998863, 0.000000000000000000 ) ) ;
#58012=PLANE ( 'NONE',  #53163 ) ;
#58013=AXIS2_PLACEMENT_3D ( 'NONE', #54922, #27245, #82685 ) ;
#58014=EDGE_LOOP ( 'NONE', ( #55168, #28645, #25376, #40870 ) ) ;
#58024=DIRECTION ( 'NONE',  ( 1.000000000000000000, 0.000000000000000000, 0.000000000000000000 ) ) ;
#58026=ORIENTED_EDGE ( 'NONE', *, *, #57971, .F. ) ;
#58032=LINE ( 'NONE', #71677, #38650 ) ;
#58043=CARTESIAN_POINT ( 'NONE',  ( 83.15048135366386362, 79.66749569656609253, 100.6522392491107922 ) ) ;
#58051=ORIENTED_EDGE ( 'NONE', *, *, #15614, .F. ) ;
#58058=CARTESIAN_POINT ( 'NONE',  ( 74.36911441044604487, 81.72118090664555723, 92.32962665258637003 ) ) ;
#58074=CARTESIAN_POINT ( 'NONE',  ( 0.000000000000000000, 125.7300000000000040, 0.000000000000000000 ) ) ;
#58078=EDGE_CURVE ( 'NONE', #89290, #74189, #39816, .T. ) ;
#58095=DIRECTION ( 'NONE',  ( 0.000000000000000000, 1.000000000000000000, 0.000000000000000000 ) ) ;
#58101=ORIENTED_EDGE ( 'NONE', *, *, #13098, .T. ) ;
#58103=EDGE_LOOP ( 'NONE', ( #15942, #6320 ) ) ;
#58106=EDGE_LOOP ( 'NONE', ( #32023, #23518, #14014, #26633, #89906, #18975, #51924, #24664, #44312, #23015 ) ) ;
#58115=LINE ( 'NONE', #50852, #30147 ) ;
#58147=EDGE_CURVE ( 'NONE', #19337, #1704, #9423, .T. ) ;
#58155=CARTESIAN_POINT ( 'NONE',  ( 33.98325472291465132, 111.1250000000000000, -3.174999999999999822 ) ) ;
#58169=ORIENTED_EDGE ( 'NONE', *, *, #21401, .F. ) ;
#58177=DIRECTION ( 'NONE',  ( 0.000000000000000000, 0.000000000000000000, 1.000000000000000000 ) ) ;
#58187=LINE ( 'NONE', #50921, #71937 ) ;
#58209=CARTESIAN_POINT ( 'NONE',  ( -7.301849239715819957E-13, 120.6499999999999915, 98.60478223830740774 ) ) ;
#58239=CARTESIAN_POINT ( 'NONE',  ( -8.383129030752360933, 73.00074830044857777, 130.2869803084437592 ) ) ;
#58244=CARTESIAN_POINT ( 'NONE',  ( 76.20505178924339873, 127.0000000000000000, 76.20505178924419454 ) ) ;
#58268=DIRECTION ( 'NONE',  ( 0.000000000000000000, 0.000000000000000000, -1.000000000000000000 ) ) ;
#58300=CARTESIAN_POINT ( 'NONE',  ( 118.5560669097358470, 69.84937538953987257, -0.8299548590967218420 ) ) ;
#58303=EDGE_CURVE ( 'NONE', #11327, #35298, #66054, .T. ) ;
#58323=CARTESIAN_POINT ( 'NONE',  ( -4.085245964383497075, 70.51776014978250373, 118.4862668242151358 ) ) ;
#58345=CARTESIAN_POINT ( 'NONE',  ( -129.9368274816650626, 82.54999999999999716, -12.70000000000045404 ) ) ;
#58348=ORIENTED_EDGE ( 'NONE', *, *, #74697, .F. ) ;
#58354=DIRECTION ( 'NONE',  ( 0.000000000000000000, 0.000000000000000000, -1.000000000000000000 ) ) ;
#58366=FACE_OUTER_BOUND ( 'NONE', #53398, .T. ) ;
#58387=ORIENTED_EDGE ( 'NONE', *, *, #30619, .F. ) ;
#58405=CARTESIAN_POINT ( 'NONE',  ( 75.24778849303555717, 87.79588542099537563, 91.61507027739615694 ) ) ;
#58410=CARTESIAN_POINT ( 'NONE',  ( 6.349842397765909752, 93.55646220832403515, 130.4020064843513467 ) ) ;
#58418=ORIENTED_EDGE ( 'NONE', *, *, #50292, .T. ) ;
#58419=ORIENTED_EDGE ( 'NONE', *, *, #58147, .F. ) ;
#58420=ADVANCED_FACE ( 'NONE', ( #20416 ), #14948, .F. ) ;
#58442=CARTESIAN_POINT ( 'NONE',  ( 0.000000000000000000, 61.59999999999999432, 0.000000000000000000 ) ) ;
#58461=DIRECTION ( 'NONE',  ( 0.000000000000000000, 0.000000000000000000, -1.000000000000000000 ) ) ;
#58480=VERTEX_POINT ( 'NONE', #7675 ) ;
#58481=ORIENTED_EDGE ( 'NONE', *, *, #29183, .F. ) ;
#58488=DIRECTION ( 'NONE',  ( 3.386875084296745512E-15, 0.000000000000000000, -1.000000000000000000 ) ) ;
#58492=CARTESIAN_POINT ( 'NONE',  ( 75.85240403722289670, 75.84278307195161517, 91.11526841082653050 ) ) ;
#58504=CARTESIAN_POINT ( 'NONE',  ( 117.8738102209306362, 82.54999999999999716, 12.70000000000123386 ) ) ;
#58512=DIRECTION ( 'NONE',  ( 0.000000000000000000, 1.000000000000000000, 0.000000000000000000 ) ) ;
#58524=EDGE_CURVE ( 'NONE', #12394, #62096, #81220, .T. ) ;
#58543=CYLINDRICAL_SURFACE ( 'NONE', #39114, 5.041900000000000048 ) ;
#58562=CARTESIAN_POINT ( 'NONE',  ( -7.205548786489490269E-13, 101.5999999999999943, 103.1875000000000000 ) ) ;
#58574=CARTESIAN_POINT ( 'NONE',  ( 76.20505178924389611, 127.0000000000000000, -76.20505178924359768 ) ) ;
#58585=CARTESIAN_POINT ( 'NONE',  ( -100.8961411191535973, 120.6499999999999915, -3.968750000001104894 ) ) ;
#58609=EDGE_CURVE ( 'NONE', #40086, #63483, #39395, .T. ) ;
#58615=VECTOR ( 'NONE', #8957, 1000.000000000000000 ) ;
#58618=VECTOR ( 'NONE', #76661, 1000.000000000000000 ) ;
#58619=CARTESIAN_POINT ( 'NONE',  ( -91.13883569058442902, 95.16896684734908263, 93.48397507443846166 ) ) ;
#58666=VERTEX_POINT ( 'NONE', #74374 ) ;
#58687=FACE_OUTER_BOUND ( 'NONE', #26405, .T. ) ;
#58689=AXIS2_PLACEMENT_3D ( 'NONE', #67398, #6094, #47392 ) ;
#58715=EDGE_CURVE ( 'NONE', #82109, #58666, #64220, .T. ) ;
#58721=COLOUR_RGB ( '', 0.08235294, 0.09019608, 0.10196078) ;
#58729=CARTESIAN_POINT ( 'NONE',  ( 118.0068565116052497, 76.93600387762167259, 11.39936611905845076 ) ) ;
#58765=FACE_BOUND ( 'NONE', #50729, .T. ) ;
#58776=CARTESIAN_POINT ( 'NONE',  ( 3.174999999999889688, 124.5870000000000033, 31.75000000000000000 ) ) ;
#58794=LINE ( 'NONE', #10654, #7784 ) ;
#58797=CARTESIAN_POINT ( 'NONE',  ( -31.75000000000000000, 104.3431970271541900, 3.174999999999779998 ) ) ;
#58800=ORIENTED_EDGE ( 'NONE', *, *, #79136, .F. ) ;
#58814=AXIS2_PLACEMENT_3D ( 'NONE', #39520, #87238, #88585 ) ;
#58829=CARTESIAN_POINT ( 'NONE',  ( 105.4788588808462038, 127.0000000000000000, -3.968749999999580336 ) ) ;
#58852=VECTOR ( 'NONE', #27256, 1000.000000000000114 ) ;
#58876=DIRECTION ( 'NONE',  ( 0.000000000000000000, -1.000000000000000000, 0.000000000000000000 ) ) ;
#58877=LINE ( 'NONE', #80696, #45150 ) ;
#58892=AXIS2_PLACEMENT_3D ( 'NONE', #74927, #12706, #40393 ) ;
#58908=VERTEX_POINT ( 'NONE', #38724 ) ;
#58913=CARTESIAN_POINT ( 'NONE',  ( 82.96136257729986596, 80.89704698943971550, 100.8082743238010011 ) ) ;
#58928=CARTESIAN_POINT ( 'NONE',  ( 88.20503424218220800, 71.54629894495529641, 79.21825297796496557 ) ) ;
#58943=CARTESIAN_POINT ( 'NONE',  ( 118.5472366675172537, 95.16897323824359489, -1.658320819116884781 ) ) ;
#58978=ORIENTED_EDGE ( 'NONE', *, *, #87529, .F. ) ;
#58990=ORIENTED_EDGE ( 'NONE', *, *, #56542, .T. ) ;
#59002=PLANE ( 'NONE',  #60697 ) ;
#59021=FACE_OUTER_BOUND ( 'NONE', #72766, .T. ) ;
#59028=ORIENTED_EDGE ( 'NONE', *, *, #63567, .T. ) ;
#59050=CARTESIAN_POINT ( 'NONE',  ( 0.000000000000000000, 103.1240000000000236, 0.000000000000000000 ) ) ;
#59053=ORIENTED_EDGE ( 'NONE', *, *, #16668, .T. ) ;
#59058=VECTOR ( 'NONE', #79902, 1000.000000000000000 ) ;
#59060=CARTESIAN_POINT ( 'NONE',  ( -99.76704648669993958, 88.91113633199481114, 84.21071524772808914 ) ) ;
#59074=CARTESIAN_POINT ( 'NONE',  ( 72.96458098368701428, 127.0000000000000000, -80.90208098368670164 ) ) ;
#59100=AXIS2_PLACEMENT_3D ( 'NONE', #48860, #89791, #21188 ) ;
#59114=ADVANCED_FACE ( 'NONE', ( #48207, #6893 ), #74152, .F. ) ;
#59115=CARTESIAN_POINT ( 'NONE',  ( -90.31351860656789654, 74.16967745525859357, -76.80536679343883577 ) ) ;
#59123=CIRCLE ( 'NONE', #9817, 38.10000000000000142 ) ;
#59134=ADVANCED_FACE ( 'NONE', ( #6450, #81877 ), #89132, .T. ) ;
#59146=B_SPLINE_CURVE_WITH_KNOTS ( 'NONE', 3,
 ( #62773, #22356, #42319, #14189, #13739, #50028, #84141, #15542, #70050, #7818, #21914, #49581, #36434, #21459, #43218, #70961, #77313, #42761, #76865, #8274, #70501, #69153, #62329, #35062, #1466, #6922, #29607, #22809, #83243, #57296, #35971, #75969, #29163, #8733, #85038, #34624, #64134, #63683, #84593, #21004, #28249, #56849, #111, #27809, #55942, #55488, #48680, #76412, #83687 ),
 .UNSPECIFIED., .F., .F.,
 ( 4, 2, 2, 2, 2, 2, 2, 2, 2, 2, 2, 2, 2, 2, 2, 1, 2, 2, 2, 2, 2, 2, 2, 2, 4 ),
 ( 0.01987186023414422645, 0.02111356671950572958, 0.02235527320486722924, 0.02483868617559022510, 0.02608039266095170394, 0.02732209914631318279, 0.02980551211703615089, 0.03228892508775912246, 0.03353063157312059783, 0.03477233805848208015, 0.03725575102920501008, 0.03849745751456647852, 0.03973916399992794002, 0.04222257697065086302, 0.04346428345601233145, 0.04470598994137378601, 0.04594769642673525445, 0.04718940291209671595, 0.04967281588281963894, 0.05091452236818108656, 0.05215622885354252725, 0.05463964182426545024, 0.05588134830962691868, 0.05712305479498837324, 0.05960646776571126848 ),
 .UNSPECIFIED. ) ;
#59177=CARTESIAN_POINT ( 'NONE',  ( 2.332952152375709937E-14, 127.0000000000000000, 190.5000000000000000 ) ) ;
#59178=CARTESIAN_POINT ( 'NONE',  ( 118.1261869548600600, 74.80137413886471620, 10.09682577435512840 ) ) ;
#59187=VECTOR ( 'NONE', #36800, 1000.000000000000000 ) ;
#59188=DIRECTION ( 'NONE',  ( 0.000000000000000000, 0.000000000000000000, -1.000000000000000000 ) ) ;
#59196=DIRECTION ( 'NONE',  ( 0.000000000000000000, 1.000000000000000000, 0.000000000000000000 ) ) ;
#59215=VERTEX_POINT ( 'NONE', #21886 ) ;
#59269=ORIENTED_EDGE ( 'NONE', *, *, #60158, .F. ) ;
#59295=ORIENTED_EDGE ( 'NONE', *, *, #769, .T. ) ;
#59297=CARTESIAN_POINT ( 'NONE',  ( 12.61760061281885825, 84.21489741558210085, 129.9449561063389922 ) ) ;
#59308=EDGE_CURVE ( 'NONE', #24560, #14127, #28409, .T. ) ;
#59313=VECTOR ( 'NONE', #25975, 1000.000000000000000 ) ;
#59338=VERTEX_POINT ( 'NONE', #24117 ) ;
#59354=CARTESIAN_POINT ( 'NONE',  ( 103.1875000000000000, 101.5999999999999943, 3.602774393244745134E-13 ) ) ;
#59368=CARTESIAN_POINT ( 'NONE',  ( 12.70000000000000107, 82.54999999999999716, -129.9368274816650910 ) ) ;
#59369=CARTESIAN_POINT ( 'NONE',  ( 100.5868491334648382, 79.25971567868508316, -83.22961976134665463 ) ) ;
#59393=CARTESIAN_POINT ( 'NONE',  ( 118.4232890149587405, 93.94641470820114648, -5.620000134942411130 ) ) ;
#59394=AXIS2_PLACEMENT_3D ( 'NONE', #64706, #23395, #15671 ) ;
#59404=DIRECTION ( 'NONE',  ( 0.000000000000000000, 0.000000000000000000, 1.000000000000000000 ) ) ;
#59413=ORIENTED_EDGE ( 'NONE', *, *, #4173, .F. ) ;
#59424=VECTOR ( 'NONE', #81894, 1000.000000000000000 ) ;
#59430=CARTESIAN_POINT ( 'NONE',  ( -118.3661894536416099, 71.76236341257998674, 6.714990428328777128 ) ) ;
#59444=EDGE_LOOP ( 'NONE', ( #82276, #71201, #24651, #85931, #15388, #7924 ) ) ;
#59482=CARTESIAN_POINT ( 'NONE',  ( 100.8594679592218171, 82.54999999999999716, -82.89895571708191824 ) ) ;
#59484=DIRECTION ( 'NONE',  ( 0.9659258262890666469, 0.000000000000000000, 0.2588190451025269012 ) ) ;
#59495=CIRCLE ( 'NONE', #82759, 5.041900000000001825 ) ;
#59500=VECTOR ( 'NONE', #15504, 1000.000000000000114 ) ;
#59503=DIRECTION ( 'NONE',  ( 0.7071067811865510144, 0.000000000000000000, -0.7071067811865441310 ) ) ;
#59510=FACE_OUTER_BOUND ( 'NONE', #81055, .T. ) ;
#59511=CIRCLE ( 'NONE', #82773, 5.041900000000000048 ) ;
#59527=EDGE_LOOP ( 'NONE', ( #82708, #75710, #70606, #40659 ) ) ;
#59561=CIRCLE ( 'NONE', #78685, 7.143750000000004263 ) ;
#59572=DIRECTION ( 'NONE',  ( 0.000000000000000000, 0.000000000000000000, -1.000000000000000000 ) ) ;
#59600=CARTESIAN_POINT ( 'NONE',  ( 1.088711004441995877E-14, 92.07499999999998863, -88.90000000000000568 ) ) ;
#59604=ADVANCED_FACE ( 'NONE', ( #15413 ), #14053, .T. ) ;
#59606=CARTESIAN_POINT ( 'NONE',  ( -85.31568053864886281, 74.16976894168006140, 98.82395782888174551 ) ) ;
#59619=CARTESIAN_POINT ( 'NONE',  ( 117.9438495704238505, 78.46643079253873054, -12.03279974798964247 ) ) ;
#59625=ADVANCED_FACE ( 'NONE', ( #41287 ), #42627, .F. ) ;
#59636=CARTESIAN_POINT ( 'NONE',  ( 103.1875000000000000, 127.0000000000000000, 3.602774393244745134E-13 ) ) ;
#59637=ORIENTED_EDGE ( 'NONE', *, *, #26345, .F. ) ;
#59641=ADVANCED_FACE ( 'NONE', ( #27679 ), #56717, .F. ) ;
#59642=CARTESIAN_POINT ( 'NONE',  ( -11.39816346244706580, 76.93354734096725167, 118.0069729841872146 ) ) ;
#59666=CARTESIAN_POINT ( 'NONE',  ( 103.1875000000000000, 117.4749999999999943, 3.602774393244745134E-13 ) ) ;
#59677=DIRECTION ( 'NONE',  ( 0.000000000000000000, -1.000000000000000000, 0.000000000000000000 ) ) ;
#59679=CARTESIAN_POINT ( 'NONE',  ( 103.1875000000000000, 117.4749999999999943, 3.602774393244745134E-13 ) ) ;
#59689=VECTOR ( 'NONE', #64898, 1000.000000000000114 ) ;
#59698=DIRECTION ( 'NONE',  ( 0.000000000000000000, 0.000000000000000000, 1.000000000000000000 ) ) ;
#59700=CARTESIAN_POINT ( 'NONE',  ( -107.7702177616926065, 127.0000000000000000, -1.170504665415349981E-12 ) ) ;
#59702=CARTESIAN_POINT ( 'NONE',  ( -72.96458098368600531, 127.0000000000000000, -72.96458098368781009 ) ) ;
#59718=CARTESIAN_POINT ( 'NONE',  ( -74.43377912862143830, 80.88465057165899452, 92.27764637677488224 ) ) ;
#59732=CARTESIAN_POINT ( 'NONE',  ( 90.65736737572362358, 90.28416741362497078, 76.39920031718118310 ) ) ;
#59738=CARTESIAN_POINT ( 'NONE',  ( 5.616699032889737708, 93.94804372660794911, 130.4356411629704837 ) ) ;
#59749=ORIENTED_EDGE ( 'NONE', *, *, #6625, .T. ) ;
#59751=VERTEX_POINT ( 'NONE', #23742 ) ;
#59781=VERTEX_POINT ( 'NONE', #80489 ) ;
#59825=DIRECTION ( 'NONE',  ( 1.000000000000000000, 0.000000000000000000, 8.465970413060558704E-17 ) ) ;
#59838=CARTESIAN_POINT ( 'NONE',  ( 118.2599598282757114, 92.11680164986009345, -8.393562877890433427 ) ) ;
#59872=PLANE ( 'NONE',  #61538 ) ;
#59893=CARTESIAN_POINT ( 'NONE',  ( -3.174999999999664979, 124.5870000000000033, -31.75000000000000000 ) ) ;
#59903=B_SPLINE_CURVE_WITH_KNOTS ( 'NONE', 3,
 ( #67228, #33610, #60405, #59951, #88145, #87684, #18640, #73601, #25907, #25010, #19083, #47220, #45868, #12276, #67685, #61307, #5467, #74949, #19989, #12731, #40421, #68134, #38629, #89026, #26787, #54469, #66331, #55812, #76291, #34496, #82680, #21330, #62206, #89480, #77198, #28121, #75844, #49002, #63557, #49283, #886, #47670, #56269, #7257, #34040, #69931, #1341, #28579, #83563 ),
 .UNSPECIFIED., .F., .F.,
 ( 4, 2, 2, 2, 2, 2, 2, 2, 2, 2, 2, 2, 2, 2, 2, 1, 2, 2, 2, 2, 2, 2, 2, 2, 4 ),
 ( 0.01987186023414422298, 0.02111356671950572264, 0.02235527320486722577, 0.02483868617559022510, 0.02608039266095170741, 0.02732209914631318973, 0.02980551211703611619, 0.03228892508775904613, 0.03353063157312050069, 0.03477233805848195525, 0.03725575102920487131, 0.03849745751456633280, 0.03973916399992778736, 0.04222257697065069648, 0.04346428345601215798, 0.04470598994137361254, 0.04594769642673507404, 0.04718940291209652860, 0.04967281588281947241, 0.05091452236818093391, 0.05215622885354238847, 0.05463964182426533228, 0.05588134830962680766, 0.05712305479498828303, 0.05960646776571126848 ),
 .UNSPECIFIED. ) ;
#59912=CARTESIAN_POINT ( 'NONE',  ( -130.5480414536684179, 95.16896684734908263, 1.658263961150568067 ) ) ;
#59926=FACE_OUTER_BOUND ( 'NONE', #70272, .T. ) ;
#59931=CARTESIAN_POINT ( 'NONE',  ( -8.398302923777746898, 72.98741371662136146, -118.2596197875572415 ) ) ;
#59937=ADVANCED_FACE ( 'NONE', ( #77259 ), #43941, .F. ) ;
#59951=CARTESIAN_POINT ( 'NONE',  ( -117.8848147242576374, 84.21376545118702950, -12.59751181725430946 ) ) ;
#59967=EDGE_CURVE ( 'NONE', #38484, #63081, #58032, .T. ) ;
#59973=CARTESIAN_POINT ( 'NONE',  ( -72.96458098368600531, 101.5999999999999943, -72.96458098368781009 ) ) ;
#59979=VECTOR ( 'NONE', #82518, 1000.000000000000000 ) ;
#59987=CARTESIAN_POINT ( 'NONE',  ( 130.4667775723041814, 94.30053010088478516, -4.871090541622842274 ) ) ;
#60049=EDGE_CURVE ( 'NONE', #28641, #7172, #38468, .T. ) ;
#60063=CARTESIAN_POINT ( 'NONE',  ( 118.1708971306823486, 74.16967745525860778, -9.551705748360291182 ) ) ;
#60064=B_SPLINE_CURVE_WITH_KNOTS ( 'NONE', 3,
 ( #77524, #1677, #62540, #49796, #36643, #57513, #48888, #56614, #35273, #23021, #16199, #83440, #762, #64345, #76626, #8488, #84358, #29380, #8030, #62983, #316, #28462, #56152, #29826, #55690, #42972, #43877, #7137, #34833, #22570, #15306, #35724, #63439, #83903, #1225, #21674, #28013, #50243, #14408, #77978, #63900, #49348, #42083, #57057, #69814, #77079, #43424, #7587, #14861 ),
 .UNSPECIFIED., .F., .F.,
 ( 4, 2, 2, 2, 2, 2, 2, 2, 2, 2, 2, 2, 2, 2, 2, 1, 2, 2, 2, 2, 2, 2, 2, 2, 4 ),
 ( 0.01986933033599076401, 0.02111088875730812026, 0.02235244717862547650, 0.02483556402126018900, 0.02607712244257756606, 0.02731868086389493966, 0.02980179770652969379, 0.03228491454916444792, 0.03352647297048182151, 0.03476803139179918817, 0.03725114823443395617, 0.03849270665575131589, 0.03973426507706866173, 0.04221738191970339504, 0.04345894034102079639, 0.04470049876233819081, 0.04594205718365558522, 0.04718361560497297963, 0.04966673244760778927, 0.05090829086892520450, 0.05214984929024261973, 0.05463296613287743630, 0.05587452455419480990, 0.05711608297551218349, 0.05959919981814693069 ),
 .UNSPECIFIED. ) ;
#60070=ORIENTED_EDGE ( 'NONE', *, *, #15554, .F. ) ;
#60072=DIRECTION ( 'NONE',  ( 0.000000000000000000, 1.000000000000000000, 0.000000000000000000 ) ) ;
#60080=CIRCLE ( 'NONE', #34024, 7.143749999999999822 ) ;
#60092=ORIENTED_EDGE ( 'NONE', *, *, #78704, .F. ) ;
#60098=AXIS2_PLACEMENT_3D ( 'NONE', #514, #22315, #63645 ) ;
#60153=ORIENTED_EDGE ( 'NONE', *, *, #15096, .T. ) ;
#60158=EDGE_CURVE ( 'NONE', #1704, #19337, #63304, .T. ) ;
#60177=AXIS2_PLACEMENT_3D ( 'NONE', #25439, #54459, #42089 ) ;
#60191=VERTEX_POINT ( 'NONE', #7547 ) ;
#60194=ORIENTED_EDGE ( 'NONE', *, *, #4173, .T. ) ;
#60246=CIRCLE ( 'NONE', #89327, 7.143750000000004263 ) ;
#60258=CARTESIAN_POINT ( 'NONE',  ( 6.359443759653470529, 93.55095829381066608, -130.4015408541779379 ) ) ;
#60259=AXIS2_PLACEMENT_3D ( 'NONE', #48988, #20425, #35374 ) ;
#60272=VECTOR ( 'NONE', #24811, 1000.000000000000000 ) ;
#60281=ORIENTED_EDGE ( 'NONE', *, *, #29471, .T. ) ;
#60288=CARTESIAN_POINT ( 'NONE',  ( 118.4880192609368379, 94.60304557064716846, 4.087421425393760188 ) ) ;
#60298=DIRECTION ( 'NONE',  ( 0.8660254037844392627, 0.000000000000000000, 0.4999999999999990563 ) ) ;
#60306=ORIENTED_EDGE ( 'NONE', *, *, #64665, .T. ) ;
#60318=CARTESIAN_POINT ( 'NONE',  ( -118.3861417219090129, 71.54629894495526798, 6.354613972969239910 ) ) ;
#60334=ADVANCED_FACE ( 'NONE', ( #42936 ), #77480, .F. ) ;
#60346=DIRECTION ( 'NONE',  ( 0.000000000000000000, 0.000000000000000000, 1.000000000000000000 ) ) ;
#60363=CARTESIAN_POINT ( 'NONE',  ( -130.4355093393840548, 93.94653598907719072, 5.619751006019208184 ) ) ;
#60375=ORIENTED_EDGE ( 'NONE', *, *, #30625, .F. ) ;
#60379=PLANE ( 'NONE',  #17077 ) ;
#60388=VECTOR ( 'NONE', #31567, 1000.000000000000000 ) ;
#60399=FACE_OUTER_BOUND ( 'NONE', #21251, .T. ) ;
#60405=CARTESIAN_POINT ( 'NONE',  ( -117.8759966127889527, 83.38015080693119785, -12.67975824297045051 ) ) ;
#60411=EDGE_LOOP ( 'NONE', ( #86036, #67558, #9079, #11121 ) ) ;
#60422=CARTESIAN_POINT ( 'NONE',  ( 91.61507027739585851, 87.79588542099533299, -75.24778849303586981 ) ) ;
#60426=VECTOR ( 'NONE', #26362, 1000.000000000000000 ) ;
#60460=CARTESIAN_POINT ( 'NONE',  ( -92.06079644778172621, 79.26437155269049128, -74.70173812346064324 ) ) ;
#60469=ORIENTED_EDGE ( 'NONE', *, *, #63709, .T. ) ;
#60474=CARTESIAN_POINT ( 'NONE',  ( -3.968749999999949818, 120.6499999999999915, -105.4788588808462038 ) ) ;
#60516=CARTESIAN_POINT ( 'NONE',  ( -98.60478223830740774, 127.0000000000000000, -1.074461880482445986E-12 ) ) ;
#60537=EDGE_CURVE ( 'NONE', #79701, #10974, #11103, .T. ) ;
#60562=ADVANCED_FACE ( 'NONE', ( #58366 ), #31101, .F. ) ;
#60579=DIRECTION ( 'NONE',  ( 6.982966722218760189E-15, 0.000000000000000000, -1.000000000000000000 ) ) ;
#60598=CARTESIAN_POINT ( 'NONE',  ( 103.1875000000000000, 127.0000000000000000, 3.602774393244745134E-13 ) ) ;
#60612=CARTESIAN_POINT ( 'NONE',  ( 103.1875000000000000, 127.0000000000000000, 3.602774393244745134E-13 ) ) ;
#60614=CARTESIAN_POINT ( 'NONE',  ( -76.39898589339149737, 74.81620433377383961, 90.65754775988004610 ) ) ;
#60659=DIRECTION ( 'NONE',  ( 0.000000000000000000, 1.000000000000000000, 0.000000000000000000 ) ) ;
#60661=EDGE_LOOP ( 'NONE', ( #66984, #45223, #85770, #32547 ) ) ;
#60671=CARTESIAN_POINT ( 'NONE',  ( -72.96458098368600531, 127.0000000000000000, -72.96458098368781009 ) ) ;
#60673=CARTESIAN_POINT ( 'NONE',  ( 130.0906838859329469, 76.18750001922978754, -11.02255322708036900 ) ) ;
#60695=LINE ( 'NONE', #12570, #77623 ) ;
#60697=AXIS2_PLACEMENT_3D ( 'NONE', #86740, #66726, #24951 ) ;
#60706=CARTESIAN_POINT ( 'NONE',  ( 7.746062721843873788, 92.64813751154242993, -130.3278237768880956 ) ) ;
#60735=CARTESIAN_POINT ( 'NONE',  ( 118.4407179355509072, 94.12556101775334128, 5.241146580996987048 ) ) ;
#60740=ADVANCED_FACE ( 'NONE', ( #62385 ), #165, .F. ) ;
#60772=EDGE_LOOP ( 'NONE', ( #44630, #78416, #4687, #13547 ) ) ;
#60789=DIRECTION ( 'NONE',  ( 0.000000000000000000, -1.000000000000000000, 0.000000000000000000 ) ) ;
#60807=VERTEX_POINT ( 'NONE', #42824 ) ;
#60809=CARTESIAN_POINT ( 'NONE',  ( 74.15067561874269586, 127.0000000000000000, -68.53801554307419508 ) ) ;
#60829=CARTESIAN_POINT ( 'NONE',  ( 92.60677566276832806, 95.25015599858946302, -92.02731164704627531 ) ) ;
#60855=CIRCLE ( 'NONE', #21721, 5.041900000000001825 ) ;
#60860=CARTESIAN_POINT ( 'NONE',  ( -83.15057989154965412, 85.43248893795411902, 100.6521573293566121 ) ) ;
#60864=EDGE_LOOP ( 'NONE', ( #69289, #22265, #72542, #59637 ) ) ;
#60870=ORIENTED_EDGE ( 'NONE', *, *, #18613, .F. ) ;
#60874=VECTOR ( 'NONE', #7560, 1000.000000000000000 ) ;
#60903=CARTESIAN_POINT ( 'NONE',  ( 130.0134714785366157, 87.03008507238369873, -11.89083589963720122 ) ) ;
#60913=CARTESIAN_POINT ( 'NONE',  ( -12.37565694608801437, 79.66829940370548968, -129.9681453810340770 ) ) ;
#60916=VECTOR ( 'NONE', #60579, 1000.000000000000000 ) ;
#60938=FACE_OUTER_BOUND ( 'NONE', #1381, .T. ) ;
#60946=FACE_OUTER_BOUND ( 'NONE', #49835, .T. ) ;
#60947=DIRECTION ( 'NONE',  ( 0.000000000000000000, 0.000000000000000000, -1.000000000000000000 ) ) ;
#60952=LINE ( 'NONE', #88681, #81087 ) ;
#60992=FACE_OUTER_BOUND ( 'NONE', #85013, .T. ) ;
#61007=CARTESIAN_POINT ( 'NONE',  ( 107.7702177616926065, 120.6499999999999915, 4.179089330879380409E-13 ) ) ;
#61012=CARTESIAN_POINT ( 'NONE',  ( 5.617021782840719624, 93.94788616487885236, 118.4234307144629383 ) ) ;
#61045=CARTESIAN_POINT ( 'NONE',  ( -4.087988121205965442, 94.58126409692587799, -118.4861679838275990 ) ) ;
#61052=CARTESIAN_POINT ( 'NONE',  ( 71.77848634863079269, 120.6499999999999915, 77.39114642429989033 ) ) ;
#61054=DIRECTION ( 'NONE',  ( 0.000000000000000000, 1.000000000000000000, 0.000000000000000000 ) ) ;
#61061=ADVANCED_FACE ( 'NONE', ( #60938 ), #48188, .F. ) ;
#61072=CARTESIAN_POINT ( 'NONE',  ( 72.96458098368650269, 101.5999999999999943, 72.96458098368729850 ) ) ;
#61076=ORIENTED_EDGE ( 'NONE', *, *, #12456, .T. ) ;
#61088=CARTESIAN_POINT ( 'NONE',  ( 91.51255889651523034, 88.18374315479978520, 75.37293521528393114 ) ) ;
#61096=CARTESIAN_POINT ( 'NONE',  ( -89.95943163722107272, 94.84315624882771090, -94.61941200740686497 ) ) ;
#61102=VERTEX_POINT ( 'NONE', #75920 ) ;
#61106=CARTESIAN_POINT ( 'NONE',  ( 0.000000000000000000, 92.07499999999998863, 0.000000000000000000 ) ) ;
#61119=ORIENTED_EDGE ( 'NONE', *, *, #16463, .F. ) ;
#61132=CARTESIAN_POINT ( 'NONE',  ( 129.9777455398983079, 79.26455342200333121, -12.27475243032916907 ) ) ;
#61221=LINE ( 'NONE', #74432, #36724 ) ;
#61226=VERTEX_POINT ( 'NONE', #71365 ) ;
#61241=CIRCLE ( 'NONE', #88828, 7.143750000000004263 ) ;
#61260=EDGE_CURVE ( 'NONE', #22549, #72980, #15944, .T. ) ;
#61270=VERTEX_POINT ( 'NONE', #70459 ) ;
#61305=AXIS2_PLACEMENT_3D ( 'NONE', #59973, #66805, #87706 ) ;
#61307=CARTESIAN_POINT ( 'NONE',  ( -118.3663208563465759, 93.33902940301969409, -6.712516165662615109 ) ) ;
#61340=CARTESIAN_POINT ( 'NONE',  ( 130.0919229099369545, 88.91113633199481114, 10.99998730946224690 ) ) ;
#61405=CARTESIAN_POINT ( 'NONE',  ( -88.80809839403299577, 70.80031561532533146, 95.69968022530751739 ) ) ;
#61408=ORIENTED_EDGE ( 'NONE', *, *, #20287, .F. ) ;
#61417=PLANE ( 'NONE',  #6695 ) ;
#61425=CARTESIAN_POINT ( 'NONE',  ( -92.90380151375030948, 69.84937019662270075, -91.73035097708769570 ) ) ;
#61448=CARTESIAN_POINT ( 'NONE',  ( 4.087988121205971659, 94.58126409692583536, 118.4861679838275847 ) ) ;
#61465=EDGE_CURVE ( 'NONE', #32614, #9318, #87287, .T. ) ;
#61480=CYLINDRICAL_SURFACE ( 'NONE', #77301, 38.10000000000000142 ) ;
#61481=ADVANCED_FACE ( 'NONE', ( #81753, #59926 ), #60379, .F. ) ;
#61487=EDGE_CURVE ( 'NONE', #81025, #27593, #75372, .T. ) ;
#61508=CARTESIAN_POINT ( 'NONE',  ( 103.1875000000000000, 127.0000000000000000, 3.602774393244745134E-13 ) ) ;
#61529=VERTEX_POINT ( 'NONE', #68108 ) ;
#61532=DIRECTION ( 'NONE',  ( -0.000000000000000000, 1.000000000000000000, 0.000000000000000000 ) ) ;
#61538=AXIS2_PLACEMENT_3D ( 'NONE', #80803, #87605, #69848 ) ;
#61549=EDGE_LOOP ( 'NONE', ( #86055, #48363, #13233, #27643 ) ) ;
#61559=EDGE_CURVE ( 'NONE', #40068, #5885, #40274, .T. ) ;
#61570=CARTESIAN_POINT ( 'NONE',  ( -129.9681746291968238, 79.66695435136418268, 12.37535028237962642 ) ) ;
#61575=ORIENTED_EDGE ( 'NONE', *, *, #55187, .T. ) ;
#61619=DIRECTION ( 'NONE',  ( 0.000000000000000000, 1.000000000000000000, 0.000000000000000000 ) ) ;
#61620=EDGE_CURVE ( 'NONE', #1670, #36775, #59123, .T. ) ;
#61624=EDGE_LOOP ( 'NONE', ( #20240, #20490, #2812, #34543 ) ) ;
#61630=CARTESIAN_POINT ( 'NONE',  ( 2.332952152375709937E-14, 103.1240000000000236, 190.5000000000000000 ) ) ;
#61649=PRODUCT_DEFINITION ( 'UNKNOWN', '', #26149, #43264 ) ;
#61650=PLANE ( 'NONE',  #69267 ) ;
#61678=ADVANCED_FACE ( 'NONE', ( #29016 ), #78074, .F. ) ;
#61696=CARTESIAN_POINT ( 'NONE',  ( 59.93649209371597664, 82.54999999999999716, -77.89700433585308303 ) ) ;
#61705=CARTESIAN_POINT ( 'NONE',  ( -129.9368274816652047, 83.38918798244692709, 12.69999999999955165 ) ) ;
#61712=ORIENTED_EDGE ( 'NONE', *, *, #84720, .T. ) ;
#61719=DIRECTION ( 'NONE',  ( 0.000000000000000000, 1.000000000000000000, 0.000000000000000000 ) ) ;
#61751=DIRECTION ( 'NONE',  ( 0.000000000000000000, 0.000000000000000000, -1.000000000000000000 ) ) ;
#61764=CARTESIAN_POINT ( 'NONE',  ( 91.50010255991666952, 88.17653575778736297, -75.38763434846433142 ) ) ;
#61776=CARTESIAN_POINT ( 'NONE',  ( 59.93649209371435660, 82.54999999999999716, 77.89700433585434780 ) ) ;
#61783=CARTESIAN_POINT ( 'NONE',  ( 130.1467854596290579, 89.94765885072629885, -10.33135106516608204 ) ) ;
#61784=VECTOR ( 'NONE', #14991, 1000.000000000000000 ) ;
#61795=CARTESIAN_POINT ( 'NONE',  ( -2.899933897858971488, 70.17843983949715891, -130.5244343740981776 ) ) ;
#61802=EDGE_CURVE ( 'NONE', #64147, #4701, #11284, .T. ) ;
#61820=CARTESIAN_POINT ( 'NONE',  ( 88.80809839403359263, 70.80031561532540252, -95.69968022530694896 ) ) ;
#61825=DIRECTION ( 'NONE',  ( 0.000000000000000000, 1.000000000000000000, 0.000000000000000000 ) ) ;
#61826=CARTESIAN_POINT ( 'NONE',  ( 6.360060842339565923, 71.54945291875249325, 118.3858484385471286 ) ) ;
#61844=CARTESIAN_POINT ( 'NONE',  ( -100.8594679592211918, 81.72130195885945625, 82.89895571708260036 ) ) ;
#61859=EDGE_CURVE ( 'NONE', #83766, #78870, #73017, .T. ) ;
#61897=ORIENTED_EDGE ( 'NONE', *, *, #26734, .F. ) ;
#61915=EDGE_CURVE ( 'NONE', #45031, #22549, #34250, .T. ) ;
#61916=AXIS2_PLACEMENT_3D ( 'NONE', #58004, #85737, #48925 ) ;
#61932=CARTESIAN_POINT ( 'NONE',  ( 12.70000000000000107, 82.54999999999999716, -117.8738102209307641 ) ) ;
#61946=DIRECTION ( 'NONE',  ( 0.000000000000000000, 1.000000000000000000, 0.000000000000000000 ) ) ;
#61960=CARTESIAN_POINT ( 'NONE',  ( -88.90442867305931429, 72.22378176823141871, 78.43243611888119915 ) ) ;
#61984=CARTESIAN_POINT ( 'NONE',  ( -90.83954799657452384, 95.08644067748866746, -93.77212533081383583 ) ) ;
#62002=EDGE_CURVE ( 'NONE', #68541, #81147, #20637, .T. ) ;
#62013=DIRECTION ( 'NONE',  ( -8.465970413060558704E-17, 0.000000000000000000, 1.000000000000000000 ) ) ;
#62024=ORIENTED_EDGE ( 'NONE', *, *, #12456, .F. ) ;
#62025=CARTESIAN_POINT ( 'NONE',  ( 130.1658077747426319, 74.80151635532865839, 10.09693588310459766 ) ) ;
#62029=FACE_OUTER_BOUND ( 'NONE', #2999, .T. ) ;
#62048=EDGE_CURVE ( 'NONE', #83626, #53265, #17137, .T. ) ;
#62065=AXIS2_PLACEMENT_3D ( 'NONE', #951, #42265, #7765 ) ;
#62096=VERTEX_POINT ( 'NONE', #16503 ) ;
#62105=EDGE_CURVE ( 'NONE', #16980, #79245, #2432, .T. ) ;
#62114=CARTESIAN_POINT ( 'NONE',  ( -1.663885868249260769, 95.14749804389165888, 118.5450564992234064 ) ) ;
#62121=CARTESIAN_POINT ( 'NONE',  ( -117.8738102209307215, 81.72118090664557144, -12.70000000000041496 ) ) ;
#62124=VECTOR ( 'NONE', #50596, 1000.000000000000000 ) ;
#62129=CARTESIAN_POINT ( 'NONE',  ( 1.665763066381118485, 69.93250922127340630, -118.5470808886261125 ) ) ;
#62133=VERTEX_POINT ( 'NONE', #84220 ) ;
#62163=CARTESIAN_POINT ( 'NONE',  ( 100.3415888741731550, 78.07027470200927155, 83.52520760052999549 ) ) ;
#62177=AXIS2_PLACEMENT_3D ( 'NONE', #52512, #18020, #45703 ) ;
#62184=VERTEX_POINT ( 'NONE', #70578 ) ;
#62194=EDGE_CURVE ( 'NONE', #40277, #37737, #70120, .T. ) ;
#62206=CARTESIAN_POINT ( 'NONE',  ( -118.3862315815643882, 93.55466788070663142, 6.352948492897542820 ) ) ;
#62207=DIRECTION ( 'NONE',  ( 0.000000000000000000, 0.000000000000000000, 1.000000000000000000 ) ) ;
#62210=CARTESIAN_POINT ( 'NONE',  ( 0.000000000000000000, 82.54999999999999716, -97.46299999999996544 ) ) ;
#62220=CARTESIAN_POINT ( 'NONE',  ( -82.89895571708225930, 82.54999999999999716, -100.8594679592215471 ) ) ;
#62262=CARTESIAN_POINT ( 'NONE',  ( -84.99964240976918006, 69.93120980984940616, -82.65143893653593921 ) ) ;
#62272=ADVANCED_FACE ( 'NONE', ( #18272 ), #10567, .F. ) ;
#62284=ADVANCED_FACE ( 'NONE', ( #11470, #31449 ), #39605, .T. ) ;
#62289=DIRECTION ( 'NONE',  ( 1.000000000000000000, 0.000000000000000000, 0.000000000000000000 ) ) ;
#62292=ORIENTED_EDGE ( 'NONE', *, *, #62497, .F. ) ;
#62302=CARTESIAN_POINT ( 'NONE',  ( -3.174999999999644995, 111.1250000000000000, -33.98325472291465132 ) ) ;
#62305=CARTESIAN_POINT ( 'NONE',  ( -97.62852612868731228, 72.47310549519059464, 86.68128281353570230 ) ) ;
#62308=ORIENTED_EDGE ( 'NONE', *, *, #4272, .T. ) ;
#62319=CARTESIAN_POINT ( 'NONE',  ( 0.000000000000000000, 111.1250000000000000, 0.000000000000000000 ) ) ;
#62329=CARTESIAN_POINT ( 'NONE',  ( -82.65057572782323803, 95.14807216649714405, -84.99753727674128356 ) ) ;
#62334=ORIENTED_EDGE ( 'NONE', *, *, #29820, .F. ) ;
#62336=VECTOR ( 'NONE', #46027, 1000.000000000000114 ) ;
#62349=CARTESIAN_POINT ( 'NONE',  ( 107.7702177616926065, 127.0000000000000000, 4.185020385794044591E-13 ) ) ;
#62376=DIRECTION ( 'NONE',  ( 0.000000000000000000, 1.000000000000000000, 0.000000000000000000 ) ) ;
#62385=FACE_OUTER_BOUND ( 'NONE', #74073, .T. ) ;
#62422=DIRECTION ( 'NONE',  ( 0.9659258262890670910, 0.000000000000000000, 0.2588190451025250693 ) ) ;
#62439=CIRCLE ( 'NONE', #76902, 42.54500000000000171 ) ;
#62454=ORIENTED_EDGE ( 'NONE', *, *, #7251, .T. ) ;
#62477=CARTESIAN_POINT ( 'NONE',  ( -129.9449656991350253, 80.88456863959032717, 12.61750076990854552 ) ) ;
#62488=CARTESIAN_POINT ( 'NONE',  ( 72.96458098368650269, 117.4749999999999943, 72.96458098368729850 ) ) ;
#62497=EDGE_CURVE ( 'NONE', #46818, #53446, #60952, .T. ) ;
#62501=DIRECTION ( 'NONE',  ( -3.576143065239989638E-15, 0.000000000000000000, 1.000000000000000000 ) ) ;
#62505=EDGE_CURVE ( 'NONE', #81090, #6159, #28676, .T. ) ;
#62511=FACE_OUTER_BOUND ( 'NONE', #76988, .T. ) ;
#62515=DIRECTION ( 'NONE',  ( 0.7071067811865415775, 0.000000000000000000, 0.7071067811865535679 ) ) ;
#62537=CARTESIAN_POINT ( 'NONE',  ( 103.1875000000000000, 127.0000000000000000, 7.143750000000359535 ) ) ;
#62540=CARTESIAN_POINT ( 'NONE',  ( 82.91466710319107847, 83.38002811471483255, 100.8465607796074011 ) ) ;
#62546=EDGE_LOOP ( 'NONE', ( #25123, #42732, #84981, #57794 ) ) ;
#62549=EDGE_CURVE ( 'NONE', #29308, #34288, #35477, .T. ) ;
#62554=FACE_OUTER_BOUND ( 'NONE', #55838, .T. ) ;
#62561=CIRCLE ( 'NONE', #7460, 7.143750000000004263 ) ;
#62564=CARTESIAN_POINT ( 'NONE',  ( -3.299336700116765719, 94.84201444875799325, 118.5128796971597467 ) ) ;
#62567=EDGE_CURVE ( 'NONE', #12422, #14878, #29133, .T. ) ;
#62570=CARTESIAN_POINT ( 'NONE',  ( -117.8738102209307215, 82.54999999999999716, -12.70000000000041318 ) ) ;
#62582=CIRCLE ( 'NONE', #43706, 34.13125000000000142 ) ;
#62584=ORIENTED_EDGE ( 'NONE', *, *, #49953, .T. ) ;
#62615=CARTESIAN_POINT ( 'NONE',  ( 88.24354053934726494, 71.14122173980733521, 96.22129751242573548 ) ) ;
#62644=FACE_OUTER_BOUND ( 'NONE', #17809, .T. ) ;
#62654=CARTESIAN_POINT ( 'NONE',  ( -92.31685958143586390, 83.38015080693119785, 74.38497350661531016 ) ) ;
#62659=CARTESIAN_POINT ( 'NONE',  ( 76.20754074253719068, 75.15251084995277608, -90.81844170390297677 ) ) ;
#62660=ORIENTED_EDGE ( 'NONE', *, *, #21401, .T. ) ;
#62665=ORIENTED_EDGE ( 'NONE', *, *, #28939, .F. ) ;
#62684=EDGE_LOOP ( 'NONE', ( #67254, #39584 ) ) ;
#62687=DIRECTION ( 'NONE',  ( -6.982966722218760189E-15, 0.000000000000000000, 1.000000000000000000 ) ) ;
#62714=CARTESIAN_POINT ( 'NONE',  ( -87.20837788851378036, 70.80054595721396993, -80.31601367611384035 ) ) ;
#62728=DIRECTION ( 'NONE',  ( -0.4999999999999998890, 0.000000000000000000, 0.8660254037844387076 ) ) ;
#62733=CARTESIAN_POINT ( 'NONE',  ( 68.53801554307389665, 127.0000000000000000, 74.15067561874289481 ) ) ;
#62735=CARTESIAN_POINT ( 'NONE',  ( 9.275582543403935176, 73.86526018886296185, 118.1929554227103267 ) ) ;
#62753=CARTESIAN_POINT ( 'NONE',  ( -100.6522392491099112, 79.66749569656610674, 83.15048135366490101 ) ) ;
#62773=CARTESIAN_POINT ( 'NONE',  ( -74.36911441044668436, 82.54999999999999716, -92.32962665258587265 ) ) ;
#62782=CIRCLE ( 'NONE', #78774, 7.937500000000000000 ) ;
#62809=CARTESIAN_POINT ( 'NONE',  ( 3.968749999999229949, 120.6499999999999915, 100.8961411191535973 ) ) ;
#62844=CARTESIAN_POINT ( 'NONE',  ( 129.9468070739257257, 84.21348395916258767, 12.59754631664314317 ) ) ;
#62858=CARTESIAN_POINT ( 'NONE',  ( -77.68655577178658689, 72.98405218941670114, 89.55818655986143995 ) ) ;
#62870=DIRECTION ( 'NONE',  ( 0.000000000000000000, 0.000000000000000000, 1.000000000000000000 ) ) ;
#62887=CARTESIAN_POINT ( 'NONE',  ( 69.72411017812960665, 127.0000000000000000, 69.72411017813040246 ) ) ;
#62896=CARTESIAN_POINT ( 'NONE',  ( -76.20505178924278766, 120.6499999999999915, -76.20505178924469192 ) ) ;
#62922=CARTESIAN_POINT ( 'NONE',  ( 130.2871811975776382, 72.98383416765814502, -8.394281761908146677 ) ) ;
#62932=DIRECTION ( 'NONE',  ( 0.000000000000000000, 1.000000000000000000, 0.000000000000000000 ) ) ;
#62942=DIRECTION ( 'NONE',  ( 0.000000000000000000, 1.000000000000000000, 0.000000000000000000 ) ) ;
#62957=CARTESIAN_POINT ( 'NONE',  ( 72.96458098368650269, 101.5999999999999943, 78.00648098368728256 ) ) ;
#62962=VECTOR ( 'NONE', #76899, 1000.000000000000000 ) ;
#62983=CARTESIAN_POINT ( 'NONE',  ( 89.38347482486577178, 94.60320878023492241, 95.16331303980217626 ) ) ;
#62990=ORIENTED_EDGE ( 'NONE', *, *, #72591, .F. ) ;
#63002=ORIENTED_EDGE ( 'NONE', *, *, #25695, .F. ) ;
#63007=CARTESIAN_POINT ( 'NONE',  ( -2.078103260390279150, 95.08570091005914549, 118.5384849238115805 ) ) ;
#63074=CARTESIAN_POINT ( 'NONE',  ( -7.205548786489490269E-13, 101.5999999999999943, 108.2293999999999983 ) ) ;
#63081=VERTEX_POINT ( 'NONE', #84903 ) ;
#63094=PLANE ( 'NONE',  #39413 ) ;
#63098=AXIS2_PLACEMENT_3D ( 'NONE', #17289, #86774, #71371 ) ;
#63104=DIRECTION ( 'NONE',  ( 0.000000000000000000, 1.000000000000000000, 0.000000000000000000 ) ) ;
#63135=ORIENTED_EDGE ( 'NONE', *, *, #63219, .F. ) ;
#63140=DIRECTION ( 'NONE',  ( 0.000000000000000000, 0.000000000000000000, 1.000000000000000000 ) ) ;
#63143=EDGE_CURVE ( 'NONE', #5947, #37208, #7152, .T. ) ;
#63144=CARTESIAN_POINT ( 'NONE',  ( 98.60478223830740774, 120.6499999999999915, 3.859079674607175002E-13 ) ) ;
#63155=CARTESIAN_POINT ( 'NONE',  ( 0.000000000000000000, 117.4749999999999943, -103.1875000000000000 ) ) ;
#63161=FACE_OUTER_BOUND ( 'NONE', #35238, .T. ) ;
#63163=CARTESIAN_POINT ( 'NONE',  ( -79.74945239053502632, 71.14137858619481847, -87.72765544449623576 ) ) ;
#63165=CARTESIAN_POINT ( 'NONE',  ( 103.1875000000000000, 117.4749999999999943, 3.602774393244745134E-13 ) ) ;
#63179=CARTESIAN_POINT ( 'NONE',  ( 82.89895571708363775, 81.71102547120852932, -100.8594679592203960 ) ) ;
#63208=CARTESIAN_POINT ( 'NONE',  ( -96.71266027437708601, 71.53177522571070313, 87.70409100286397575 ) ) ;
#63219=EDGE_CURVE ( 'NONE', #64147, #2062, #5343, .T. ) ;
#63224=LINE ( 'NONE', #15081, #14025 ) ;
#63229=ADVANCED_FACE ( 'NONE', ( #33483, #18509 ), #20325, .T. ) ;
#63240=LINE ( 'NONE', #43226, #39328 ) ;
#63254=CARTESIAN_POINT ( 'NONE',  ( -103.1875000000000000, 127.0000000000000000, 7.937499999998919087 ) ) ;
#63258=ORIENTED_EDGE ( 'NONE', *, *, #70286, .F. ) ;
#63260=DIRECTION ( 'NONE',  ( 0.000000000000000000, -1.000000000000000000, 0.000000000000000000 ) ) ;
#63266=FACE_OUTER_BOUND ( 'NONE', #7450, .T. ) ;
#63304=CIRCLE ( 'NONE', #9615, 5.041900000000000048 ) ;
#63318=CARTESIAN_POINT ( 'NONE',  ( -81.76234319299368281, 70.17658267799284033, 85.85227416678179679 ) ) ;
#63354=ORIENTED_EDGE ( 'NONE', *, *, #84999, .F. ) ;
#63366=CARTESIAN_POINT ( 'NONE',  ( 100.8961411191535973, 120.6499999999999915, 3.968750000000400124 ) ) ;
#63369=EDGE_LOOP ( 'NONE', ( #62454, #85232, #22482, #2166 ) ) ;
#63373=DIRECTION ( 'NONE',  ( 1.000000000000000000, 0.000000000000000000, 0.000000000000000000 ) ) ;
#63379=CARTESIAN_POINT ( 'NONE',  ( 130.3836616406707094, 71.76234181793742550, -6.714949744937471543 ) ) ;
#63386=CLOSED_SHELL ( 'NONE', ( #61678, #2679, #86827, #12261, #5814, #21895, #42659, #45554, #33484, #32557, #5283, #73061, #28988, #27627, #84491, #29236, #86399, #2389, #69704, #5407, #56154, #52626, #86459, #43626, #8716, #23311, #13904, #25994, #10828, #431, #40757, #24148, #84328, #46885, #52723, #71478, #37083, #67931, #46874, #11887, #55234, #28123, #45239, #82461, #87547, #70647, #73453, #67941, #44230, #89106, #31655, #54270, #73580, #87847, #1766, #17921, #80975, #82923, #34310, #47368, #21218, #54150, #28124, #13338, #69058, #70750, #45649, #31415, #80343, #60334, #73690, #83801, #49371, #76114, #6452, #35660, #79448, #17504, #54611, #34599, #11361, #59937, #42576, #54722, #66191, #89187, #72839, #25478, #53478, #61061, #883, #47508, #41274, #37998, #63229, #14380, #40760, #71327, #8052, #59134, #45267, #75046, #11199, #75538, #19845, #32544, #10190, #1610, #87934, #39447, #13587, #9701, #69491, #80677, #86233, #29524, #70572, #2623, #2338, #3355, #9024, #81578, #51591, #68131, #3016, #57576, #44332, #59604, #76798, #13931, #51128, #64, #61481, #59114, #5776, #66483, #74139, #82311, #8971, #11432, #62272, #49192, #66, #58420, #755, #65479, #45849, #79823, #25250, #49256, #34910, #23788, #36369, #11944, #85126, #76674, #57596, #35886, #45928, #41900, #80266, #85192, #15042, #68149, #45526, #60562, #78492, #23669, #87121, #71889, #10133, #15164, #75772, #66806, #57736, #32105, #62284, #30448, #370, #60740, #39264, #13183, #73373, #77307, #59641, #18708, #9931, #75984, #35223, #70945, #59625 ) ) ;
#63392=CARTESIAN_POINT ( 'NONE',  ( -69.72411017813060141, 127.0000000000000000, 69.72411017812929401 ) ) ;
#63400=DIRECTION ( 'NONE',  ( 0.4999999999999995004, 0.000000000000000000, -0.8660254037844390407 ) ) ;
#63412=CARTESIAN_POINT ( 'NONE',  ( 31.75000000000000000, 124.5870000000000033, -3.174999999999999822 ) ) ;
#63417=EDGE_CURVE ( 'NONE', #43612, #54367, #42081, .T. ) ;
#63421=VERTEX_POINT ( 'NONE', #42525 ) ;
#63434=ORIENTED_EDGE ( 'NONE', *, *, #67433, .F. ) ;
#63439=CARTESIAN_POINT ( 'NONE',  ( 96.70003673985384296, 93.55484823631827851, 87.71605664019050153 ) ) ;
#63440=CARTESIAN_POINT ( 'NONE',  ( 68.53801554307389665, 120.6499999999999915, 74.15067561874289481 ) ) ;
#63467=ORIENTED_EDGE ( 'NONE', *, *, #41078, .T. ) ;
#63483=VERTEX_POINT ( 'NONE', #23903 ) ;
#63491=EDGE_CURVE ( 'NONE', #29444, #86064, #8585, .T. ) ;
#63511=CARTESIAN_POINT ( 'NONE',  ( 96.20681132576044092, 71.15434825076368952, 88.25674559704650335 ) ) ;
#63531=DIRECTION ( 'NONE',  ( 0.000000000000000000, 0.000000000000000000, 1.000000000000000000 ) ) ;
#63537=ORIENTED_EDGE ( 'NONE', *, *, #84676, .T. ) ;
#63552=CARTESIAN_POINT ( 'NONE',  ( -84.99753727674097092, 95.14807216649714405, 82.65057572782355066 ) ) ;
#63557=CARTESIAN_POINT ( 'NONE',  ( -118.1268318574024221, 90.28416741362501341, 10.08204661438704619 ) ) ;
#63559=CARTESIAN_POINT ( 'NONE',  ( 80.88709205069450547, 70.52090377575432001, -86.67734222162502533 ) ) ;
#63567=EDGE_CURVE ( 'NONE', #32260, #79836, #36013, .T. ) ;
#63576=FACE_BOUND ( 'NONE', #24555, .T. ) ;
#63630=CARTESIAN_POINT ( 'NONE',  ( 96.22129751242547968, 71.14122173980733521, -88.24354053934760600 ) ) ;
#63631=LINE ( 'NONE', #29116, #32231 ) ;
#63637=DIRECTION ( 'NONE',  ( 0.7071067811865460184, 0.000000000000000000, 0.7071067811865489050 ) ) ;
#63645=DIRECTION ( 'NONE',  ( 0.000000000000000000, 0.000000000000000000, 1.000000000000000000 ) ) ;
#63669=CARTESIAN_POINT ( 'NONE',  ( 103.1875000000000000, 127.0000000000000000, 3.602774393244745134E-13 ) ) ;
#63683=CARTESIAN_POINT ( 'NONE',  ( -90.31319802837603561, 90.93089219781636245, -76.80574412431033693 ) ) ;
#63709=EDGE_CURVE ( 'NONE', #86064, #46578, #14234, .T. ) ;
#63713=LINE ( 'NONE', #28743, #73011 ) ;
#63718=CARTESIAN_POINT ( 'NONE',  ( -4.481506956522084195, 70.65969245518890318, 130.4796279538066983 ) ) ;
#63736=EDGE_CURVE ( 'NONE', #53446, #19496, #10127, .T. ) ;
#63746=DIRECTION ( 'NONE',  ( 0.000000000000000000, 0.000000000000000000, 1.000000000000000000 ) ) ;
#63771=LINE ( 'NONE', #3327, #26550 ) ;
#63772=( GEOMETRIC_REPRESENTATION_CONTEXT ( 3 ) GLOBAL_UNCERTAINTY_ASSIGNED_CONTEXT ( ( #19043 ) ) GLOBAL_UNIT_ASSIGNED_CONTEXT ( ( #73666, #11449, #74563 ) ) REPRESENTATION_CONTEXT ( 'NONE', 'WORKASPACE' ) );
#63775=CARTESIAN_POINT ( 'NONE',  ( -78.94931995840738637, 71.76236341258000095, 88.44575049335577432 ) ) ;
#63776=DIRECTION ( 'NONE',  ( 0.000000000000000000, 1.000000000000000000, 0.000000000000000000 ) ) ;
#63795=ORIENTED_EDGE ( 'NONE', *, *, #89626, .T. ) ;
#63796=CARTESIAN_POINT ( 'NONE',  ( -2.684158038187649039E-15, 69.84999999999999432, 130.5560000000000116 ) ) ;
#63797=LINE ( 'NONE', #7487, #66463 ) ;
#63799=DIRECTION ( 'NONE',  ( 0.000000000000000000, 0.000000000000000000, 1.000000000000000000 ) ) ;
#63814=CARTESIAN_POINT ( 'NONE',  ( 105.4788588808462038, 127.0000000000000000, -3.968749999999580336 ) ) ;
#63816=VECTOR ( 'NONE', #61054, 1000.000000000000000 ) ;
#63821=EDGE_LOOP ( 'NONE', ( #17576, #44225 ) ) ;
#63838=ORIENTED_EDGE ( 'NONE', *, *, #58524, .F. ) ;
#63840=ORIENTED_EDGE ( 'NONE', *, *, #10823, .T. ) ;
#63882=AXIS2_PLACEMENT_3D ( 'NONE', #32151, #33051, #5357 ) ;
#63900=CARTESIAN_POINT ( 'NONE',  ( 99.78216974382816318, 88.91243380484081626, 84.19383299529444287 ) ) ;
#63930=ORIENTED_EDGE ( 'NONE', *, *, #40677, .T. ) ;
#63946=CARTESIAN_POINT ( 'NONE',  ( -3.175000000000109956, 124.5870000000000033, 31.75000000000000000 ) ) ;
#63980=VECTOR ( 'NONE', #45407, 1000.000000000000000 ) ;
#63984=DIRECTION ( 'NONE',  ( -3.278217592397115468E-15, 0.000000000000000000, 1.000000000000000000 ) ) ;
#63989=CARTESIAN_POINT ( 'NONE',  ( 74.36911441044604487, 82.54999999999999716, 92.32962665258637003 ) ) ;
#64004=ORIENTED_EDGE ( 'NONE', *, *, #56517, .F. ) ;
#64009=VERTEX_POINT ( 'NONE', #46155 ) ;
#64010=CARTESIAN_POINT ( 'NONE',  ( -84.41404664249371592, 95.23005795263748041, 83.24642779537488479 ) ) ;
#64015=CYLINDRICAL_SURFACE ( 'NONE', #36011, 7.937500000000000000 ) ;
#64021=VERTEX_POINT ( 'NONE', #10755 ) ;
#64030=CARTESIAN_POINT ( 'NONE',  ( 74.15067561874209900, 127.0000000000000000, 68.53801554307469246 ) ) ;
#64056=AXIS2_PLACEMENT_3D ( 'NONE', #88213, #87744, #25514 ) ;
#64068=CARTESIAN_POINT ( 'NONE',  ( -7.195828152521259823E-13, 127.0000000000000000, 95.25000000000000000 ) ) ;
#64077=VECTOR ( 'NONE', #84914, 1000.000000000000000 ) ;
#64086=CARTESIAN_POINT ( 'NONE',  ( 0.000000000000000000, 125.7300000000000040, 0.000000000000000000 ) ) ;
#64090=CIRCLE ( 'NONE', #35138, 7.937500000000000000 ) ;
#64093=EDGE_CURVE ( 'NONE', #58666, #12205, #65721, .T. ) ;
#64097=CARTESIAN_POINT ( 'NONE',  ( -72.96458098368600531, 117.4749999999999943, -72.96458098368781009 ) ) ;
#64101=LINE ( 'NONE', #27773, #68820 ) ;
#64107=VERTEX_POINT ( 'NONE', #30330 ) ;
#64113=LINE ( 'NONE', #34598, #10849 ) ;
#64118=ORIENTED_EDGE ( 'NONE', *, *, #35019, .T. ) ;
#64126=LINE ( 'NONE', #3678, #10168 ) ;
#64133=CARTESIAN_POINT ( 'NONE',  ( -82.89895571708225930, 82.54999999999999716, -100.8594679592215471 ) ) ;
#64134=CARTESIAN_POINT ( 'NONE',  ( -90.13147184857913885, 91.23868085022583330, -77.01901799881255783 ) ) ;
#64137=AXIS2_PLACEMENT_3D ( 'NONE', #20411, #40390, #5888 ) ;
#64146=EDGE_CURVE ( 'NONE', #37208, #5947, #79583, .T. ) ;
#64147=VERTEX_POINT ( 'NONE', #80717 ) ;
#64193=CARTESIAN_POINT ( 'NONE',  ( -12.05184652617604435, 86.64091671906267322, 129.9989399000961328 ) ) ;
#64208=AXIS2_PLACEMENT_3D ( 'NONE', #34660, #68743, #13776 ) ;
#64220=LINE ( 'NONE', #42403, #35610 ) ;
#64242=CARTESIAN_POINT ( 'NONE',  ( -100.3414980266874039, 87.03008507238371294, -83.52531662946658741 ) ) ;
#64258=EDGE_LOOP ( 'NONE', ( #1501, #6987 ) ) ;
#64269=ORIENTED_EDGE ( 'NONE', *, *, #56985, .F. ) ;
#64287=LINE ( 'NONE', #36123, #65612 ) ;
#64297=DIRECTION ( 'NONE',  ( 0.000000000000000000, 1.000000000000000000, 0.000000000000000000 ) ) ;
#64345=CARTESIAN_POINT ( 'NONE',  ( 86.19814306825382744, 92.12504059357189590, 98.05663017059126219 ) ) ;
#64347=DIRECTION ( 'NONE',  ( 0.000000000000000000, 0.000000000000000000, -1.000000000000000000 ) ) ;
#64373=ORIENTED_EDGE ( 'NONE', *, *, #79929, .F. ) ;
#64374=ORIENTED_EDGE ( 'NONE', *, *, #7102, .T. ) ;
#64386=FACE_BOUND ( 'NONE', #27438, .T. ) ;
#64406=CARTESIAN_POINT ( 'NONE',  ( -3.175000000000120171, 124.5870000000000033, 33.98325472291460159 ) ) ;
#64421=EDGE_CURVE ( 'NONE', #75590, #65492, #89761, .T. ) ;
#64426=VERTEX_POINT ( 'NONE', #711 ) ;
#64446=VERTEX_POINT ( 'NONE', #84311 ) ;
#64447=CARTESIAN_POINT ( 'NONE',  ( 78.00648098368650096, 117.4749999999999943, 72.96458098368729850 ) ) ;
#64450=CARTESIAN_POINT ( 'NONE',  ( -89.13001032377158594, 92.64969027323469675, 78.17826422383558338 ) ) ;
#64452=AXIS2_PLACEMENT_3D ( 'NONE', #58585, #86320, #24097 ) ;
#64484=ORIENTED_EDGE ( 'NONE', *, *, #35960, .T. ) ;
#64488=CARTESIAN_POINT ( 'NONE',  ( 72.96458098368650269, 117.4749999999999943, 72.96458098368729850 ) ) ;
#64510=CARTESIAN_POINT ( 'NONE',  ( -69.72411017813060141, 120.6499999999999915, 69.72411017812929401 ) ) ;
#64514=ORIENTED_EDGE ( 'NONE', *, *, #11965, .T. ) ;
#64518=B_SPLINE_CURVE_WITH_KNOTS ( 'NONE', 3,
 ( #1064, #21975, #29226, #36490, #85097, #42822, #64193, #70559, #8331, #76924, #1967, #7429, #15601, #35119, #607, #71465, #43728, #28304, #70103, #36030, #55996, #10456, #49189, #42374, #56912, #22867 ),
 .UNSPECIFIED., .F., .F.,
 ( 4, 2, 2, 2, 2, 2, 2, 2, 2, 2, 2, 2, 4 ),
 ( 0.01986933033599076748, 0.02111058882927465200, 0.02235184732255853651, 0.02483436430912634718, 0.02607562280241026986, 0.02731688129569419254, 0.02979939828226201015, 0.03228191526882982776, 0.03352317376211373656, 0.03476443225539763843, 0.03724694924196543522, 0.03848820773524934402, 0.03972946622853323895 ),
 .UNSPECIFIED. ) ;
#64521=DIRECTION ( 'NONE',  ( 0.000000000000000000, 1.000000000000000000, 0.000000000000000000 ) ) ;
#64573=CARTESIAN_POINT ( 'NONE',  ( 72.96458098368701428, 127.0000000000000000, -72.96458098368670164 ) ) ;
#64665=EDGE_CURVE ( 'NONE', #23593, #23091, #15140, .T. ) ;
#64688=AXIS2_PLACEMENT_3D ( 'NONE', #53738, #88314, #40128 ) ;
#64702=EDGE_CURVE ( 'NONE', #7755, #28641, #35114, .T. ) ;
#64706=CARTESIAN_POINT ( 'NONE',  ( 3.175000000000334666, 104.3431970271541616, -31.75000000000000000 ) ) ;
#64767=CARTESIAN_POINT ( 'NONE',  ( -11.41209158312316774, 88.18445188672595236, -130.0566639163490095 ) ) ;
#64768=ORIENTED_EDGE ( 'NONE', *, *, #57810, .T. ) ;
#64770=DIRECTION ( 'NONE',  ( 0.000000000000000000, 1.000000000000000000, 0.000000000000000000 ) ) ;
#64788=CARTESIAN_POINT ( 'NONE',  ( 78.95116244206022316, 93.33902940301967988, 88.44409384119040851 ) ) ;
#64825=PLANE ( 'NONE',  #61916 ) ;
#64829=FACE_BOUND ( 'NONE', #42872, .T. ) ;
#64851=DIRECTION ( 'NONE',  ( -1.000000000000000000, 0.000000000000000000, 1.046082768126375896E-16 ) ) ;
#64880=CARTESIAN_POINT ( 'NONE',  ( 79.74945239053440105, 71.14137858619484689, 87.72765544449677577 ) ) ;
#64886=VERTEX_POINT ( 'NONE', #24190 ) ;
#64898=DIRECTION ( 'NONE',  ( -0.9659258262890706437, 0.000000000000000000, 0.2588190451025119132 ) ) ;
#64909=EDGE_LOOP ( 'NONE', ( #75901, #79700 ) ) ;
#64927=ORIENTED_EDGE ( 'NONE', *, *, #14262, .T. ) ;
#64941=VECTOR ( 'NONE', #35774, 1000.000000000000000 ) ;
#64944=AXIS2_PLACEMENT_3D ( 'NONE', #40959, #20539, #21432 ) ;
#64951=DIRECTION ( 'NONE',  ( 0.000000000000000000, 1.000000000000000000, 0.000000000000000000 ) ) ;
#64976=EDGE_CURVE ( 'NONE', #53519, #24962, #45935, .T. ) ;
#64986=DIRECTION ( 'NONE',  ( 0.000000000000000000, 1.000000000000000000, 0.000000000000000000 ) ) ;
#65006=ORIENTED_EDGE ( 'NONE', *, *, #44854, .T. ) ;
#65010=CARTESIAN_POINT ( 'NONE',  ( -87.71605664018947834, 93.55484823631826430, 96.70003673985476667 ) ) ;
#65047=VECTOR ( 'NONE', #21537, 1000.000000000000000 ) ;
#65058=CARTESIAN_POINT ( 'NONE',  ( -1.665555919329872792, 69.93248702128259708, 130.5479027315182066 ) ) ;
#65102=EDGE_CURVE ( 'NONE', #32236, #34136, #23118, .T. ) ;
#65117=CARTESIAN_POINT ( 'NONE',  ( 118.1052048222230724, 75.15251084995277608, -10.33146714902655816 ) ) ;
#65121=CARTESIAN_POINT ( 'NONE',  ( 0.000000000000000000, 127.0000000000000000, -188.9759999999999991 ) ) ;
#65163=CARTESIAN_POINT ( 'NONE',  ( -130.2063869749194964, 74.16976894168006140, 9.551794474071689578 ) ) ;
#65182=CARTESIAN_POINT ( 'NONE',  ( -72.96458098368600531, 127.0000000000000000, -80.10833098368780725 ) ) ;
#65212=CARTESIAN_POINT ( 'NONE',  ( -9.549815870737166534, 90.93248498521381862, -130.2065322450556550 ) ) ;
#65237=CIRCLE ( 'NONE', #46398, 7.143750000000004263 ) ;
#65238=CARTESIAN_POINT ( 'NONE',  ( 6.710386649963810513, 93.34051461951031570, 130.3838978039176482 ) ) ;
#65279=FACE_OUTER_BOUND ( 'NONE', #43419, .T. ) ;
#65302=CARTESIAN_POINT ( 'NONE',  ( -72.96458098368751166, 127.0000000000000000, 72.96458098368620426 ) ) ;
#65321=VERTEX_POINT ( 'NONE', #53743 ) ;
#65324=CARTESIAN_POINT ( 'NONE',  ( 91.51265874544223777, 76.91656954603719498, 75.37281393334542656 ) ) ;
#65330=ORIENTED_EDGE ( 'NONE', *, *, #4655, .F. ) ;
#65335=FACE_OUTER_BOUND ( 'NONE', #48079, .T. ) ;
#65336=CARTESIAN_POINT ( 'NONE',  ( -68.91674821478457602, 82.54999999999999716, 68.91674821478434865 ) ) ;
#65340=VERTEX_POINT ( 'NONE', #85448 ) ;
#65349=DIRECTION ( 'NONE',  ( 0.000000000000000000, -1.000000000000000000, 0.000000000000000000 ) ) ;
#65372=EDGE_CURVE ( 'NONE', #73425, #64021, #30457, .T. ) ;
#65379=CARTESIAN_POINT ( 'NONE',  ( 72.96458098368650269, 127.0000000000000000, 72.96458098368729850 ) ) ;
#65381=FACE_OUTER_BOUND ( 'NONE', #78859, .T. ) ;
#65383=DIRECTION ( 'NONE',  ( 0.000000000000000000, 0.000000000000000000, -1.000000000000000000 ) ) ;
#65396=EDGE_CURVE ( 'NONE', #66271, #84986, #71020, .T. ) ;
#65425=CARTESIAN_POINT ( 'NONE',  ( 100.8594679592218171, 82.96445444011519044, -82.89895571708193245 ) ) ;
#65465=CARTESIAN_POINT ( 'NONE',  ( -3.175000000000109956, 111.1250000000000000, 31.75000000000000000 ) ) ;
#65470=LINE ( 'NONE', #58209, #21026 ) ;
#65479=ADVANCED_FACE ( 'NONE', ( #68442 ), #75258, .F. ) ;
#65491=AXIS2_PLACEMENT_3D ( 'NONE', #13467, #88888, #27096 ) ;
#65492=VERTEX_POINT ( 'NONE', #53878 ) ;
#65502=CARTESIAN_POINT ( 'NONE',  ( -10.79079172156231081, 75.84006377869074811, 130.1095006741098530 ) ) ;
#65510=PLANE ( 'NONE',  #75597 ) ;
#65531=CYLINDRICAL_SURFACE ( 'NONE', #15135, 190.5000000000000000 ) ;
#65548=VECTOR ( 'NONE', #58512, 1000.000000000000000 ) ;
#65564=CARTESIAN_POINT ( 'NONE',  ( 118.5214325610856605, 70.17658267799284033, -2.892017926149469620 ) ) ;
#65599=ORIENTED_EDGE ( 'NONE', *, *, #63143, .F. ) ;
#65609=CARTESIAN_POINT ( 'NONE',  ( -130.1093520674644139, 75.84295037288958952, -10.79257909650410951 ) ) ;
#65612=VECTOR ( 'NONE', #30206, 1000.000000000000000 ) ;
#65614=VERTEX_POINT ( 'NONE', #78409 ) ;
#65640=CARTESIAN_POINT ( 'NONE',  ( 100.8961411191535973, 127.0000000000000000, -3.968749999999580336 ) ) ;
#65643=EDGE_CURVE ( 'NONE', #89346, #66826, #49320, .T. ) ;
#65651=DIRECTION ( 'NONE',  ( -0.9659258262890706437, 0.000000000000000000, 0.2588190451025119132 ) ) ;
#65655=ORIENTED_EDGE ( 'NONE', *, *, #83984, .F. ) ;
#65663=DIRECTION ( 'NONE',  ( 0.000000000000000000, 1.000000000000000000, 0.000000000000000000 ) ) ;
#65666=CARTESIAN_POINT ( 'NONE',  ( 76.79137032886029601, 90.93965867633433220, 90.32698471909210980 ) ) ;
#65708=FACE_BOUND ( 'NONE', #79715, .T. ) ;
#65721=LINE ( 'NONE', #11207, #20112 ) ;
#65726=DIRECTION ( 'NONE',  ( 1.000000000000000000, 0.000000000000000000, 0.000000000000000000 ) ) ;
#65736=CARTESIAN_POINT ( 'NONE',  ( 9.572882853229341293, 90.93765695308120200, -130.2059221945669947 ) ) ;
#65756=EDGE_CURVE ( 'NONE', #28103, #27899, #35698, .T. ) ;
#65762=CARTESIAN_POINT ( 'NONE',  ( 118.0447731586489084, 88.91144712388913263, 10.99980504627958133 ) ) ;
#65765=DIRECTION ( 'NONE',  ( 0.7071067811865461294, 0.000000000000000000, 0.7071067811865489050 ) ) ;
#65779=CARTESIAN_POINT ( 'NONE',  ( 92.12462914090806976, 79.66725693986900581, -74.62294912200620445 ) ) ;
#65783=EDGE_CURVE ( 'NONE', #14127, #24560, #72507, .T. ) ;
#65801=ORIENTED_EDGE ( 'NONE', *, *, #60537, .F. ) ;
#65876=LINE ( 'NONE', #46761, #35607 ) ;
#65881=CIRCLE ( 'NONE', #54253, 7.143750000000004263 ) ;
#65885=CARTESIAN_POINT ( 'NONE',  ( -100.1374281256141217, 87.79544278253753475, 83.76986456925436642 ) ) ;
#65889=DIRECTION ( 'NONE',  ( 0.000000000000000000, 0.000000000000000000, 1.000000000000000000 ) ) ;
#65891=ORIENTED_EDGE ( 'NONE', *, *, #78627, .F. ) ;
#65913=DIRECTION ( 'NONE',  ( 0.000000000000000000, 0.000000000000000000, 1.000000000000000000 ) ) ;
#65922=EDGE_LOOP ( 'NONE', ( #67953, #27595 ) ) ;
#65934=CARTESIAN_POINT ( 'NONE',  ( -90.65754775987979031, 74.81620433377383961, -76.39898589339183843 ) ) ;
#65969=EDGE_CURVE ( 'NONE', #27146, #52484, #87027, .T. ) ;
#65981=EDGE_CURVE ( 'NONE', #30848, #26828, #40614, .T. ) ;
#65982=CARTESIAN_POINT ( 'NONE',  ( -83.41556370846475943, 78.46683822717000112, 100.4327019155588090 ) ) ;
#65991=LINE ( 'NONE', #16970, #28828 ) ;
#65995=CARTESIAN_POINT ( 'NONE',  ( 118.3250318368774856, 72.22378176823140450, 7.404816947595408649 ) ) ;
#66017=CARTESIAN_POINT ( 'NONE',  ( -6.364907348149458244, 71.52879593750107290, 118.3870396030140029 ) ) ;
#66031=EDGE_LOOP ( 'NONE', ( #61712, #54588, #10607, #76036 ) ) ;
#66032=ORIENTED_EDGE ( 'NONE', *, *, #13872, .T. ) ;
#66045=EDGE_CURVE ( 'NONE', #12494, #71312, #65237, .T. ) ;
#66054=B_SPLINE_CURVE_WITH_KNOTS ( 'NONE', 3,
 ( #46747, #11809, #53999, #13154, #26760, #66760, #74479, #80408, #5443, #53552, #53094, #67664, #4546, #59931, #81757, #33139, #19508, #68563, #40835, #11353, #18615, #47190, #25425, #74930, #68113 ),
 .UNSPECIFIED., .F., .F.,
 ( 4, 2, 2, 2, 2, 2, 2, 2, 2, 1, 2, 2, 4 ),
 ( 0.05960646776571127542, 0.06208810814592213845, 0.06332892833602757343, 0.06456974852613300841, 0.06705138890634392002, 0.06829220909644936888, 0.06953302928655483162, 0.07201466966676572934, 0.07325548985687117820, 0.07449631004697662706, 0.07573713023708206205, 0.07697795042718751091, 0.07945959080739838087 ),
 .UNSPECIFIED. ) ;
#66077=CIRCLE ( 'NONE', #58814, 24.63800000000000168 ) ;
#66103=DIRECTION ( 'NONE',  ( 0.000000000000000000, 0.000000000000000000, 1.000000000000000000 ) ) ;
#66104=CIRCLE ( 'NONE', #57419, 7.937500000000000000 ) ;
#66106=CARTESIAN_POINT ( 'NONE',  ( 5.635138049808393390, 71.13823012824934722, -130.4366002064613212 ) ) ;
#66179=CARTESIAN_POINT ( 'NONE',  ( 3.175000000000334666, 104.3431970271541616, -31.75000000000000000 ) ) ;
#66191=ADVANCED_FACE ( 'NONE', ( #15612 ), #56922, .F. ) ;
#66196=VERTEX_POINT ( 'NONE', #71025 ) ;
#66207=CARTESIAN_POINT ( 'NONE',  ( 118.1262036371151680, 90.29828471680512791, 10.09645181158910354 ) ) ;
#66216=DIRECTION ( 'NONE',  ( 0.000000000000000000, 1.000000000000000000, 0.000000000000000000 ) ) ;
#66240=CARTESIAN_POINT ( 'NONE',  ( -118.0058494126929389, 76.91656954603718077, 11.41259371393320521 ) ) ;
#66250=FACE_OUTER_BOUND ( 'NONE', #14517, .T. ) ;
#66251=VERTEX_POINT ( 'NONE', #70114 ) ;
#66271=VERTEX_POINT ( 'NONE', #49652 ) ;
#66276=CARTESIAN_POINT ( 'NONE',  ( 4.163101094985349692E-14, 127.0000000000000000, -98.60478223830740774 ) ) ;
#66303=DIRECTION ( 'NONE',  ( 0.000000000000000000, -1.000000000000000000, 0.000000000000000000 ) ) ;
#66304=CARTESIAN_POINT ( 'NONE',  ( 72.96458098368650269, 117.4749999999999943, 65.02708098368729850 ) ) ;
#66321=DIRECTION ( 'NONE',  ( 0.000000000000000000, 0.000000000000000000, 1.000000000000000000 ) ) ;
#66331=CARTESIAN_POINT ( 'NONE',  ( -118.5472366675172253, 95.16897323824362331, 1.658320819117713674 ) ) ;
#66333=CARTESIAN_POINT ( 'NONE',  ( 0.000000000000000000, 127.0000000000000000, -103.1875000000000000 ) ) ;
#66340=ORIENTED_EDGE ( 'NONE', *, *, #50738, .T. ) ;
#66378=ORIENTED_EDGE ( 'NONE', *, *, #61559, .T. ) ;
#66389=EDGE_CURVE ( 'NONE', #5020, #16533, #13111, .T. ) ;
#66398=DIRECTION ( 'NONE',  ( 0.000000000000000000, 1.000000000000000000, 0.000000000000000000 ) ) ;
#66401=AXIS2_PLACEMENT_3D ( 'NONE', #53807, #61532, #19321 ) ;
#66410=AXIS2_PLACEMENT_3D ( 'NONE', #28184, #89090, #13673 ) ;
#66424=FACE_OUTER_BOUND ( 'NONE', #48595, .T. ) ;
#66430=CARTESIAN_POINT ( 'NONE',  ( -84.72210942531908984, 75.15271101351805783, 99.33321048326511971 ) ) ;
#66443=CARTESIAN_POINT ( 'NONE',  ( 117.8825533107838908, 80.89685143461888117, 12.61964884581579049 ) ) ;
#66453=FACE_OUTER_BOUND ( 'NONE', #46760, .T. ) ;
#66462=ORIENTED_EDGE ( 'NONE', *, *, #56252, .F. ) ;
#66463=VECTOR ( 'NONE', #9275, 1000.000000000000000 ) ;
#66471=AXIS2_PLACEMENT_3D ( 'NONE', #28931, #56617, #42974 ) ;
#66483=ADVANCED_FACE ( 'NONE', ( #60946 ), #74140, .F. ) ;
#66515=DIRECTION ( 'NONE',  ( 0.000000000000000000, -1.000000000000000000, 0.000000000000000000 ) ) ;
#66548=EDGE_LOOP ( 'NONE', ( #11413, #15212, #45421, #15784 ) ) ;
#66550=ORIENTED_EDGE ( 'NONE', *, *, #21948, .F. ) ;
#66591=EDGE_CURVE ( 'NONE', #66826, #67802, #62439, .T. ) ;
#66603=ORIENTED_EDGE ( 'NONE', *, *, #12488, .F. ) ;
#66615=CARTESIAN_POINT ( 'NONE',  ( 0.000000000000000000, 127.0000000000000000, -95.25000000000000000 ) ) ;
#66634=CARTESIAN_POINT ( 'NONE',  ( -3.175000000000109956, 124.5870000000000033, 31.75000000000000000 ) ) ;
#66635=CARTESIAN_POINT ( 'NONE',  ( 12.53577546185475988, 84.62767492864718122, -129.9527996235914884 ) ) ;
#66650=DIRECTION ( 'NONE',  ( 0.000000000000000000, 1.000000000000000000, 0.000000000000000000 ) ) ;
#66652=EDGE_CURVE ( 'NONE', #32905, #23593, #513, .T. ) ;
#66699=CARTESIAN_POINT ( 'NONE',  ( -118.3867465934798702, 71.53193882405243187, -6.370299515174613347 ) ) ;
#66703=VECTOR ( 'NONE', #3785, 1000.000000000000000 ) ;
#66705=ORIENTED_EDGE ( 'NONE', *, *, #17540, .F. ) ;
#66726=DIRECTION ( 'NONE',  ( -1.000000000000000000, 0.000000000000000000, 0.000000000000000000 ) ) ;
#66738=CARTESIAN_POINT ( 'NONE',  ( 103.1875000000000000, 120.6499999999999915, 7.937500000000369482 ) ) ;
#66739=ORIENTED_EDGE ( 'NONE', *, *, #78329, .T. ) ;
#66745=CARTESIAN_POINT ( 'NONE',  ( -129.9368274816650626, 82.54999999999999716, -12.70000000000045404 ) ) ;
#66746=DIRECTION ( 'NONE',  ( 0.000000000000000000, 0.000000000000000000, 1.000000000000000000 ) ) ;
#66760=CARTESIAN_POINT ( 'NONE',  ( -12.03342778677654934, 78.46830267626332045, -117.9437853765525404 ) ) ;
#66769=AXIS2_PLACEMENT_3D ( 'NONE', #80432, #66783, #74049 ) ;
#66783=DIRECTION ( 'NONE',  ( -0.000000000000000000, 1.000000000000000000, 0.000000000000000000 ) ) ;
#66793=VERTEX_POINT ( 'NONE', #66304 ) ;
#66805=DIRECTION ( 'NONE',  ( 0.000000000000000000, 1.000000000000000000, 0.000000000000000000 ) ) ;
#66806=ADVANCED_FACE ( 'NONE', ( #24106 ), #23666, .F. ) ;
#66812=CARTESIAN_POINT ( 'NONE',  ( 103.1875000000000000, 127.0000000000000000, -7.143749999999640110 ) ) ;
#66820=CARTESIAN_POINT ( 'NONE',  ( 130.4924867222204341, 94.58014758961630264, -4.091264198875782299 ) ) ;
#66822=VECTOR ( 'NONE', #10385, 1000.000000000000000 ) ;
#66826=VERTEX_POINT ( 'NONE', #4091 ) ;
#66848=VECTOR ( 'NONE', #70787, 1000.000000000000000 ) ;
#66853=SHAPE_REPRESENTATION_RELATIONSHIP ( 'NONE' , 'NONE' ,  #42769, #43438 ) ;
#66861=CYLINDRICAL_SURFACE ( 'NONE', #8087, 5.041900000000001825 ) ;
#66885=VECTOR ( 'NONE', #31424, 1000.000000000000227 ) ;
#66899=FACE_OUTER_BOUND ( 'NONE', #87373, .T. ) ;
#66900=CARTESIAN_POINT ( 'NONE',  ( -72.96458098368600531, 117.4749999999999943, -80.10833098368780725 ) ) ;
#66910=CARTESIAN_POINT ( 'NONE',  ( 33.98325472291465132, 124.5870000000000033, -3.174999999999999822 ) ) ;
#66912=VECTOR ( 'NONE', #20294, 1000.000000000000000 ) ;
#66916=CARTESIAN_POINT ( 'NONE',  ( -7.205548786489490269E-13, 117.4749999999999943, 103.1875000000000000 ) ) ;
#66958=CYLINDRICAL_SURFACE ( 'NONE', #83373, 7.143750000000004263 ) ;
#66977=LINE ( 'NONE', #25640, #6864 ) ;
#66981=VECTOR ( 'NONE', #16053, 1000.000000000000000 ) ;
#66984=ORIENTED_EDGE ( 'NONE', *, *, #14724, .T. ) ;
#67004=DIRECTION ( 'NONE',  ( 0.000000000000000000, 0.000000000000000000, 1.000000000000000000 ) ) ;
#67008=CARTESIAN_POINT ( 'NONE',  ( -100.8961411191535973, 120.6499999999999915, -3.968750000001104894 ) ) ;
#67016=CARTESIAN_POINT ( 'NONE',  ( 10.08079905861141867, 90.28579524239225407, 130.1664991954059474 ) ) ;
#67024=CARTESIAN_POINT ( 'NONE',  ( -68.53801554307499089, 120.6499999999999915, 74.15067561874188584 ) ) ;
#67068=PLANE ( 'NONE',  #41185 ) ;
#67072=CARTESIAN_POINT ( 'NONE',  ( 2.332952152375709937E-14, 125.4759999999999991, 190.5000000000000000 ) ) ;
#67094=VERTEX_POINT ( 'NONE', #27668 ) ;
#67101=CARTESIAN_POINT ( 'NONE',  ( 69.72411017812960665, 120.6499999999999915, 69.72411017813040246 ) ) ;
#67106=ORIENTED_EDGE ( 'NONE', *, *, #19166, .T. ) ;
#67115=CARTESIAN_POINT ( 'NONE',  ( 117.8914297010764756, 84.62843115047675724, 12.53565398905701578 ) ) ;
#67147=CARTESIAN_POINT ( 'NONE',  ( -117.8738102209308494, 81.71068249639866110, 12.69999999999959250 ) ) ;
#67154=CARTESIAN_POINT ( 'NONE',  ( 0.000000000000000000, 95.25000000000000000, 0.000000000000000000 ) ) ;
#67161=ORIENTED_EDGE ( 'NONE', *, *, #52274, .F. ) ;
#67187=CARTESIAN_POINT ( 'NONE',  ( -130.5559693845970060, 95.24968527363473925, 0.8339068267398820344 ) ) ;
#67200=CARTESIAN_POINT ( 'NONE',  ( 77.39114642429960611, 120.6499999999999915, -71.77848634863110533 ) ) ;
#67201=DIRECTION ( 'NONE',  ( 0.000000000000000000, 1.000000000000000000, 0.000000000000000000 ) ) ;
#67203=DIRECTION ( 'NONE',  ( 0.000000000000000000, 0.000000000000000000, -1.000000000000000000 ) ) ;
#67228=CARTESIAN_POINT ( 'NONE',  ( -117.8738102209307215, 82.54999999999999716, -12.70000000000041318 ) ) ;
#67252=VECTOR ( 'NONE', #25315, 1000.000000000000000 ) ;
#67254=ORIENTED_EDGE ( 'NONE', *, *, #43934, .T. ) ;
#67264=PRESENTATION_STYLE_ASSIGNMENT (( #88187 ) ) ;
#67279=CARTESIAN_POINT ( 'NONE',  ( 0.000000000000000000, 127.0000000000000000, 0.000000000000000000 ) ) ;
#67281=CARTESIAN_POINT ( 'NONE',  ( -92.32962665258511947, 81.71068249639866110, -74.36911441044765070 ) ) ;
#67290=ORIENTED_EDGE ( 'NONE', *, *, #85286, .T. ) ;
#67336=DIRECTION ( 'NONE',  ( 0.000000000000000000, 0.000000000000000000, -1.000000000000000000 ) ) ;
#67340=PLANE ( 'NONE',  #35891 ) ;
#67343=CARTESIAN_POINT ( 'NONE',  ( -89.37861919290428148, 70.52006616879377532, -95.16559702356661887 ) ) ;
#67348=CARTESIAN_POINT ( 'NONE',  ( 4.163101094985349692E-14, 127.0000000000000000, -98.60478223830740774 ) ) ;
#67363=DIRECTION ( 'NONE',  ( 0.2588190451025131344, 0.000000000000000000, 0.9659258262890704216 ) ) ;
#67367=VECTOR ( 'NONE', #29813, 1000.000000000000000 ) ;
#67373=CARTESIAN_POINT ( 'NONE',  ( 72.96458098368650269, 127.0000000000000000, 72.96458098368729850 ) ) ;
#67394=DIRECTION ( 'NONE',  ( 0.000000000000000000, 0.000000000000000000, 1.000000000000000000 ) ) ;
#67398=CARTESIAN_POINT ( 'NONE',  ( 72.96458098368650269, 117.4749999999999943, 72.96458098368729850 ) ) ;
#67423=EDGE_CURVE ( 'NONE', #49178, #24254, #11241, .T. ) ;
#67429=CARTESIAN_POINT ( 'NONE',  ( 72.96458098368701428, 127.0000000000000000, -72.96458098368670164 ) ) ;
#67433=EDGE_CURVE ( 'NONE', #25068, #20813, #25765, .T. ) ;
#67446=LINE ( 'NONE', #33379, #73740 ) ;
#67449=CARTESIAN_POINT ( 'NONE',  ( 12.03144885753538595, 78.46257116061715919, -130.0004926519013111 ) ) ;
#67484=ORIENTED_EDGE ( 'NONE', *, *, #8787, .F. ) ;
#67493=EDGE_LOOP ( 'NONE', ( #43182, #52553 ) ) ;
#67505=CIRCLE ( 'NONE', #76202, 7.937500000000000000 ) ;
#67531=CARTESIAN_POINT ( 'NONE',  ( 12.05184652617604613, 86.64091671906268743, -129.9989399000961612 ) ) ;
#67534=LINE ( 'NONE', #5321, #37061 ) ;
#67558=ORIENTED_EDGE ( 'NONE', *, *, #51810, .F. ) ;
#67562=CARTESIAN_POINT ( 'NONE',  ( -69.72411017812909506, 120.6499999999999915, -69.72411017813089984 ) ) ;
#67611=ORIENTED_EDGE ( 'NONE', *, *, #13689, .T. ) ;
#67636=ORIENTED_EDGE ( 'NONE', *, *, #28024, .T. ) ;
#67637=DIRECTION ( 'NONE',  ( 0.000000000000000000, 0.000000000000000000, 1.000000000000000000 ) ) ;
#67643=CARTESIAN_POINT ( 'NONE',  ( -130.5169520046879086, 94.84315624882769669, -3.295103719954349142 ) ) ;
#67646=VECTOR ( 'NONE', #49573, 1000.000000000000000 ) ;
#67648=EDGE_CURVE ( 'NONE', #9719, #5415, #13938, .T. ) ;
#67654=FACE_OUTER_BOUND ( 'NONE', #9183, .T. ) ;
#67657=ORIENTED_EDGE ( 'NONE', *, *, #46799, .F. ) ;
#67660=CARTESIAN_POINT ( 'NONE',  ( 83.22850972642787326, 85.83513192049075258, -100.5877680347017957 ) ) ;
#67664=CARTESIAN_POINT ( 'NONE',  ( -9.554550254943340093, 74.17292945273928240, -118.1706666865833455 ) ) ;
#67675=CARTESIAN_POINT ( 'NONE',  ( 82.89895571708156297, 82.54999999999999716, 100.8594679592221155 ) ) ;
#67685=CARTESIAN_POINT ( 'NONE',  ( -118.3048154812336321, 92.64969027323465411, -7.744053933098289377 ) ) ;
#67690=FACE_OUTER_BOUND ( 'NONE', #27436, .T. ) ;
#67714=DIRECTION ( 'NONE',  ( 1.000000000000000000, 0.000000000000000000, 0.000000000000000000 ) ) ;
#67720=ORIENTED_EDGE ( 'NONE', *, *, #69947, .F. ) ;
#67721=CARTESIAN_POINT ( 'NONE',  ( 130.4942851453020012, 94.60320878023495084, 4.086962795942436166 ) ) ;
#67731=CARTESIAN_POINT ( 'NONE',  ( -12.69999999999999929, 81.71142461540233626, -129.9368274816650626 ) ) ;
#67750=FACE_OUTER_BOUND ( 'NONE', #46952, .T. ) ;
#67802=VERTEX_POINT ( 'NONE', #68297 ) ;
#67828=ORIENTED_EDGE ( 'NONE', *, *, #30435, .T. ) ;
#67845=AXIS2_PLACEMENT_3D ( 'NONE', #64510, #78607, #30437 ) ;
#67847=AXIS2_PLACEMENT_3D ( 'NONE', #5123, #34157, #12849 ) ;
#67874=CARTESIAN_POINT ( 'NONE',  ( -72.96458098368751166, 101.5999999999999943, 67.92268098368620599 ) ) ;
#67889=DIRECTION ( 'NONE',  ( 0.000000000000000000, 0.000000000000000000, -1.000000000000000000 ) ) ;
#67903=CARTESIAN_POINT ( 'NONE',  ( 11.00676631360785862, 76.20068480870281746, -130.0913480697105342 ) ) ;
#67907=CARTESIAN_POINT ( 'NONE',  ( 81.47101467905535799, 94.84303900880917126, 86.13165781700368484 ) ) ;
#67913=DIRECTION ( 'NONE',  ( 0.000000000000000000, 0.000000000000000000, 1.000000000000000000 ) ) ;
#67914=CARTESIAN_POINT ( 'NONE',  ( -84.37439091330328722, 89.26666702275849730, -99.62873342662643950 ) ) ;
#67917=CARTESIAN_POINT ( 'NONE',  ( -76.20505178924449297, 127.0000000000000000, 76.20505178924310030 ) ) ;
#67931=ADVANCED_FACE ( 'NONE', ( #70889 ), #22286, .F. ) ;
#67941=ADVANCED_FACE ( 'NONE', ( #2290 ), #22740, .F. ) ;
#67946=DIRECTION ( 'NONE',  ( 0.7071067811865389130, 0.000000000000000000, 0.7071067811865561215 ) ) ;
#67952=CARTESIAN_POINT ( 'NONE',  ( 129.9681746291969375, 79.66695435136418268, -12.37535028237872226 ) ) ;
#67953=ORIENTED_EDGE ( 'NONE', *, *, #42477, .T. ) ;
#67960=AXIS2_PLACEMENT_3D ( 'NONE', #8736, #15545, #37771 ) ;
#67982=ORIENTED_EDGE ( 'NONE', *, *, #65396, .F. ) ;
#67998=DIRECTION ( 'NONE',  ( 0.000000000000000000, 0.000000000000000000, -1.000000000000000000 ) ) ;
#68005=VERTEX_POINT ( 'NONE', #77248 ) ;
#68012=LINE ( 'NONE', #68468, #5490 ) ;
#68017=FACE_OUTER_BOUND ( 'NONE', #8988, .T. ) ;
#68020=CARTESIAN_POINT ( 'NONE',  ( 100.8961411191535973, 120.6499999999999915, -3.968749999999580336 ) ) ;
#68037=AXIS2_PLACEMENT_3D ( 'NONE', #87351, #25111, #52774 ) ;
#68050=CARTESIAN_POINT ( 'NONE',  ( -117.8738102209307925, 82.54999999999999716, 12.69999999999959073 ) ) ;
#68053=EDGE_CURVE ( 'NONE', #53519, #42410, #21496, .T. ) ;
#68059=CARTESIAN_POINT ( 'NONE',  ( 8.690994986491583418, 73.28026231907210786, -118.2373793989773247 ) ) ;
#68072=CYLINDRICAL_SURFACE ( 'NONE', #31525, 5.041900000000001825 ) ;
#68095=CARTESIAN_POINT ( 'NONE',  ( -130.2877996231769941, 92.12504059357188169, -8.385216644674851949 ) ) ;
#68108=CARTESIAN_POINT ( 'NONE',  ( -7.301849239715819957E-13, 127.0000000000000000, 98.60478223830740774 ) ) ;
#68113=CARTESIAN_POINT ( 'NONE',  ( -6.802569982901797644E-16, 69.84999999999999432, -118.5560000000000116 ) ) ;
#68126=ORIENTED_EDGE ( 'NONE', *, *, #81613, .F. ) ;
#68131=ADVANCED_FACE ( 'NONE', ( #45374, #9991 ), #24072, .F. ) ;
#68134=CARTESIAN_POINT ( 'NONE',  ( -118.5385583271987713, 95.08639429146512612, -2.073938160688237442 ) ) ;
#68149=ADVANCED_FACE ( 'NONE', ( #31306 ), #59002, .F. ) ;
#68173=CARTESIAN_POINT ( 'NONE',  ( 69.72411017813010403, 127.0000000000000000, -69.72411017812979139 ) ) ;
#68179=( NAMED_UNIT ( * ) PLANE_ANGLE_UNIT ( ) SI_UNIT ( $, .RADIAN. ) );
#68185=ORIENTED_EDGE ( 'NONE', *, *, #40134, .T. ) ;
#68188=CARTESIAN_POINT ( 'NONE',  ( -6.720195294977327372, 71.76561749959921599, -130.3833905926466628 ) ) ;
#68242=CARTESIAN_POINT ( 'NONE',  ( -95.16559702356633466, 70.52006616879377532, 89.37861919290460833 ) ) ;
#68250=CARTESIAN_POINT ( 'NONE',  ( 12.70000000000000107, 82.54999999999999716, 117.8738102209307641 ) ) ;
#68258=CARTESIAN_POINT ( 'NONE',  ( -3.174999999999644995, 124.5870000000000033, -33.98325472291465132 ) ) ;
#68290=CARTESIAN_POINT ( 'NONE',  ( 9.549789689180780528, 90.93251752167836344, 118.1710524764279029 ) ) ;
#68297=CARTESIAN_POINT ( 'NONE',  ( 5.210259806972410633E-15, 127.0000000000000000, -42.54500000000000171 ) ) ;
#68322=CARTESIAN_POINT ( 'NONE',  ( -4.868064396069518907, 94.30179516618007085, -118.4578665249601386 ) ) ;
#68330=VECTOR ( 'NONE', #3295, 1000.000000000000000 ) ;
#68333=LINE ( 'NONE', #82873, #3025 ) ;
#68363=CARTESIAN_POINT ( 'NONE',  ( 84.99816483510821286, 95.16897323824359489, 82.65294504194773140 ) ) ;
#68370=AXIS2_PLACEMENT_3D ( 'NONE', #72560, #45272, #58024 ) ;
#68408=ORIENTED_EDGE ( 'NONE', *, *, #87532, .T. ) ;
#68409=CARTESIAN_POINT ( 'NONE',  ( 130.5560612649026950, 69.84937019662270075, -0.8297548318604713868 ) ) ;
#68413=LINE ( 'NONE', #87510, #82277 ) ;
#68426=CARTESIAN_POINT ( 'NONE',  ( 0.000000000000000000, 124.5870000000000033, 0.000000000000000000 ) ) ;
#68431=PLANE ( 'NONE',  #12323 ) ;
#68437=FACE_OUTER_BOUND ( 'NONE', #5887, .T. ) ;
#68442=FACE_OUTER_BOUND ( 'NONE', #30760, .T. ) ;
#68468=CARTESIAN_POINT ( 'NONE',  ( 0.000000000000000000, 61.59999999999999432, 118.5560000000000116 ) ) ;
#68469=CARTESIAN_POINT ( 'NONE',  ( -72.96458098368751166, 127.0000000000000000, 72.96458098368620426 ) ) ;
#68470=CARTESIAN_POINT ( 'NONE',  ( 3.968750000000050182, 120.6499999999999915, -100.8961411191535973 ) ) ;
#68472=EDGE_CURVE ( 'NONE', #8309, #81558, #67446, .T. ) ;
#68492=VECTOR ( 'NONE', #4299, 1000.000000000000000 ) ;
#68496=CARTESIAN_POINT ( 'NONE',  ( -4.090931056105388208, 94.60184303864161848, 118.4878965444427763 ) ) ;
#68504=ORIENTED_EDGE ( 'NONE', *, *, #71708, .T. ) ;
#68505=B_SPLINE_CURVE_WITH_KNOTS ( 'NONE', 3,
 ( #6869, #63179, #49980, #54984, #29115, #48625, #34117, #84090, #15497, #83637, #35013, #504, #49532, #76365, #42712, #957, #82754, #34570, #61820, #89552, #70454, #28197, #84547, #69552, #35916, #1416, #70000, #28656, #49079, #77719, #63630, #76812, #20517, #14138, #43168, #75916, #13684, #41816, #41374, #25749, #87992, #53426, #80733, #59369, #17167, #79403, #86652, #81194 ),
 .UNSPECIFIED., .F., .F.,
 ( 4, 2, 2, 2, 2, 2, 2, 2, 2, 1, 2, 2, 2, 2, 2, 2, 2, 2, 2, 2, 2, 1, 2, 2, 4 ),
 ( 0.05959919981814691681, 0.06208168506169069872, 0.06332292768346259315, 0.06456417030523449452, 0.06704665554877822786, 0.06828789817055011535, 0.06952914079232200284, 0.07201162603586573618, 0.07325286865763760979, 0.07449411127940946953, 0.07573535390118135702, 0.07697659652295323063, 0.07945908176649693622, 0.08194156701004066956, 0.08318280963181254317, 0.08442405225358443066, 0.08690653749712810849, 0.08814778011889994047, 0.08938902274067177245, 0.09187150798421545028, 0.09311275060598728226, 0.09435399322775911424, 0.09559523584953094621, 0.09683647847130277819, 0.09931896371484644215 ),
 .UNSPECIFIED. ) ;
#68514=ORIENTED_EDGE ( 'NONE', *, *, #86349, .T. ) ;
#68517=AXIS2_PLACEMENT_3D ( 'NONE', #29795, #76602, #85228 ) ;
#68541=VERTEX_POINT ( 'NONE', #39301 ) ;
#68543=CARTESIAN_POINT ( 'NONE',  ( -129.9761744276715092, 85.85000629251466364, -12.29186252049120931 ) ) ;
#68544=CARTESIAN_POINT ( 'NONE',  ( 100.8961411191535973, 120.6499999999999915, 3.968750000000400124 ) ) ;
#68556=CARTESIAN_POINT ( 'NONE',  ( 103.1875000000000000, 117.4749999999999943, 5.041900000000359761 ) ) ;
#68557=CARTESIAN_POINT ( 'NONE',  ( 83.15057989155033624, 85.43248893795414745, -100.6521573293560294 ) ) ;
#68563=CARTESIAN_POINT ( 'NONE',  ( -5.627926923415666138, 71.15750911566317427, -118.4229113093306438 ) ) ;
#68592=PLANE ( 'NONE',  #58013 ) ;
#68598=EDGE_CURVE ( 'NONE', #83603, #83684, #77864, .T. ) ;
#68625=CARTESIAN_POINT ( 'NONE',  ( 130.2266700119015752, 91.23859726994547259, -9.271983876140096115 ) ) ;
#68643=CARTESIAN_POINT ( 'NONE',  ( -76.38829385798634064, 74.80137413886474462, -90.66736180499671605 ) ) ;
#68664=CARTESIAN_POINT ( 'NONE',  ( 10.33363185139394957, 75.15554654547490543, 118.1050150300115007 ) ) ;
#68677=CARTESIAN_POINT ( 'NONE',  ( -69.72411017813060141, 120.6499999999999915, 69.72411017812929401 ) ) ;
#68690=EDGE_CURVE ( 'NONE', #87834, #40086, #65991, .T. ) ;
#68695=VECTOR ( 'NONE', #58488, 1000.000000000000000 ) ;
#68706=CARTESIAN_POINT ( 'NONE',  ( -100.0338904447226582, 76.91670260214422683, -83.89393544538330616 ) ) ;
#68711=VECTOR ( 'NONE', #73285, 1000.000000000000000 ) ;
#68731=CARTESIAN_POINT ( 'NONE',  ( 1.145694247088684285E-22, 95.25000000000000000, 118.5560000000000116 ) ) ;
#68743=DIRECTION ( 'NONE',  ( -0.000000000000000000, -0.000000000000000000, 1.000000000000000000 ) ) ;
#68765=AXIS2_PLACEMENT_3D ( 'NONE', #47093, #54347, #40740 ) ;
#68783=VERTEX_POINT ( 'NONE', #37862 ) ;
#68788=ORIENTED_EDGE ( 'NONE', *, *, #84814, .T. ) ;
#68793=CARTESIAN_POINT ( 'NONE',  ( -92.05992619857299530, 79.25941250729452747, 74.70281015415477555 ) ) ;
#68808=DIRECTION ( 'NONE',  ( 0.5000000000000061062, 0.000000000000000000, -0.8660254037844351549 ) ) ;
#68811=VERTEX_POINT ( 'NONE', #73251 ) ;
#68820=VECTOR ( 'NONE', #84103, 1000.000000000000114 ) ;
#68822=VECTOR ( 'NONE', #77929, 1000.000000000000000 ) ;
#68852=CARTESIAN_POINT ( 'NONE',  ( 130.4924045281959764, 70.52074417248461202, -4.093845692692696936 ) ) ;
#68863=DIRECTION ( 'NONE',  ( 0.000000000000000000, -1.000000000000000000, 0.000000000000000000 ) ) ;
#68884=DIRECTION ( 'NONE',  ( 1.000000000000000000, 0.000000000000000000, 6.982966722218760189E-15 ) ) ;
#68891=VECTOR ( 'NONE', #86818, 1000.000000000000114 ) ;
#68912=LINE ( 'NONE', #54803, #4897 ) ;
#68958=ORIENTED_EDGE ( 'NONE', *, *, #9703, .T. ) ;
#68959=VECTOR ( 'NONE', #49285, 1000.000000000000000 ) ;
#68989=CARTESIAN_POINT ( 'NONE',  ( 87.70409100286292414, 71.53177522571066049, 96.71266027437792445 ) ) ;
#68996=ORIENTED_EDGE ( 'NONE', *, *, #42865, .T. ) ;
#68997=VERTEX_POINT ( 'NONE', #68250 ) ;
#69002=CARTESIAN_POINT ( 'NONE',  ( 83.89391322244436822, 88.18319050751493648, -100.0339087179661703 ) ) ;
#69004=CARTESIAN_POINT ( 'NONE',  ( 77.39114642429960611, 120.6499999999999915, -71.77848634863110533 ) ) ;
#69006=CARTESIAN_POINT ( 'NONE',  ( 92.32962665258456525, 81.71068249639864689, 74.36911441044827598 ) ) ;
#69014=AXIS2_PLACEMENT_3D ( 'NONE', #6686, #21679, #47999 ) ;
#69034=CARTESIAN_POINT ( 'NONE',  ( 76.39898589339213686, 74.81620433377382540, -90.65754775987947767 ) ) ;
#69058=ADVANCED_FACE ( 'NONE', ( #89142 ), #26901, .F. ) ;
#69081=CARTESIAN_POINT ( 'NONE',  ( -10.08507579090307971, 74.81978989419388881, -130.1661673264300418 ) ) ;
#69099=PLANE ( 'NONE',  #75655 ) ;
#69112=CARTESIAN_POINT ( 'NONE',  ( -105.4788588808464027, 120.6499999999999915, 3.968749999998844924 ) ) ;
#69129=DIRECTION ( 'NONE',  ( 0.000000000000000000, 0.000000000000000000, 1.000000000000000000 ) ) ;
#69153=CARTESIAN_POINT ( 'NONE',  ( -82.35292268805503113, 95.08639429146515454, -85.28591416242375089 ) ) ;
#69170=EDGE_CURVE ( 'NONE', #1704, #51660, #25333, .T. ) ;
#69209=CARTESIAN_POINT ( 'NONE',  ( 3.299336700116783483, 94.84201444875797904, -118.5128796971597609 ) ) ;
#69260=EDGE_LOOP ( 'NONE', ( #84341, #67636 ) ) ;
#69262=CARTESIAN_POINT ( 'NONE',  ( -96.70003673985446824, 93.55484823631823588, -87.71605664018984783 ) ) ;
#69267=AXIS2_PLACEMENT_3D ( 'NONE', #6703, #7166, #41651 ) ;
#69271=EDGE_CURVE ( 'NONE', #3921, #79223, #83448, .T. ) ;
#69289=ORIENTED_EDGE ( 'NONE', *, *, #77024, .F. ) ;
#69335=FACE_OUTER_BOUND ( 'NONE', #7116, .T. ) ;
#69381=ORIENTED_EDGE ( 'NONE', *, *, #54081, .T. ) ;
#69387=ORIENTED_EDGE ( 'NONE', *, *, #66591, .F. ) ;
#69397=CARTESIAN_POINT ( 'NONE',  ( -118.2371168503542407, 73.28361289573329884, -8.694557611692772525 ) ) ;
#69399=VERTEX_POINT ( 'NONE', #8037 ) ;
#69419=DIRECTION ( 'NONE',  ( 0.000000000000000000, 1.000000000000000000, 0.000000000000000000 ) ) ;
#69439=CARTESIAN_POINT ( 'NONE',  ( 98.82395782888086444, 74.16976894168011825, 85.31568053864990020 ) ) ;
#69452=CARTESIAN_POINT ( 'NONE',  ( -97.46299999999996544, 82.54999999999999716, -3.402902457276681768E-13 ) ) ;
#69454=VECTOR ( 'NONE', #55991, 1000.000000000000000 ) ;
#69457=LINE ( 'NONE', #42175, #2249 ) ;
#69459=VERTEX_POINT ( 'NONE', #85264 ) ;
#69478=CARTESIAN_POINT ( 'NONE',  ( -74.43373480440688184, 84.21498941703525531, 92.27768215250002015 ) ) ;
#69483=EDGE_CURVE ( 'NONE', #65340, #79836, #1683, .T. ) ;
#69485=CARTESIAN_POINT ( 'NONE',  ( 74.36911441044797755, 81.71068249639866110, -92.32962665258484947 ) ) ;
#69491=ADVANCED_FACE ( 'NONE', ( #36194 ), #14416, .T. ) ;
#69502=CARTESIAN_POINT ( 'NONE',  ( 86.13165781700342905, 94.84303900880917126, -81.47101467905569905 ) ) ;
#69539=CARTESIAN_POINT ( 'NONE',  ( -81.76240029069585091, 70.17671898886891313, -85.85219768521579908 ) ) ;
#69552=CARTESIAN_POINT ( 'NONE',  ( 91.73035097708802255, 69.84937019662271496, -92.90380151375003948 ) ) ;
#69571=ORIENTED_EDGE ( 'NONE', *, *, #24426, .T. ) ;
#69609=CARTESIAN_POINT ( 'NONE',  ( -92.32962665258507684, 82.54999999999999716, -74.36911441044765070 ) ) ;
#69625=LINE ( 'NONE', #63254, #3019 ) ;
#69628=CARTESIAN_POINT ( 'NONE',  ( 12.61753767970230200, 84.21537865765687059, 117.8827776564339302 ) ) ;
#69642=CARTESIAN_POINT ( 'NONE',  ( 6.174546696621030198E-16, 127.0000000000000000, -108.2293999999999983 ) ) ;
#69702=CARTESIAN_POINT ( 'NONE',  ( -31.75000000000000000, 124.5870000000000033, -3.175000000000219647 ) ) ;
#69704=ADVANCED_FACE ( 'NONE', ( #26141 ), #12513, .F. ) ;
#69716=CARTESIAN_POINT ( 'NONE',  ( 11.89174298505462524, 78.07232539501590907, 130.0133884065672589 ) ) ;
#69725=ORIENTED_EDGE ( 'NONE', *, *, #83033, .T. ) ;
#69735=EDGE_CURVE ( 'NONE', #70474, #14878, #55920, .T. ) ;
#69753=CARTESIAN_POINT ( 'NONE',  ( 130.2664984484595720, 73.28356282573680858, 8.694507028641202950 ) ) ;
#69754=ORIENTED_EDGE ( 'NONE', *, *, #61859, .T. ) ;
#69770=VERTEX_POINT ( 'NONE', #22917 ) ;
#69773=AXIS2_PLACEMENT_3D ( 'NONE', #35159, #41967, #62870 ) ;
#69796=EDGE_CURVE ( 'NONE', #50035, #12421, #22465, .T. ) ;
#69812=DIRECTION ( 'NONE',  ( 0.2588190451025269012, 0.000000000000000000, -0.9659258262890665359 ) ) ;
#69814=CARTESIAN_POINT ( 'NONE',  ( 100.5877680347015399, 85.83513192049082363, 83.22850972642827116 ) ) ;
#69822=EDGE_CURVE ( 'NONE', #48773, #81111, #63797, .T. ) ;
#69828=CARTESIAN_POINT ( 'NONE',  ( 72.96458098368701428, 127.0000000000000000, -72.96458098368670164 ) ) ;
#69848=DIRECTION ( 'NONE',  ( 0.000000000000000000, 1.000000000000000000, 0.000000000000000000 ) ) ;
#69852=CARTESIAN_POINT ( 'NONE',  ( 8.383266637423213652, 73.00087262779534569, -118.2596760195012848 ) ) ;
#69857=EDGE_LOOP ( 'NONE', ( #42438, #58978, #9080, #1130 ) ) ;
#69858=CARTESIAN_POINT ( 'NONE',  ( 0.000000000000000000, 103.1240000000000236, 0.000000000000000000 ) ) ;
#69903=VECTOR ( 'NONE', #71717, 1000.000000000000000 ) ;
#69911=ORIENTED_EDGE ( 'NONE', *, *, #28768, .T. ) ;
#69918=AXIS2_PLACEMENT_3D ( 'NONE', #51643, #30771, #58461 ) ;
#69927=ORIENTED_EDGE ( 'NONE', *, *, #80457, .T. ) ;
#69928=CARTESIAN_POINT ( 'NONE',  ( -75.37293521528297902, 88.18374315479975678, 91.51255889651606878 ) ) ;
#69931=CARTESIAN_POINT ( 'NONE',  ( -117.9083627453486827, 85.43299024555680887, 12.37536754217487101 ) ) ;
#69934=ORIENTED_EDGE ( 'NONE', *, *, #23151, .F. ) ;
#69935=LINE ( 'NONE', #42207, #24687 ) ;
#69947=EDGE_CURVE ( 'NONE', #11982, #60807, #34575, .T. ) ;
#69950=CARTESIAN_POINT ( 'NONE',  ( 74.43373480440749290, 84.21498941703526953, -92.27768215249952277 ) ) ;
#69979=CARTESIAN_POINT ( 'NONE',  ( 72.96458098368701428, 127.0000000000000000, -80.90208098368670164 ) ) ;
#69982=CIRCLE ( 'NONE', #19204, 5.041900000000000048 ) ;
#69986=ORIENTED_EDGE ( 'NONE', *, *, #8773, .F. ) ;
#70000=CARTESIAN_POINT ( 'NONE',  ( 94.33955404248733601, 70.17666187254644683, -90.25011051337669699 ) ) ;
#70020=EDGE_CURVE ( 'NONE', #68005, #12422, #59146, .T. ) ;
#70028=DIRECTION ( 'NONE',  ( -1.000000000000000000, 0.000000000000000000, -7.067626426349370916E-15 ) ) ;
#70029=AXIS2_PLACEMENT_3D ( 'NONE', #56964, #84705, #7490 ) ;
#70031=CARTESIAN_POINT ( 'NONE',  ( -99.77245543246419857, 76.20343663217359165, 84.20430400022985395 ) ) ;
#70049=CARTESIAN_POINT ( 'NONE',  ( -83.63178471058881769, 77.68489675156565966, -100.2530235599237329 ) ) ;
#70050=CARTESIAN_POINT ( 'NONE',  ( -75.38763434846467248, 88.17653575778736297, -91.50010255991641372 ) ) ;
#70072=CARTESIAN_POINT ( 'NONE',  ( 12.03238568418269416, 86.63481793440479350, 117.9438919316608008 ) ) ;
#70081=DIRECTION ( 'NONE',  ( 0.000000000000000000, 0.000000000000000000, 1.000000000000000000 ) ) ;
#70102=CARTESIAN_POINT ( 'NONE',  ( 11.57394144444449502, 87.79471777913514074, -117.9898073157514915 ) ) ;
#70103=CARTESIAN_POINT ( 'NONE',  ( -5.244075232672812170, 94.12423341047687586, 130.4512049017868094 ) ) ;
#70108=ORIENTED_EDGE ( 'NONE', *, *, #79929, .T. ) ;
#70114=CARTESIAN_POINT ( 'NONE',  ( 103.1875000000000000, 101.5999999999999943, 5.041900000000359761 ) ) ;
#70120=LINE ( 'NONE', #7892, #40327 ) ;
#70126=AXIS2_PLACEMENT_3D ( 'NONE', #44637, #72370, #8817 ) ;
#70133=CARTESIAN_POINT ( 'NONE',  ( -91.72954454028258908, 77.68452069048194630, 75.10852668448676184 ) ) ;
#70137=VERTEX_POINT ( 'NONE', #30945 ) ;
#70164=VERTEX_POINT ( 'NONE', #16875 ) ;
#70178=EDGE_CURVE ( 'NONE', #16533, #5020, #70840, .T. ) ;
#70199=ORIENTED_EDGE ( 'NONE', *, *, #39048, .F. ) ;
#70225=LINE ( 'NONE', #21187, #5393 ) ;
#70227=DIRECTION ( 'NONE',  ( 0.000000000000000000, 1.000000000000000000, 0.000000000000000000 ) ) ;
#70243=EDGE_CURVE ( 'NONE', #72171, #51571, #37438, .T. ) ;
#70261=CARTESIAN_POINT ( 'NONE',  ( 0.000000000000000000, 124.5870000000000033, 0.000000000000000000 ) ) ;
#70272=EDGE_LOOP ( 'NONE', ( #8079, #44689 ) ) ;
#70286=EDGE_CURVE ( 'NONE', #5023, #16980, #5936, .T. ) ;
#70306=FACE_OUTER_BOUND ( 'NONE', #47666, .T. ) ;
#70334=CARTESIAN_POINT ( 'NONE',  ( 94.62072105690005230, 70.27892663483461888, 89.95524642164141937 ) ) ;
#70359=B_SPLINE_CURVE_WITH_KNOTS ( 'NONE', 3,
 ( #61932, #82857, #34227, #89664, #1063, #41479, #83742, #70102, #49640, #20171, #35118, #54646, #82409, #6532, #49188, #7426, #83294, #76922, #77365, #47845, #69209, #14701, #15144, #6981, #42820, #55541 ),
 .UNSPECIFIED., .F., .F.,
 ( 4, 2, 2, 2, 2, 2, 2, 2, 2, 2, 2, 2, 4 ),
 ( 0.01987186023414422298, 0.02111327400948153146, 0.02235468778481883648, 0.02483751533549341181, 0.02607892911083071683, 0.02732034288616802531, 0.02980317043684266656, 0.03228599798751731476, 0.03352741176285463365, 0.03476882553819194560, 0.03725165308886656951, 0.03849306686420388146, 0.03973448063954118648 ),
 .UNSPECIFIED. ) ;
#70366=CARTESIAN_POINT ( 'NONE',  ( -103.1875000000000000, 117.4749999999999943, -1.080832317973422076E-12 ) ) ;
#70369=CARTESIAN_POINT ( 'NONE',  ( -88.44409384118955586, 93.33902940301969409, 78.95116244206113265 ) ) ;
#70383=ORIENTED_EDGE ( 'NONE', *, *, #52222, .T. ) ;
#70416=DIRECTION ( 'NONE',  ( 0.000000000000000000, 1.000000000000000000, 0.000000000000000000 ) ) ;
#70428=VECTOR ( 'NONE', #81521, 1000.000000000000000 ) ;
#70429=LINE ( 'NONE', #69979, #75318 ) ;
#70447=VERTEX_POINT ( 'NONE', #82695 ) ;
#70454=CARTESIAN_POINT ( 'NONE',  ( 89.95524642164112095, 70.27892663483459046, -94.62072105690033652 ) ) ;
#70459=CARTESIAN_POINT ( 'NONE',  ( -103.1875000000000000, 117.4749999999999943, 7.143749999998919797 ) ) ;
#70474=VERTEX_POINT ( 'NONE', #62220 ) ;
#70499=ORIENTED_EDGE ( 'NONE', *, *, #31019, .F. ) ;
#70501=CARTESIAN_POINT ( 'NONE',  ( -81.47101467905596905, 94.84303900880915705, -86.13165781700311641 ) ) ;
#70559=CARTESIAN_POINT ( 'NONE',  ( -11.57415360872103172, 87.79424630570802890, 130.0420457590604144 ) ) ;
#70560=DIRECTION ( 'NONE',  ( -1.000000000000000000, 0.000000000000000000, -1.047445008332813989E-14 ) ) ;
#70572=ADVANCED_FACE ( 'NONE', ( #44899 ), #10394, .T. ) ;
#70578=CARTESIAN_POINT ( 'NONE',  ( -3.174999999999644995, 111.1250000000000000, -33.98325472291465132 ) ) ;
#70590=VECTOR ( 'NONE', #75989, 1000.000000000000000 ) ;
#70603=CARTESIAN_POINT ( 'NONE',  ( -7.195828152521259823E-13, 117.4749999999999943, 95.25000000000000000 ) ) ;
#70606=ORIENTED_EDGE ( 'NONE', *, *, #77607, .T. ) ;
#70609=CARTESIAN_POINT ( 'NONE',  ( 10.08507579090307971, 74.81978989419388881, 130.1661673264300418 ) ) ;
#70647=ADVANCED_FACE ( 'NONE', ( #41541 ), #33851, .T. ) ;
#70653=CARTESIAN_POINT ( 'NONE',  ( -130.4017839623309669, 71.54617234588344843, 6.354402276675589434 ) ) ;
#70656=CARTESIAN_POINT ( 'NONE',  ( 0.000000000000000000, 124.5870000000000033, 0.000000000000000000 ) ) ;
#70687=LINE ( 'NONE', #22543, #71719 ) ;
#70742=ORIENTED_EDGE ( 'NONE', *, *, #33186, .T. ) ;
#70750=ADVANCED_FACE ( 'NONE', ( #21585 ), #29292, .F. ) ;
#70763=ORIENTED_EDGE ( 'NONE', *, *, #61487, .F. ) ;
#70787=DIRECTION ( 'NONE',  ( 3.596091637922019804E-15, 0.000000000000000000, 1.000000000000000000 ) ) ;
#70791=CARTESIAN_POINT ( 'NONE',  ( 100.8068867829397703, 80.88456863959029874, 82.96304607088372052 ) ) ;
#70793=DIRECTION ( 'NONE',  ( 0.000000000000000000, 0.000000000000000000, 1.000000000000000000 ) ) ;
#70795=ORIENTED_EDGE ( 'NONE', *, *, #63143, .T. ) ;
#70809=VECTOR ( 'NONE', #32899, 999.9999999999998863 ) ;
#70829=CARTESIAN_POINT ( 'NONE',  ( -84.12159398442656766, 95.25015226514366873, 83.54193218351881001 ) ) ;
#70831=EDGE_CURVE ( 'NONE', #12282, #72980, #77433, .T. ) ;
#70840=CIRCLE ( 'NONE', #82458, 7.937500000000000000 ) ;
#70853=DIRECTION ( 'NONE',  ( 0.000000000000000000, 0.000000000000000000, 1.000000000000000000 ) ) ;
#70857=CARTESIAN_POINT ( 'NONE',  ( 74.36911441044797755, 83.38952084682853183, -92.32962665258484947 ) ) ;
#70871=DIRECTION ( 'NONE',  ( 0.2588190451025229599, 0.000000000000000000, 0.9659258262890676461 ) ) ;
#70873=DIRECTION ( 'NONE',  ( -0.8660254037844384856, 0.000000000000000000, 0.5000000000000003331 ) ) ;
#70879=DIRECTION ( 'NONE',  ( 0.000000000000000000, 1.000000000000000000, 0.000000000000000000 ) ) ;
#70889=FACE_OUTER_BOUND ( 'NONE', #36583, .T. ) ;
#70919=CARTESIAN_POINT ( 'NONE',  ( 0.000000000000000000, 127.0000000000000000, 0.000000000000000000 ) ) ;
#70922=EDGE_CURVE ( 'NONE', #9197, #50419, #9290, .T. ) ;
#70938=EDGE_CURVE ( 'NONE', #37445, #40480, #78960, .T. ) ;
#70945=ADVANCED_FACE ( 'NONE', ( #12871 ), #40556, .F. ) ;
#70956=ORIENTED_EDGE ( 'NONE', *, *, #44395, .F. ) ;
#70961=CARTESIAN_POINT ( 'NONE',  ( -78.95116244206084843, 93.33902940301970830, -88.44409384118986850 ) ) ;
#70965=VECTOR ( 'NONE', #53449, 1000.000000000000000 ) ;
#70983=EDGE_LOOP ( 'NONE', ( #47916, #68126, #37667, #80346 ) ) ;
#71020=CIRCLE ( 'NONE', #84056, 24.63800000000000168 ) ;
#71025=CARTESIAN_POINT ( 'NONE',  ( 72.96458098368701428, 127.0000000000000000, -65.02708098368670164 ) ) ;
#71032=CARTESIAN_POINT ( 'NONE',  ( -72.96458098368600531, 117.4749999999999943, -72.96458098368781009 ) ) ;
#71049=DIRECTION ( 'NONE',  ( 0.000000000000000000, 0.000000000000000000, 1.000000000000000000 ) ) ;
#71053=ORIENTED_EDGE ( 'NONE', *, *, #6920, .F. ) ;
#71067=ORIENTED_EDGE ( 'NONE', *, *, #43328, .T. ) ;
#71070=CARTESIAN_POINT ( 'NONE',  ( 4.100932966941606139, 70.52316614063619227, 130.4921811224707824 ) ) ;
#71071=CARTESIAN_POINT ( 'NONE',  ( -100.5877680347020799, 85.83513192049078100, -83.22850972642753220 ) ) ;
#71090=PLANE ( 'NONE',  #59394 ) ;
#71099=ORIENTED_EDGE ( 'NONE', *, *, #17540, .T. ) ;
#71110=CARTESIAN_POINT ( 'NONE',  ( -130.4924667154230633, 70.52006616879378953, -4.092011266637315181 ) ) ;
#71142=LINE ( 'NONE', #63412, #82918 ) ;
#71149=VECTOR ( 'NONE', #41300, 1000.000000000000114 ) ;
#71172=AXIS2_PLACEMENT_3D ( 'NONE', #44472, #37683, #65383 ) ;
#71196=ORIENTED_EDGE ( 'NONE', *, *, #54480, .F. ) ;
#71201=ORIENTED_EDGE ( 'NONE', *, *, #45461, .T. ) ;
#71205=FACE_OUTER_BOUND ( 'NONE', #39815, .T. ) ;
#71208=DIRECTION ( 'NONE',  ( 0.000000000000000000, 1.000000000000000000, 0.000000000000000000 ) ) ;
#71232=AXIS2_PLACEMENT_3D ( 'NONE', #11187, #44813, #4390 ) ;
#71245=CARTESIAN_POINT ( 'NONE',  ( 84.36969927706093131, 75.84295037288958952, 99.63271100832298544 ) ) ;
#71261=CARTESIAN_POINT ( 'NONE',  ( 74.70281015415382342, 79.25941250729455589, 92.05992619857379111 ) ) ;
#71262=LINE ( 'NONE', #77458, #35625 ) ;
#71279=DIRECTION ( 'NONE',  ( 0.000000000000000000, 0.000000000000000000, -1.000000000000000000 ) ) ;
#71282=CARTESIAN_POINT ( 'NONE',  ( -89.55214429302371570, 92.12496802699141085, 77.69357874334745873 ) ) ;
#71289=ORIENTED_EDGE ( 'NONE', *, *, #23151, .T. ) ;
#71291=DIRECTION ( 'NONE',  ( 1.000000000000000000, 0.000000000000000000, 1.047444401652940007E-14 ) ) ;
#71297=DIRECTION ( 'NONE',  ( -1.000000000000000000, 0.000000000000000000, 0.000000000000000000 ) ) ;
#71309=VERTEX_POINT ( 'NONE', #4597 ) ;
#71312=VERTEX_POINT ( 'NONE', #66812 ) ;
#71316=DIRECTION ( 'NONE',  ( 0.000000000000000000, 0.000000000000000000, 1.000000000000000000 ) ) ;
#71325=ORIENTED_EDGE ( 'NONE', *, *, #72591, .T. ) ;
#71327=ADVANCED_FACE ( 'NONE', ( #26377, #40450 ), #47696, .T. ) ;
#71328=DIRECTION ( 'NONE',  ( -1.000000000000000000, 0.000000000000000000, -3.576143065239989638E-15 ) ) ;
#71365=CARTESIAN_POINT ( 'NONE',  ( 12.70000000000000107, 82.54999999999999716, 129.9368274816650910 ) ) ;
#71369=LINE ( 'NONE', #30903, #45789 ) ;
#71371=DIRECTION ( 'NONE',  ( 0.000000000000000000, 0.000000000000000000, 1.000000000000000000 ) ) ;
#71376=CARTESIAN_POINT ( 'NONE',  ( -77.39114642430010349, 127.0000000000000000, 71.77848634863050847 ) ) ;
#71398=EDGE_LOOP ( 'NONE', ( #86949, #89265 ) ) ;
#71408=FACE_OUTER_BOUND ( 'NONE', #69857, .T. ) ;
#71409=CARTESIAN_POINT ( 'NONE',  ( 0.000000000000000000, 124.5870000000000033, 0.000000000000000000 ) ) ;
#71410=VECTOR ( 'NONE', #85782, 999.9999999999998863 ) ;
#71432=CARTESIAN_POINT ( 'NONE',  ( -100.8961411191535973, 120.6499999999999915, -3.968750000001104894 ) ) ;
#71465=CARTESIAN_POINT ( 'NONE',  ( -6.714856022345324860, 93.33757043186105307, 130.3836582748265585 ) ) ;
#71471=LINE ( 'NONE', #67200, #66981 ) ;
#71478=ADVANCED_FACE ( 'NONE', ( #83156 ), #29522, .F. ) ;
#71482=ORIENTED_EDGE ( 'NONE', *, *, #37979, .F. ) ;
#71515=CARTESIAN_POINT ( 'NONE',  ( 9.554664674393775314, 74.17305037928137779, 130.2061759407760633 ) ) ;
#71525=ORIENTED_EDGE ( 'NONE', *, *, #10243, .T. ) ;
#71534=CARTESIAN_POINT ( 'NONE',  ( 72.96458098368701428, 127.0000000000000000, -65.02708098368670164 ) ) ;
#71555=CARTESIAN_POINT ( 'NONE',  ( -130.5246120830808820, 70.17656663518266669, 2.891956274607122790 ) ) ;
#71595=CARTESIAN_POINT ( 'NONE',  ( -2.883471595053325398, 94.92538689125282758, -130.5247975405367526 ) ) ;
#71612=DIRECTION ( 'NONE',  ( -1.000000000000000000, 0.000000000000000000, -3.491481338843133355E-15 ) ) ;
#71615=CARTESIAN_POINT ( 'NONE',  ( 74.44936585838333087, 84.21376545118702950, 92.26493792250116144 ) ) ;
#71617=ORIENTED_EDGE ( 'NONE', *, *, #33916, .F. ) ;
#71639=ORIENTED_EDGE ( 'NONE', *, *, #76963, .F. ) ;
#71649=FACE_BOUND ( 'NONE', #24724, .T. ) ;
#71654=FACE_OUTER_BOUND ( 'NONE', #10227, .T. ) ;
#71660=CIRCLE ( 'NONE', #10746, 7.937500000000000000 ) ;
#71661=LINE ( 'NONE', #50293, #64941 ) ;
#71677=CARTESIAN_POINT ( 'NONE',  ( 4.163101094985349692E-14, 127.0000000000000000, -107.7702177616926065 ) ) ;
#71680=ORIENTED_EDGE ( 'NONE', *, *, #30467, .T. ) ;
#71691=ORIENTED_EDGE ( 'NONE', *, *, #68690, .T. ) ;
#71708=EDGE_CURVE ( 'NONE', #76254, #57775, #12993, .T. ) ;
#71717=DIRECTION ( 'NONE',  ( 0.000000000000000000, -1.000000000000000000, 0.000000000000000000 ) ) ;
#71719=VECTOR ( 'NONE', #1657, 999.9999999999998863 ) ;
#71725=CARTESIAN_POINT ( 'NONE',  ( 92.27899210470920366, 80.89685143461889538, -74.43211355457083300 ) ) ;
#71726=ORIENTED_EDGE ( 'NONE', *, *, #64421, .T. ) ;
#71733=EDGE_CURVE ( 'NONE', #12494, #69459, #42080, .T. ) ;
#71763=EDGE_LOOP ( 'NONE', ( #45617, #15208 ) ) ;
#71791=EDGE_LOOP ( 'NONE', ( #86461, #21125, #37971, #35533 ) ) ;
#71800=CARTESIAN_POINT ( 'NONE',  ( 100.0213216842705748, 88.17609398443094904, -83.90854149456399114 ) ) ;
#71825=VECTOR ( 'NONE', #51780, 1000.000000000000114 ) ;
#71827=DIRECTION ( 'NONE',  ( 0.000000000000000000, -1.000000000000000000, 0.000000000000000000 ) ) ;
#71843=EDGE_CURVE ( 'NONE', #89451, #66196, #29299, .T. ) ;
#71845=DIRECTION ( 'NONE',  ( 0.000000000000000000, 1.000000000000000000, 0.000000000000000000 ) ) ;
#71846=DIRECTION ( 'NONE',  ( 0.000000000000000000, 0.000000000000000000, -1.000000000000000000 ) ) ;
#71882=CARTESIAN_POINT ( 'NONE',  ( -2.684158038187649039E-15, 69.84999999999999432, 130.5560000000000116 ) ) ;
#71889=ADVANCED_FACE ( 'NONE', ( #8407 ), #71090, .F. ) ;
#71893=DIRECTION ( 'NONE',  ( -3.406823656978775284E-15, 0.000000000000000000, -1.000000000000000000 ) ) ;
#71921=ORIENTED_EDGE ( 'NONE', *, *, #70286, .T. ) ;
#71937=VECTOR ( 'NONE', #30044, 1000.000000000000000 ) ;
#71982=ORIENTED_EDGE ( 'NONE', *, *, #37508, .T. ) ;
#71989=FACE_OUTER_BOUND ( 'NONE', #75263, .T. ) ;
#71999=ORIENTED_EDGE ( 'NONE', *, *, #70938, .T. ) ;
#72005=DIRECTION ( 'NONE',  ( 0.000000000000000000, 0.000000000000000000, -1.000000000000000000 ) ) ;
#72011=DIRECTION ( 'NONE',  ( -1.000000000000000000, 0.000000000000000000, -3.491481338843133355E-15 ) ) ;
#72033=CARTESIAN_POINT ( 'NONE',  ( -6.349842397765894653, 93.55646220832403515, -130.4020064843512614 ) ) ;
#72071=ORIENTED_EDGE ( 'NONE', *, *, #45261, .F. ) ;
#72097=CARTESIAN_POINT ( 'NONE',  ( 68.53801554307389665, 127.0000000000000000, 74.15067561874289481 ) ) ;
#72098=DIRECTION ( 'NONE',  ( 0.000000000000000000, 0.000000000000000000, 1.000000000000000000 ) ) ;
#72114=LINE ( 'NONE', #30336, #42521 ) ;
#72138=DIRECTION ( 'NONE',  ( 0.000000000000000000, 1.000000000000000000, 0.000000000000000000 ) ) ;
#72142=AXIS2_PLACEMENT_3D ( 'NONE', #48483, #69419, #34434 ) ;
#72145=CARTESIAN_POINT ( 'NONE',  ( 87.71317827224373787, 71.15456258041355397, 79.76251016565973373 ) ) ;
#72168=CARTESIAN_POINT ( 'NONE',  ( 0.000000000000000000, 125.4759999999999991, 0.000000000000000000 ) ) ;
#72170=CARTESIAN_POINT ( 'NONE',  ( 91.72954497613136482, 77.68452076096559722, -75.10852726169345317 ) ) ;
#72171=VERTEX_POINT ( 'NONE', #41002 ) ;
#72181=CARTESIAN_POINT ( 'NONE',  ( 100.8961411191535973, 120.6499999999999915, -3.968749999999580336 ) ) ;
#72220=DIRECTION ( 'NONE',  ( -0.000000000000000000, 1.000000000000000000, 0.000000000000000000 ) ) ;
#72233=LINE ( 'NONE', #17268, #84335 ) ;
#72250=CARTESIAN_POINT ( 'NONE',  ( 3.174999999999889688, 104.3431970271541900, 31.75000000000000000 ) ) ;
#72254=ORIENTED_EDGE ( 'NONE', *, *, #77607, .F. ) ;
#72285=CARTESIAN_POINT ( 'NONE',  ( -100.8594679592206802, 82.54999999999999716, -82.89895571708333932 ) ) ;
#72318=CARTESIAN_POINT ( 'NONE',  ( 2.332952152375709937E-14, 103.1240000000000236, -190.5000000000000000 ) ) ;
#72351=CYLINDRICAL_SURFACE ( 'NONE', #12362, 7.937500000000000000 ) ;
#72361=EDGE_CURVE ( 'NONE', #15453, #68541, #50505, .T. ) ;
#72370=DIRECTION ( 'NONE',  ( 0.8660254037844351549, 0.000000000000000000, 0.5000000000000061062 ) ) ;
#72389=CARTESIAN_POINT ( 'NONE',  ( 118.3034456680046134, 72.47328848629021536, 7.741103959108575516 ) ) ;
#72404=VECTOR ( 'NONE', #62501, 1000.000000000000000 ) ;
#72426=VERTEX_POINT ( 'NONE', #77785 ) ;
#72434=LINE ( 'NONE', #58776, #84522 ) ;
#72465=FACE_OUTER_BOUND ( 'NONE', #46631, .T. ) ;
#72476=ORIENTED_EDGE ( 'NONE', *, *, #29285, .T. ) ;
#72478=CARTESIAN_POINT ( 'NONE',  ( -12.03249045273851969, 86.63451674300236505, -130.0003965276981432 ) ) ;
#72501=CARTESIAN_POINT ( 'NONE',  ( 75.38763434846404721, 88.17653575778740560, 91.50010255991693953 ) ) ;
#72507=CIRCLE ( 'NONE', #50770, 7.937500000000000000 ) ;
#72516=PLANE ( 'NONE',  #51738 ) ;
#72542=ORIENTED_EDGE ( 'NONE', *, *, #49597, .T. ) ;
#72550=CARTESIAN_POINT ( 'NONE',  ( 77.39114642429899504, 127.0000000000000000, 71.77848634863160271 ) ) ;
#72560=CARTESIAN_POINT ( 'NONE',  ( -72.96458098368751166, 117.4749999999999943, 72.96458098368620426 ) ) ;
#72569=CYLINDRICAL_SURFACE ( 'NONE', #30317, 7.143750000000004263 ) ;
#72584=EDGE_LOOP ( 'NONE', ( #88252, #49499, #30486, #53736 ) ) ;
#72591=EDGE_CURVE ( 'NONE', #28958, #54712, #59511, .T. ) ;
#72592=CIRCLE ( 'NONE', #81301, 88.90000000000000568 ) ;
#72594=CARTESIAN_POINT ( 'NONE',  ( 74.62294912200587760, 79.66725693986900581, 92.12462914090833976 ) ) ;
#72627=CARTESIAN_POINT ( 'NONE',  ( 33.98325472291465132, 124.5870000000000033, -3.174999999999999822 ) ) ;
#72752=VERTEX_POINT ( 'NONE', #55408 ) ;
#72760=DIRECTION ( 'NONE',  ( 0.000000000000000000, 0.000000000000000000, 1.000000000000000000 ) ) ;
#72766=EDGE_LOOP ( 'NONE', ( #3296, #38871, #88073, #4324 ) ) ;
#72768=CARTESIAN_POINT ( 'NONE',  ( -12.61959663417972521, 80.89626266586573422, 129.9447639770759508 ) ) ;
#72777=CARTESIAN_POINT ( 'NONE',  ( -103.1875000000000000, 117.4749999999999943, -5.041900000001080073 ) ) ;
#72799=CIRCLE ( 'NONE', #33635, 7.937500000000000000 ) ;
#72802=ORIENTED_EDGE ( 'NONE', *, *, #31407, .F. ) ;
#72816=EDGE_LOOP ( 'NONE', ( #37259, #76547, #77164, #82630, #29632, #7827 ) ) ;
#72829=DIRECTION ( 'NONE',  ( 0.000000000000000000, 1.000000000000000000, 0.000000000000000000 ) ) ;
#72839=ADVANCED_FACE ( 'NONE', ( #50854 ), #35427, .F. ) ;
#72846=CARTESIAN_POINT ( 'NONE',  ( 6.802569982901797644E-16, 69.84999999999999432, 118.5560000000000116 ) ) ;
#72926=CARTESIAN_POINT ( 'NONE',  ( 4.084841600441663445, 70.51762400537137410, -130.4926920574403937 ) ) ;
#72931=ORIENTED_EDGE ( 'NONE', *, *, #83144, .F. ) ;
#72932=CARTESIAN_POINT ( 'NONE',  ( 8.391680458684335875, 92.11847147219766896, 130.2873503055691344 ) ) ;
#72976=FACE_BOUND ( 'NONE', #13735, .T. ) ;
#72980=VERTEX_POINT ( 'NONE', #38555 ) ;
#73011=VECTOR ( 'NONE', #79146, 1000.000000000000000 ) ;
#73017=LINE ( 'NONE', #3098, #57717 ) ;
#73020=CARTESIAN_POINT ( 'NONE',  ( 80.59807192910871265, 70.66242608954391358, 86.94609723791424472 ) ) ;
#73022=ORIENTED_EDGE ( 'NONE', *, *, #74527, .F. ) ;
#73030=CARTESIAN_POINT ( 'NONE',  ( 117.9438598201575843, 86.63388195152280957, -12.03269986015406445 ) ) ;
#73031=VECTOR ( 'NONE', #15062, 1000.000000000000000 ) ;
#73057=CARTESIAN_POINT ( 'NONE',  ( 72.96458098368701428, 127.0000000000000000, -72.96458098368670164 ) ) ;
#73060=CARTESIAN_POINT ( 'NONE',  ( 3.968750000000050182, 120.6499999999999915, -100.8961411191535973 ) ) ;
#73061=ADVANCED_FACE ( 'NONE', ( #66250 ), #16792, .F. ) ;
#73066=CARTESIAN_POINT ( 'NONE',  ( -118.1052048222230155, 75.15251084995274766, 10.33146714902738061 ) ) ;
#73069=ORIENTED_EDGE ( 'NONE', *, *, #25378, .F. ) ;
#73098=CARTESIAN_POINT ( 'NONE',  ( 1.166476076187854022E-15, 125.7300000000000040, -9.525000000000000355 ) ) ;
#73103=PLANE ( 'NONE',  #19513 ) ;
#73135=CARTESIAN_POINT ( 'NONE',  ( 3.968749999999215294, 120.6499999999999915, 105.4788588808464027 ) ) ;
#73145=CARTESIAN_POINT ( 'NONE',  ( -86.19179098795268601, 92.11674985319540099, 98.06216817836288158 ) ) ;
#73215=DIRECTION ( 'NONE',  ( 0.000000000000000000, -1.000000000000000000, 0.000000000000000000 ) ) ;
#73237=CARTESIAN_POINT ( 'NONE',  ( 103.1875000000000000, 117.4749999999999943, -5.041899999999640336 ) ) ;
#73243=CARTESIAN_POINT ( 'NONE',  ( -83.89393544538295089, 76.91670260214422683, 100.0338904447229993 ) ) ;
#73249=LINE ( 'NONE', #78319, #10965 ) ;
#73251=CARTESIAN_POINT ( 'NONE',  ( 1.145694247088684285E-22, 95.25000000000000000, 118.5560000000000116 ) ) ;
#73261=EDGE_CURVE ( 'NONE', #67802, #66826, #3072, .T. ) ;
#73283=CARTESIAN_POINT ( 'NONE',  ( -9.568977433314790559, 74.15890990428199814, 118.1706578929490377 ) ) ;
#73285=DIRECTION ( 'NONE',  ( 0.000000000000000000, 1.000000000000000000, 0.000000000000000000 ) ) ;
#73291=DIRECTION ( 'NONE',  ( 0.000000000000000000, 1.000000000000000000, 0.000000000000000000 ) ) ;
#73305=DIRECTION ( 'NONE',  ( 0.000000000000000000, 1.000000000000000000, 0.000000000000000000 ) ) ;
#73308=ORIENTED_EDGE ( 'NONE', *, *, #45338, .F. ) ;
#73317=FACE_OUTER_BOUND ( 'NONE', #81760, .T. ) ;
#73324=CARTESIAN_POINT ( 'NONE',  ( 1.451892259197136103E-14, 61.59999999999999432, -118.5560000000000116 ) ) ;
#73329=CARTESIAN_POINT ( 'NONE',  ( 1.598849865763559337E-14, 95.25000000000000000, -130.5560000000000116 ) ) ;
#73332=CARTESIAN_POINT ( 'NONE',  ( -11.89031456967464706, 87.03148351030580443, -117.9583453772440151 ) ) ;
#73344=DIRECTION ( 'NONE',  ( 0.000000000000000000, 0.000000000000000000, 1.000000000000000000 ) ) ;
#73354=CARTESIAN_POINT ( 'NONE',  ( -8.391680458684334099, 92.11847147219766896, -130.2873503055691629 ) ) ;
#73366=ORIENTED_EDGE ( 'NONE', *, *, #80409, .T. ) ;
#73372=CARTESIAN_POINT ( 'NONE',  ( 8.690912999409459161, 73.28018275885442279, -130.2667388509219677 ) ) ;
#73373=ADVANCED_FACE ( 'NONE', ( #87062, #52494, #38440, #2609 ), #73415, .F. ) ;
#73375=CARTESIAN_POINT ( 'NONE',  ( 74.87617104506175281, 86.64222086580517157, 91.91945768840264464 ) ) ;
#73395=CYLINDRICAL_SURFACE ( 'NONE', #73853, 130.5560000000000116 ) ;
#73407=VERTEX_POINT ( 'NONE', #86171 ) ;
#73415=CYLINDRICAL_SURFACE ( 'NONE', #8856, 118.5560000000000116 ) ;
#73416=ORIENTED_EDGE ( 'NONE', *, *, #37508, .F. ) ;
#73425=VERTEX_POINT ( 'NONE', #43916 ) ;
#73453=ADVANCED_FACE ( 'NONE', ( #23945 ), #18002, .F. ) ;
#73491=B_SPLINE_CURVE_WITH_KNOTS ( 'NONE', 3,
 ( #841, #43050, #70791, #83976, #83515, #83087, #62163, #21749, #77154, #76248, #41707, #69439, #27650, #7215, #8561, #34904, #42598, #63511, #36261, #13571, #70334, #8110, #89439, #21288, #35797, #76702, #27200, #54875, #20402, #75806, #62615, #68989, #89898, #41261, #28085, #6758, #50318, #57587, #71245, #10769, #79400, #44394, #51207, #30346, #58043, #58913, #23544, #17164 ),
 .UNSPECIFIED., .F., .F.,
 ( 4, 2, 2, 2, 2, 2, 2, 2, 2, 1, 2, 2, 2, 2, 2, 2, 2, 2, 2, 2, 2, 1, 2, 2, 4 ),
 ( 0.05959919981814692375, 0.06208168506169063627, 0.06332292768346249601, 0.06456417030523434186, 0.06704665554877808908, 0.06828789817054996270, 0.06952914079232185018, 0.07201162603586555577, 0.07325286865763741551, 0.07449411127940928912, 0.07573535390118114885, 0.07697659652295302246, 0.07945908176649678356, 0.08194156701004054466, 0.08318280963181240439, 0.08442405225358426413, 0.08690653749712799747, 0.08814778011889984333, 0.08938902274067170306, 0.09187150798421539477, 0.09311275060598722675, 0.09435399322775908648, 0.09559523584953094621, 0.09683647847130277819, 0.09931896371484646990 ),
 .UNSPECIFIED. ) ;
#73495=CARTESIAN_POINT ( 'NONE',  ( 72.96458098368701428, 127.0000000000000000, -78.00648098368678518 ) ) ;
#73515=CARTESIAN_POINT ( 'NONE',  ( -118.4716181662680583, 70.66242608954391358, -4.488731742999155117 ) ) ;
#73527=VECTOR ( 'NONE', #19521, 1000.000000000000000 ) ;
#73556=CARTESIAN_POINT ( 'NONE',  ( 72.96458098368701428, 117.4749999999999943, -67.92268098368680285 ) ) ;
#73557=CARTESIAN_POINT ( 'NONE',  ( -130.0919229099370398, 88.91113633199481114, -10.99998730946133918 ) ) ;
#73579=VECTOR ( 'NONE', #78951, 1000.000000000000000 ) ;
#73580=ADVANCED_FACE ( 'NONE', ( #11652 ), #46136, .F. ) ;
#73589=DIRECTION ( 'NONE',  ( 0.5000000000000003331, 0.000000000000000000, 0.8660254037844383745 ) ) ;
#73601=CARTESIAN_POINT ( 'NONE',  ( -117.9898589647455083, 87.79588542099531878, -11.57341593931141155 ) ) ;
#73605=CARTESIAN_POINT ( 'NONE',  ( 0.000000000000000000, 92.07499999999998863, 0.000000000000000000 ) ) ;
#73610=ORIENTED_EDGE ( 'NONE', *, *, #85477, .T. ) ;
#73618=DIRECTION ( 'NONE',  ( 0.000000000000000000, 1.000000000000000000, 0.000000000000000000 ) ) ;
#73620=VECTOR ( 'NONE', #1725, 1000.000000000000000 ) ;
#73627=VERTEX_POINT ( 'NONE', #7520 ) ;
#73644=DIRECTION ( 'NONE',  ( 1.047445008332813989E-14, 0.000000000000000000, -1.000000000000000000 ) ) ;
#73650=ORIENTED_EDGE ( 'NONE', *, *, #35254, .F. ) ;
#73666=( LENGTH_UNIT ( ) NAMED_UNIT ( * ) SI_UNIT ( .MILLI., .METRE. ) );
#73690=ADVANCED_FACE ( 'NONE', ( #35664 ), #1159, .F. ) ;
#73692=DIRECTION ( 'NONE',  ( 0.000000000000000000, 1.000000000000000000, 0.000000000000000000 ) ) ;
#73700=CARTESIAN_POINT ( 'NONE',  ( 107.7702177616926065, 120.6499999999999915, 4.179089330879380409E-13 ) ) ;
#73722=ORIENTED_EDGE ( 'NONE', *, *, #33186, .F. ) ;
#73727=CYLINDRICAL_SURFACE ( 'NONE', #49133, 5.041900000000001825 ) ;
#73729=VECTOR ( 'NONE', #30573, 1000.000000000000114 ) ;
#73736=EDGE_LOOP ( 'NONE', ( #22765, #13343, #12931, #26664 ) ) ;
#73737=CARTESIAN_POINT ( 'NONE',  ( -10.09446275336743781, 74.79825716961998694, 118.1263904669630733 ) ) ;
#73740=VECTOR ( 'NONE', #73822, 1000.000000000000000 ) ;
#73744=VECTOR ( 'NONE', #37086, 1000.000000000000114 ) ;
#73811=CYLINDRICAL_SURFACE ( 'NONE', #17858, 5.041900000000000048 ) ;
#73822=DIRECTION ( 'NONE',  ( 1.000000000000000000, 0.000000000000000000, 6.982966722218760189E-15 ) ) ;
#73826=LINE ( 'NONE', #67008, #54849 ) ;
#73832=CARTESIAN_POINT ( 'NONE',  ( 11.41209158312316774, 88.18445188672593815, 130.0566639163489810 ) ) ;
#73835=EDGE_CURVE ( 'NONE', #76109, #82989, #84392, .T. ) ;
#73853=AXIS2_PLACEMENT_3D ( 'NONE', #77659, #4370, #70853 ) ;
#73877=ORIENTED_EDGE ( 'NONE', *, *, #84789, .F. ) ;
#73904=CARTESIAN_POINT ( 'NONE',  ( 10.09777173618929069, 90.29655250510941755, -130.1657284840294437 ) ) ;
#73934=CARTESIAN_POINT ( 'NONE',  ( 118.1932448497438628, 91.23868085022584751, -9.271905035164968112 ) ) ;
#73954=ORIENTED_EDGE ( 'NONE', *, *, #25365, .T. ) ;
#73969=CARTESIAN_POINT ( 'NONE',  ( -118.4231949783269613, 71.15456258041351134, 5.621971333130180604 ) ) ;
#73987=CARTESIAN_POINT ( 'NONE',  ( 0.000000000000000000, 127.0000000000000000, -95.25000000000000000 ) ) ;
#73999=ORIENTED_EDGE ( 'NONE', *, *, #34297, .T. ) ;
#74011=CARTESIAN_POINT ( 'NONE',  ( -130.3279567413622715, 92.64985122628465319, -7.743850073003764933 ) ) ;
#74014=ORIENTED_EDGE ( 'NONE', *, *, #31407, .T. ) ;
#74024=CARTESIAN_POINT ( 'NONE',  ( 84.91247172076084837, 90.28418055714726620, -99.17062120112620960 ) ) ;
#74049=DIRECTION ( 'NONE',  ( 1.000000000000000000, 0.000000000000000000, 0.000000000000000000 ) ) ;
#74050=CARTESIAN_POINT ( 'NONE',  ( -105.4788588808462038, 120.6499999999999915, -3.968750000001139977 ) ) ;
#74067=CARTESIAN_POINT ( 'NONE',  ( 92.07164801315056479, 85.85031469618033384, -74.68844285250138171 ) ) ;
#74073=EDGE_LOOP ( 'NONE', ( #76519, #63930, #41785, #54727 ) ) ;
#74080=CARTESIAN_POINT ( 'NONE',  ( 72.96458098368701428, 117.4749999999999943, -72.96458098368670164 ) ) ;
#74087=( NAMED_UNIT ( * ) SI_UNIT ( $, .STERADIAN. ) SOLID_ANGLE_UNIT ( ) );
#74105=ORIENTED_EDGE ( 'NONE', *, *, #14312, .T. ) ;
#74117=CIRCLE ( 'NONE', #52355, 7.143750000000004263 ) ;
#74139=ADVANCED_FACE ( 'NONE', ( #63161 ), #49516, .F. ) ;
#74140=CYLINDRICAL_SURFACE ( 'NONE', #39218, 9.525000000000000355 ) ;
#74144=ORIENTED_EDGE ( 'NONE', *, *, #19955, .F. ) ;
#74152=PLANE ( 'NONE',  #37056 ) ;
#74155=FACE_BOUND ( 'NONE', #23306, .T. ) ;
#74156=B_SPLINE_CURVE_WITH_KNOTS ( 'NONE', 3,
 ( #89559, #40940, #47748, #76372, #48635, #49090, #27319, #14147, #48190, #68664, #76820, #83199, #62735, #20524, #41383, #54994, #61826, #13692, #41824, #55448, #54547, #89111, #82310, #75024, #6431 ),
 .UNSPECIFIED., .F., .F.,
 ( 4, 2, 2, 2, 2, 2, 2, 2, 2, 1, 2, 2, 4 ),
 ( 0.05960646776571127542, 0.06208810814592213845, 0.06332892833602757343, 0.06456974852613300841, 0.06705138890634392002, 0.06829220909644936888, 0.06953302928655483162, 0.07201466966676572934, 0.07325548985687117820, 0.07449631004697662706, 0.07573713023708206205, 0.07697795042718751091, 0.07945959080739838087 ),
 .UNSPECIFIED. ) ;
#74177=CARTESIAN_POINT ( 'NONE',  ( -100.4327019155584964, 78.46683822716998691, -83.41556370846515733 ) ) ;
#74189=VERTEX_POINT ( 'NONE', #73098 ) ;
#74237=DIRECTION ( 'NONE',  ( 6.982966722218758611E-15, 0.000000000000000000, -1.000000000000000000 ) ) ;
#74243=CARTESIAN_POINT ( 'NONE',  ( -9.549789689180773422, 90.93251752167839186, -118.1710524764278887 ) ) ;
#74262=ORIENTED_EDGE ( 'NONE', *, *, #87532, .F. ) ;
#74270=AXIS2_PLACEMENT_3D ( 'NONE', #77545, #36208, #43899 ) ;
#74282=DIRECTION ( 'NONE',  ( 0.000000000000000000, 1.000000000000000000, 0.000000000000000000 ) ) ;
#74289=CARTESIAN_POINT ( 'NONE',  ( -84.21071524772774808, 88.91113633199476851, -99.76704648670025222 ) ) ;
#74323=FACE_OUTER_BOUND ( 'NONE', #83985, .T. ) ;
#74357=CARTESIAN_POINT ( 'NONE',  ( 3.298961202091078793, 94.84210650921833974, -130.5168528568578097 ) ) ;
#74374=CARTESIAN_POINT ( 'NONE',  ( -3.968749999999935163, 127.0000000000000000, -100.8961411191535973 ) ) ;
#74387=CARTESIAN_POINT ( 'NONE',  ( 117.9898589647454799, 87.79588542099538984, 11.57341593931223223 ) ) ;
#74432=CARTESIAN_POINT ( 'NONE',  ( 72.96458098368701428, 127.0000000000000000, -65.82083098368670449 ) ) ;
#74437=LINE ( 'NONE', #54854, #33913 ) ;
#74447=LINE ( 'NONE', #25849, #8862 ) ;
#74461=CARTESIAN_POINT ( 'NONE',  ( -129.9528072873947337, 84.62817240485475168, -12.53569626682267568 ) ) ;
#74475=CARTESIAN_POINT ( 'NONE',  ( 87.44839512528858450, 93.33885111288435610, -96.94208673522955166 ) ) ;
#74479=CARTESIAN_POINT ( 'NONE',  ( -11.89159109876203146, 78.07192968827520474, -117.9582163940502966 ) ) ;
#74491=DIRECTION ( 'NONE',  ( 0.000000000000000000, 0.000000000000000000, 1.000000000000000000 ) ) ;
#74499=CARTESIAN_POINT ( 'NONE',  ( -83.22850972642717693, 85.83513192049080942, 100.5877680347024068 ) ) ;
#74510=ORIENTED_EDGE ( 'NONE', *, *, #4655, .T. ) ;
#74527=EDGE_CURVE ( 'NONE', #11232, #27146, #43034, .T. ) ;
#74537=CARTESIAN_POINT ( 'NONE',  ( 130.5559693845970344, 95.24968527363472504, -0.8339068267389735389 ) ) ;
#74563=( NAMED_UNIT ( * ) SI_UNIT ( $, .STERADIAN. ) SOLID_ANGLE_UNIT ( ) );
#74571=FACE_OUTER_BOUND ( 'NONE', #73736, .T. ) ;
#74617=CARTESIAN_POINT ( 'NONE',  ( -94.62072105690063495, 70.27892663483460467, -89.95524642164077989 ) ) ;
#74632=DIRECTION ( 'NONE',  ( 0.000000000000000000, 1.000000000000000000, 0.000000000000000000 ) ) ;
#74643=ORIENTED_EDGE ( 'NONE', *, *, #86485, .F. ) ;
#74660=DIRECTION ( 'NONE',  ( 0.000000000000000000, -1.000000000000000000, 0.000000000000000000 ) ) ;
#74672=VECTOR ( 'NONE', #1056, 1000.000000000000000 ) ;
#74697=EDGE_CURVE ( 'NONE', #2616, #32576, #45273, .T. ) ;
#74708=EDGE_CURVE ( 'NONE', #52316, #6564, #19142, .T. ) ;
#74722=CARTESIAN_POINT ( 'NONE',  ( 0.000000000000000000, 103.1240000000000236, 0.000000000000000000 ) ) ;
#74734=CARTESIAN_POINT ( 'NONE',  ( -83.40142812120586768, 86.64186789594792515, -100.4448767513720639 ) ) ;
#74747=EDGE_CURVE ( 'NONE', #65614, #43245, #64090, .T. ) ;
#74755=CARTESIAN_POINT ( 'NONE',  ( 0.000000000000000000, 61.59999999999999432, 0.000000000000000000 ) ) ;
#74768=CARTESIAN_POINT ( 'NONE',  ( 129.9368274816652047, 81.71102547120854354, -12.69999999999864038 ) ) ;
#74772=ORIENTED_EDGE ( 'NONE', *, *, #40750, .F. ) ;
#74790=FACE_OUTER_BOUND ( 'NONE', #60772, .T. ) ;
#74801=AXIS2_PLACEMENT_3D ( 'NONE', #22675, #36743, #29933 ) ;
#74804=DIRECTION ( 'NONE',  ( 0.000000000000000000, 1.000000000000000000, 0.000000000000000000 ) ) ;
#74813=EDGE_CURVE ( 'NONE', #2544, #66251, #69982, .T. ) ;
#74815=DIRECTION ( 'NONE',  ( 0.000000000000000000, -1.000000000000000000, 0.000000000000000000 ) ) ;
#74835=CARTESIAN_POINT ( 'NONE',  ( 118.3663208563465190, 93.33902940301965145, 6.712516165663437562 ) ) ;
#74846=AXIS2_PLACEMENT_3D ( 'NONE', #10047, #79098, #71827 ) ;
#74869=CIRCLE ( 'NONE', #35704, 7.143750000000004263 ) ;
#74909=CARTESIAN_POINT ( 'NONE',  ( -130.2266700119015184, 91.23859726994547259, 9.271983876140998504 ) ) ;
#74925=CARTESIAN_POINT ( 'NONE',  ( 87.71605664019014625, 93.55484823631826430, -96.70003673985416981 ) ) ;
#74927=CARTESIAN_POINT ( 'NONE',  ( 72.96458098368650269, 127.0000000000000000, 72.96458098368729850 ) ) ;
#74930=CARTESIAN_POINT ( 'NONE',  ( -0.8391700603252211232, 69.85000000000000853, -118.5560000000000400 ) ) ;
#74949=CARTESIAN_POINT ( 'NONE',  ( -118.4232034889089533, 93.94553785444267646, -5.621872244391297180 ) ) ;
#74950=CARTESIAN_POINT ( 'NONE',  ( -12.70000000000000107, 82.54999999999999716, -117.8738102209307641 ) ) ;
#74953=DIRECTION ( 'NONE',  ( 0.000000000000000000, 0.000000000000000000, 1.000000000000000000 ) ) ;
#74985=CARTESIAN_POINT ( 'NONE',  ( 130.0420937742006231, 87.79544278253750633, 11.57361518220490737 ) ) ;
#75003=CARTESIAN_POINT ( 'NONE',  ( -90.81844170390323256, 75.15251084995277608, -76.20754074253689225 ) ) ;
#75016=DIRECTION ( 'NONE',  ( 0.000000000000000000, 1.000000000000000000, 0.000000000000000000 ) ) ;
#75024=CARTESIAN_POINT ( 'NONE',  ( 0.8391700603252211232, 69.85000000000000853, 118.5560000000000400 ) ) ;
#75032=LINE ( 'NONE', #40505, #76074 ) ;
#75046=ADVANCED_FACE ( 'NONE', ( #42042, #22977 ), #14815, .T. ) ;
#75051=CARTESIAN_POINT ( 'NONE',  ( -82.89895571708295563, 82.54999999999999716, 100.8594679592209644 ) ) ;
#75054=ORIENTED_EDGE ( 'NONE', *, *, #24046, .T. ) ;
#75070=CARTESIAN_POINT ( 'NONE',  ( -96.94335780202320052, 71.76234181793741129, -87.44698480207792102 ) ) ;
#75075=CARTESIAN_POINT ( 'NONE',  ( 68.91674821478504498, 82.54999999999999716, -68.91674821478385127 ) ) ;
#75081=CARTESIAN_POINT ( 'NONE',  ( -12.70000000000000107, 82.54999999999999716, 117.8738102209307641 ) ) ;
#75083=CARTESIAN_POINT ( 'NONE',  ( -71.77848634863190114, 120.6499999999999915, 77.39114642429879609 ) ) ;
#75101=VECTOR ( 'NONE', #49355, 1000.000000000000000 ) ;
#75109=VERTEX_POINT ( 'NONE', #7541 ) ;
#75131=CARTESIAN_POINT ( 'NONE',  ( -12.61753767970230200, 84.21537865765682795, -117.8827776564338734 ) ) ;
#75138=PLANE ( 'NONE',  #21463 ) ;
#75175=CARTESIAN_POINT ( 'NONE',  ( 92.12450916458644201, 85.43299024555680887, 74.62309654709238771 ) ) ;
#75179=EDGE_LOOP ( 'NONE', ( #24122, #1887, #44358, #1434 ) ) ;
#75184=AXIS2_PLACEMENT_3D ( 'NONE', #74050, #47222, #11831 ) ;
#75231=FACE_OUTER_BOUND ( 'NONE', #82673, .T. ) ;
#75258=CYLINDRICAL_SURFACE ( 'NONE', #78289, 7.937500000000000000 ) ;
#75263=EDGE_LOOP ( 'NONE', ( #28116, #65891, #19635, #83266 ) ) ;
#75287=DIRECTION ( 'NONE',  ( 0.000000000000000000, 1.000000000000000000, 0.000000000000000000 ) ) ;
#75309=CARTESIAN_POINT ( 'NONE',  ( -31.75000000000000000, 104.3431970271541900, 3.174999999999779998 ) ) ;
#75313=CARTESIAN_POINT ( 'NONE',  ( -118.2594037030539198, 73.00424585431356661, -8.387096233283337199 ) ) ;
#75318=VECTOR ( 'NONE', #7307, 1000.000000000000000 ) ;
#75324=CARTESIAN_POINT ( 'NONE',  ( -6.802569982901797644E-16, 69.84999999999999432, -118.5560000000000116 ) ) ;
#75331=PRODUCT ( 'Pneumatic Workpiece Fixture Plate', 'Pneumatic Workpiece Fixture Plate', '', ( #82197 ) ) ;
#75359=CARTESIAN_POINT ( 'NONE',  ( -130.5461193570662317, 95.14808745951974345, -1.659440300507330157 ) ) ;
#75362=VECTOR ( 'NONE', #7411, 1000.000000000000000 ) ;
#75372=LINE ( 'NONE', #12246, #15654 ) ;
#75374=COLOUR_RGB ( '', 0.08235294, 0.09019608, 0.10196078) ;
#75376=CIRCLE ( 'NONE', #29019, 118.5560000000000116 ) ;
#75447=ORIENTED_EDGE ( 'NONE', *, *, #62105, .T. ) ;
#75462=ORIENTED_EDGE ( 'NONE', *, *, #30467, .F. ) ;
#75463=CARTESIAN_POINT ( 'NONE',  ( -79.20758933349353015, 71.53193882405241766, -88.21655330423251939 ) ) ;
#75479=AXIS2_PLACEMENT_3D ( 'NONE', #6908, #84128, #77300 ) ;
#75486=CARTESIAN_POINT ( 'NONE',  ( 0.000000000000000000, 92.07499999999998863, 0.000000000000000000 ) ) ;
#75503=CARTESIAN_POINT ( 'NONE',  ( -100.8082743238001200, 80.89704698943971550, 82.96136257730093178 ) ) ;
#75524=CARTESIAN_POINT ( 'NONE',  ( -91.12742965731001732, 69.93364840292896645, -93.49502539975229354 ) ) ;
#75530=ORIENTED_EDGE ( 'NONE', *, *, #55309, .F. ) ;
#75534=ORIENTED_EDGE ( 'NONE', *, *, #3664, .T. ) ;
#75538=ADVANCED_FACE ( 'NONE', ( #87863 ), #61480, .F. ) ;
#75553=CARTESIAN_POINT ( 'NONE',  ( 12.37521547983011239, 85.43365698736771208, 117.9083787315452270 ) ) ;
#75556=DIRECTION ( 'NONE',  ( 0.000000000000000000, -1.000000000000000000, 0.000000000000000000 ) ) ;
#75578=CARTESIAN_POINT ( 'NONE',  ( 100.8961411191535973, 127.0000000000000000, 3.968750000000400124 ) ) ;
#75590=VERTEX_POINT ( 'NONE', #42819 ) ;
#75597=AXIS2_PLACEMENT_3D ( 'NONE', #8776, #22853, #15130 ) ;
#75598=DIRECTION ( 'NONE',  ( -1.000000000000000000, 0.000000000000000000, -3.491483361109379305E-15 ) ) ;
#75615=CARTESIAN_POINT ( 'NONE',  ( -78.16952835488679341, 72.45860812971083931, 89.13771950014329093 ) ) ;
#75639=CARTESIAN_POINT ( 'NONE',  ( -91.13664476550682991, 95.14808745951974345, -93.48344774443309291 ) ) ;
#75647=VECTOR ( 'NONE', #44956, 1000.000000000000000 ) ;
#75649=ORIENTED_EDGE ( 'NONE', *, *, #64093, .T. ) ;
#75655=AXIS2_PLACEMENT_3D ( 'NONE', #40489, #13242, #6865 ) ;
#75673=CARTESIAN_POINT ( 'NONE',  ( 130.3267157422428113, 72.47310549519059464, 7.740869983443941393 ) ) ;
#75688=DIRECTION ( 'NONE',  ( 0.000000000000000000, 1.000000000000000000, 0.000000000000000000 ) ) ;
#75690=VERTEX_POINT ( 'NONE', #48283 ) ;
#75710=ORIENTED_EDGE ( 'NONE', *, *, #12679, .T. ) ;
#75730=LINE ( 'NONE', #83009, #79228 ) ;
#75759=LINE ( 'NONE', #63814, #13594 ) ;
#75762=EDGE_LOOP ( 'NONE', ( #28321, #82879, #1251, #6538 ) ) ;
#75772=ADVANCED_FACE ( 'NONE', ( #58687 ), #51424, .T. ) ;
#75801=CIRCLE ( 'NONE', #45299, 25.39999999999999858 ) ;
#75804=ORIENTED_EDGE ( 'NONE', *, *, #47415, .F. ) ;
#75806=CARTESIAN_POINT ( 'NONE',  ( 89.08909376919952194, 70.66229531820914644, 95.43663006862890086 ) ) ;
#75809=ORIENTED_EDGE ( 'NONE', *, *, #64146, .T. ) ;
#75816=CARTESIAN_POINT ( 'NONE',  ( 85.52787878288724244, 91.23859726994545838, -98.64044413062958938 ) ) ;
#75844=CARTESIAN_POINT ( 'NONE',  ( -118.1932448497438202, 91.23868085022589014, 9.271905035165794118 ) ) ;
#75847=CARTESIAN_POINT ( 'NONE',  ( 90.32738470895340299, 74.16215221268208779, -76.79083731950171909 ) ) ;
#75875=AXIS2_PLACEMENT_3D ( 'NONE', #78731, #73215, #51863 ) ;
#75878=FACE_OUTER_BOUND ( 'NONE', #80296, .T. ) ;
#75885=CARTESIAN_POINT ( 'NONE',  ( 130.3273610158207418, 92.64237678566784950, -7.754451942556684685 ) ) ;
#75901=ORIENTED_EDGE ( 'NONE', *, *, #80925, .T. ) ;
#75916=CARTESIAN_POINT ( 'NONE',  ( 98.26026929335873206, 73.28356282573679437, -85.96437953530649168 ) ) ;
#75920=CARTESIAN_POINT ( 'NONE',  ( 71.77848634863140376, 120.6499999999999915, -77.39114642429929347 ) ) ;
#75927=LINE ( 'NONE', #13698, #29154 ) ;
#75941=PLANE ( 'NONE',  #64944 ) ;
#75942=DIRECTION ( 'NONE',  ( 0.000000000000000000, 0.000000000000000000, -1.000000000000000000 ) ) ;
#75946=CARTESIAN_POINT ( 'NONE',  ( -87.44698480207762259, 71.76234181793739708, 96.94335780202351316 ) ) ;
#75952=DIRECTION ( 'NONE',  ( 0.000000000000000000, 0.000000000000000000, 1.000000000000000000 ) ) ;
#75959=LINE ( 'NONE', #83232, #6633 ) ;
#75965=ORIENTED_EDGE ( 'NONE', *, *, #57993, .T. ) ;
#75968=CARTESIAN_POINT ( 'NONE',  ( 72.96458098368650269, 127.0000000000000000, 72.96458098368729850 ) ) ;
#75969=CARTESIAN_POINT ( 'NONE',  ( -87.71185091857921634, 93.94641470820117490, -79.76397050720419202 ) ) ;
#75974=CYLINDRICAL_SURFACE ( 'NONE', #29166, 5.041900000000001825 ) ;
#75977=CARTESIAN_POINT ( 'NONE',  ( -68.91674821478409285, 82.54999999999999716, -68.91674821478481761 ) ) ;
#75984=ADVANCED_FACE ( 'NONE', ( #23604 ), #30401, .F. ) ;
#75989=DIRECTION ( 'NONE',  ( -1.000000000000000000, 0.000000000000000000, -6.982966722218760189E-15 ) ) ;
#75991=ORIENTED_EDGE ( 'NONE', *, *, #24068, .F. ) ;
#76006=AXIS2_PLACEMENT_3D ( 'NONE', #50824, #78994, #29050 ) ;
#76012=LINE ( 'NONE', #34221, #60916 ) ;
#76036=ORIENTED_EDGE ( 'NONE', *, *, #17476, .T. ) ;
#76046=CARTESIAN_POINT ( 'NONE',  ( -77.01855645442535092, 73.86197090048098346, 90.13186587200978295 ) ) ;
#76070=CARTESIAN_POINT ( 'NONE',  ( -94.33669211993698411, 94.92443974548201879, -90.25311968877646507 ) ) ;
#76074=VECTOR ( 'NONE', #6435, 1000.000000000000000 ) ;
#76109=VERTEX_POINT ( 'NONE', #31277 ) ;
#76114=ADVANCED_FACE ( 'NONE', ( #78576 ), #52587, .F. ) ;
#76129=CARTESIAN_POINT ( 'NONE',  ( -3.968750000000754508, 120.6499999999999915, 100.8961411191535973 ) ) ;
#76138=DIRECTION ( 'NONE',  ( 0.000000000000000000, 1.000000000000000000, 0.000000000000000000 ) ) ;
#76146=CIRCLE ( 'NONE', #34115, 7.937500000000000000 ) ;
#76184=CYLINDRICAL_SURFACE ( 'NONE', #35409, 5.041900000000000048 ) ;
#76202=AXIS2_PLACEMENT_3D ( 'NONE', #65379, #9974, #71316 ) ;
#76215=ORIENTED_EDGE ( 'NONE', *, *, #37483, .F. ) ;
#76220=VERTEX_POINT ( 'NONE', #678 ) ;
#76237=CARTESIAN_POINT ( 'NONE',  ( 12.70000000000000107, 82.54999999999999716, -97.46299999999996544 ) ) ;
#76248=CARTESIAN_POINT ( 'NONE',  ( 99.33321048326423863, 75.15271101351808625, 84.72210942532007039 ) ) ;
#76254=VERTEX_POINT ( 'NONE', #48805 ) ;
#76263=CARTESIAN_POINT ( 'NONE',  ( 92.12448541806557500, 79.66685870724428753, 74.62312585591683955 ) ) ;
#76284=EDGE_CURVE ( 'NONE', #32868, #32236, #61221, .T. ) ;
#76287=AXIS2_PLACEMENT_3D ( 'NONE', #68469, #7141, #19870 ) ;
#76288=CARTESIAN_POINT ( 'NONE',  ( -92.22587532767808227, 84.62843115047674303, 74.49778344313872935 ) ) ;
#76291=CARTESIAN_POINT ( 'NONE',  ( -118.5108459337403843, 94.82191660594813243, 3.295896443149240351 ) ) ;
#76294=CARTESIAN_POINT ( 'NONE',  ( 79.21825297796463872, 71.54629894495526798, -88.20503424218246380 ) ) ;
#76309=CARTESIAN_POINT ( 'NONE',  ( 79.76397050720444781, 93.94641470820114648, -87.71185091857894633 ) ) ;
#76334=CIRCLE ( 'NONE', #40074, 5.041900000000000048 ) ;
#76347=CARTESIAN_POINT ( 'NONE',  ( -86.67734222162535218, 70.52090377575436264, -80.88709205069426389 ) ) ;
#76356=VECTOR ( 'NONE', #37792, 1000.000000000000000 ) ;
#76365=CARTESIAN_POINT ( 'NONE',  ( 86.19129576945162796, 72.98383416765814502, -98.06260288352355303 ) ) ;
#76367=CARTESIAN_POINT ( 'NONE',  ( 117.8738102209306362, 82.54999999999999716, 12.70000000000123386 ) ) ;
#76372=CARTESIAN_POINT ( 'NONE',  ( 12.37563412544579045, 79.66819247178165142, 117.9083347083516173 ) ) ;
#76412=CARTESIAN_POINT ( 'NONE',  ( -92.32962665258509105, 83.38952084682850341, -74.36911441044763649 ) ) ;
#76415=VECTOR ( 'NONE', #77335, 1000.000000000000000 ) ;
#76431=CIRCLE ( 'NONE', #89478, 5.041900000000001825 ) ;
#76436=CARTESIAN_POINT ( 'NONE',  ( 0.000000000000000000, 101.5999999999999943, 0.000000000000000000 ) ) ;
#76444=LINE ( 'NONE', #14227, #62962 ) ;
#76463=DIRECTION ( 'NONE',  ( 0.000000000000000000, 0.000000000000000000, 1.000000000000000000 ) ) ;
#76471=DIRECTION ( 'NONE',  ( -6.982966722218760189E-15, 0.000000000000000000, 1.000000000000000000 ) ) ;
#76511=CYLINDRICAL_SURFACE ( 'NONE', #69773, 5.041900000000001825 ) ;
#76519=ORIENTED_EDGE ( 'NONE', *, *, #9559, .T. ) ;
#76521=CARTESIAN_POINT ( 'NONE',  ( 6.720195294977327372, 71.76561749959921599, 130.3833905926466628 ) ) ;
#76526=EDGE_CURVE ( 'NONE', #1241, #77970, #32219, .T. ) ;
#76544=AXIS2_PLACEMENT_3D ( 'NONE', #84408, #36692, #28978 ) ;
#76547=ORIENTED_EDGE ( 'NONE', *, *, #9703, .F. ) ;
#76550=CARTESIAN_POINT ( 'NONE',  ( 0.000000000000000000, 125.7300000000000040, 9.525000000000000355 ) ) ;
#76554=EDGE_CURVE ( 'NONE', #84986, #28006, #34874, .T. ) ;
#76563=DIRECTION ( 'NONE',  ( -0.8660254037844379305, 0.000000000000000000, 0.5000000000000011102 ) ) ;
#76565=CARTESIAN_POINT ( 'NONE',  ( 130.5149182481443688, 70.27892663483460467, -3.298988752045384221 ) ) ;
#76578=CARTESIAN_POINT ( 'NONE',  ( -72.96458098368751166, 127.0000000000000000, 72.96458098368620426 ) ) ;
#76582=CYLINDRICAL_SURFACE ( 'NONE', #4559, 9.525000000000000355 ) ;
#76602=DIRECTION ( 'NONE',  ( -0.7071067811865441310, 0.000000000000000000, -0.7071067811865510144 ) ) ;
#76626=CARTESIAN_POINT ( 'NONE',  ( 86.68005309089053867, 92.64985122628469583, 97.63151088911791931 ) ) ;
#76633=VERTEX_POINT ( 'NONE', #51179 ) ;
#76650=CARTESIAN_POINT ( 'NONE',  ( -7.746212673614270905, 92.64801822704207268, 118.3046725678181872 ) ) ;
#76653=AXIS2_PLACEMENT_3D ( 'NONE', #44629, #18725, #51441 ) ;
#76661=DIRECTION ( 'NONE',  ( 0.000000000000000000, 1.000000000000000000, 0.000000000000000000 ) ) ;
#76674=ADVANCED_FACE ( 'NONE', ( #8986, #24392, #85743, #64386, #64829, #15795, #50745, #38015, #65708, #71654 ), #38442, .T. ) ;
#76702=CARTESIAN_POINT ( 'NONE',  ( 91.12742965730937783, 69.93364840292896645, 93.49502539975293303 ) ) ;
#76712=DIRECTION ( 'NONE',  ( 0.000000000000000000, 0.000000000000000000, -1.000000000000000000 ) ) ;
#76722=CIRCLE ( 'NONE', #67960, 7.937500000000000000 ) ;
#76737=CARTESIAN_POINT ( 'NONE',  ( -105.4788588808464027, 120.6499999999999915, 3.968749999998844924 ) ) ;
#76743=CARTESIAN_POINT ( 'NONE',  ( 83.24493215373414046, 69.84937538953985836, -84.41866557162641982 ) ) ;
#76746=FACE_OUTER_BOUND ( 'NONE', #10627, .T. ) ;
#76754=CARTESIAN_POINT ( 'NONE',  ( 0.000000000000000000, 124.5870000000000033, 0.000000000000000000 ) ) ;
#76767=EDGE_LOOP ( 'NONE', ( #67484, #11837, #13646, #82194, #74643, #53429, #45256, #11175, #44634, #38332, #25592, #25460, #49, #42441, #72931, #12074 ) ) ;
#76770=CARTESIAN_POINT ( 'NONE',  ( -77.39114642430010349, 120.6499999999999915, 71.77848634863050847 ) ) ;
#76784=AXIS2_PLACEMENT_3D ( 'NONE', #10367, #44875, #9929 ) ;
#76793=ORIENTED_EDGE ( 'NONE', *, *, #56252, .T. ) ;
#76798=ADVANCED_FACE ( 'NONE', ( #2161, #29871 ), #87955, .F. ) ;
#76812=CARTESIAN_POINT ( 'NONE',  ( 96.71266027437765445, 71.53177522571071734, -87.70409100286326520 ) ) ;
#76814=CARTESIAN_POINT ( 'NONE',  ( 103.1875000000000000, 127.0000000000000000, -7.143749999999640110 ) ) ;
#76820=CARTESIAN_POINT ( 'NONE',  ( 10.08473622792051039, 74.81935728795534146, 118.1266015380916912 ) ) ;
#76836=DIRECTION ( 'NONE',  ( 1.047445008332813989E-14, 0.000000000000000000, -1.000000000000000000 ) ) ;
#76854=LINE ( 'NONE', #35500, #40077 ) ;
#76865=CARTESIAN_POINT ( 'NONE',  ( -80.04418453221599350, 94.12556101775332706, -87.45628510944642642 ) ) ;
#76872=ORIENTED_EDGE ( 'NONE', *, *, #66652, .F. ) ;
#76890=CARTESIAN_POINT ( 'NONE',  ( 6.710838307577478012, 93.34022857041041732, 118.3664257206621357 ) ) ;
#76893=CARTESIAN_POINT ( 'NONE',  ( -72.96458098368600531, 117.4749999999999943, -72.96458098368781009 ) ) ;
#76899=DIRECTION ( 'NONE',  ( 0.000000000000000000, 1.000000000000000000, 0.000000000000000000 ) ) ;
#76902=AXIS2_PLACEMENT_3D ( 'NONE', #70919, #29128, #35468 ) ;
#76922=CARTESIAN_POINT ( 'NONE',  ( 5.624880194777466258, 93.94404932077411274, -118.4230601929072435 ) ) ;
#76924=CARTESIAN_POINT ( 'NONE',  ( -11.00078833628931818, 88.90974477516434149, 130.0918550420129236 ) ) ;
#76930=CARTESIAN_POINT ( 'NONE',  ( -105.4788588808462038, 127.0000000000000000, -3.968750000001139977 ) ) ;
#76951=CARTESIAN_POINT ( 'NONE',  ( -84.43201024598403137, 69.85063172184841562, 83.23139715273285333 ) ) ;
#76962=CARTESIAN_POINT ( 'NONE',  ( -103.1875000000000000, 117.4749999999999943, -7.937500000001080913 ) ) ;
#76963=EDGE_CURVE ( 'NONE', #6159, #29190, #84710, .T. ) ;
#76985=EDGE_CURVE ( 'NONE', #8401, #82562, #26130, .T. ) ;
#76987=VERTEX_POINT ( 'NONE', #29764 ) ;
#76988=EDGE_LOOP ( 'NONE', ( #6268, #22529, #63354, #18607 ) ) ;
#77000=EDGE_CURVE ( 'NONE', #83000, #52485, #72434, .T. ) ;
#77024=EDGE_CURVE ( 'NONE', #1670, #14963, #64287, .T. ) ;
#77036=FACE_OUTER_BOUND ( 'NONE', #57457, .T. ) ;
#77041=DIRECTION ( 'NONE',  ( 0.000000000000000000, -1.000000000000000000, 0.000000000000000000 ) ) ;
#77079=CARTESIAN_POINT ( 'NONE',  ( 100.6521573293557452, 85.43248893795416166, 83.15057989155073415 ) ) ;
#77103=ORIENTED_EDGE ( 'NONE', *, *, #56743, .T. ) ;
#77123=CARTESIAN_POINT ( 'NONE',  ( 0.000000000000000000, 127.0000000000000000, 0.000000000000000000 ) ) ;
#77134=CARTESIAN_POINT ( 'NONE',  ( 72.96458098368701428, 101.5999999999999943, -67.92268098368680285 ) ) ;
#77140=FACE_BOUND ( 'NONE', #15021, .T. ) ;
#77154=CARTESIAN_POINT ( 'NONE',  ( 99.78212687779678447, 76.18750001922980175, 84.19388261208071356 ) ) ;
#77163=ORIENTED_EDGE ( 'NONE', *, *, #39832, .T. ) ;
#77164=ORIENTED_EDGE ( 'NONE', *, *, #10823, .F. ) ;
#77189=EDGE_LOOP ( 'NONE', ( #57697, #71053, #17059, #8271 ) ) ;
#77193=ORIENTED_EDGE ( 'NONE', *, *, #62567, .F. ) ;
#77194=ORIENTED_EDGE ( 'NONE', *, *, #4797, .T. ) ;
#77195=CARTESIAN_POINT ( 'NONE',  ( -74.70172715947499853, 85.83559868056558173, 92.06080542007487111 ) ) ;
#77198=CARTESIAN_POINT ( 'NONE',  ( -118.3041687469093830, 92.64232203292144163, 7.754495127085286654 ) ) ;
#77201=CARTESIAN_POINT ( 'NONE',  ( 74.89042153202936447, 78.46643079253871633, -91.90737012895618818 ) ) ;
#77223=ORIENTED_EDGE ( 'NONE', *, *, #20593, .F. ) ;
#77248=CARTESIAN_POINT ( 'NONE',  ( -74.36911441044668436, 82.54999999999999716, -92.32962665258587265 ) ) ;
#77259=FACE_OUTER_BOUND ( 'NONE', #46139, .T. ) ;
#77270=VECTOR ( 'NONE', #12597, 1000.000000000000000 ) ;
#77291=PLANE ( 'NONE',  #41847 ) ;
#77297=VECTOR ( 'NONE', #33555, 1000.000000000000000 ) ;
#77300=DIRECTION ( 'NONE',  ( 0.000000000000000000, 0.000000000000000000, -1.000000000000000000 ) ) ;
#77301=AXIS2_PLACEMENT_3D ( 'NONE', #81518, #81961, #40598 ) ;
#77307=ADVANCED_FACE ( 'NONE', ( #63266 ), #55976, .F. ) ;
#77313=CARTESIAN_POINT ( 'NONE',  ( -79.21650378603835918, 93.55239623846826191, -88.20661029664601926 ) ) ;
#77335=DIRECTION ( 'NONE',  ( -1.000000000000000000, 0.000000000000000000, -7.067626426349370916E-15 ) ) ;
#77353=CARTESIAN_POINT ( 'NONE',  ( 3.968750000000050182, 120.6499999999999915, -100.8961411191535973 ) ) ;
#77365=CARTESIAN_POINT ( 'NONE',  ( 5.244287019405557082, 94.12413552026931995, -118.4405785268131552 ) ) ;
#77372=EDGE_CURVE ( 'NONE', #12421, #39347, #52554, .T. ) ;
#77410=CARTESIAN_POINT ( 'NONE',  ( 3.110602869834275287E-15, 124.5870000000000033, 25.39999999999999858 ) ) ;
#77420=CARTESIAN_POINT ( 'NONE',  ( 12.70000000000000107, 82.54999999999999716, 129.9368274816650910 ) ) ;
#77421=CARTESIAN_POINT ( 'NONE',  ( -100.6521573293563279, 85.43248893795414745, -83.15057989155002360 ) ) ;
#77431=VERTEX_POINT ( 'NONE', #10878 ) ;
#77433=LINE ( 'NONE', #56975, #51992 ) ;
#77445=ORIENTED_EDGE ( 'NONE', *, *, #34718, .F. ) ;
#77458=CARTESIAN_POINT ( 'NONE',  ( -12.70000000000000107, 82.54999999999999716, -97.46299999999996544 ) ) ;
#77461=CARTESIAN_POINT ( 'NONE',  ( 129.9368274816649489, 82.54999999999999716, 12.70000000000136176 ) ) ;
#77475=DIRECTION ( 'NONE',  ( 0.000000000000000000, 0.000000000000000000, 1.000000000000000000 ) ) ;
#77477=CARTESIAN_POINT ( 'NONE',  ( -103.1875000000000000, 117.4749999999999943, -1.080832317973422076E-12 ) ) ;
#77480=PLANE ( 'NONE',  #30043 ) ;
#77517=ORIENTED_EDGE ( 'NONE', *, *, #12052, .T. ) ;
#77518=AXIS2_PLACEMENT_3D ( 'NONE', #86878, #87323, #58268 ) ;
#77524=CARTESIAN_POINT ( 'NONE',  ( 82.89895571708156297, 82.54999999999999716, 100.8594679592221155 ) ) ;
#77545=CARTESIAN_POINT ( 'NONE',  ( -7.205548786489490269E-13, 117.4749999999999943, 103.1875000000000000 ) ) ;
#77558=CARTESIAN_POINT ( 'NONE',  ( 12.03133265694088294, 78.46222587235902779, -117.9439990761035943 ) ) ;
#77607=EDGE_CURVE ( 'NONE', #9436, #9318, #88542, .T. ) ;
#77612=DIRECTION ( 'NONE',  ( 0.000000000000000000, 0.000000000000000000, 1.000000000000000000 ) ) ;
#77619=ORIENTED_EDGE ( 'NONE', *, *, #76284, .T. ) ;
#77623=VECTOR ( 'NONE', #47055, 1000.000000000000000 ) ;
#77636=CARTESIAN_POINT ( 'NONE',  ( -91.50010255991617214, 88.17653575778739139, 75.38763434846499933 ) ) ;
#77645=CARTESIAN_POINT ( 'NONE',  ( 75.37281393334508550, 76.91656954603719498, -91.51265874544250778 ) ) ;
#77659=CARTESIAN_POINT ( 'NONE',  ( 0.000000000000000000, 61.59999999999999432, 0.000000000000000000 ) ) ;
#77662=CARTESIAN_POINT ( 'NONE',  ( 88.44409384119012429, 93.33902940301966566, -78.95116244206050737 ) ) ;
#77685=AXIS2_PLACEMENT_3D ( 'NONE', #17351, #72760, #63373 ) ;
#77711=AXIS2_PLACEMENT_3D ( 'NONE', #22679, #85363, #78091 ) ;
#77719=CARTESIAN_POINT ( 'NONE',  ( 95.43663006862857401, 70.66229531820914644, -89.08909376919980616 ) ) ;
#77744=CARTESIAN_POINT ( 'NONE',  ( -72.96458098368600531, 127.0000000000000000, -72.96458098368781009 ) ) ;
#77763=CARTESIAN_POINT ( 'NONE',  ( -83.15048135366454574, 79.66749569656610674, -100.6522392491101954 ) ) ;
#77770=CARTESIAN_POINT ( 'NONE',  ( 71.77848634863079269, 120.6499999999999915, 77.39114642429989033 ) ) ;
#77777=VECTOR ( 'NONE', #14181, 1000.000000000000114 ) ;
#77779=ORIENTED_EDGE ( 'NONE', *, *, #89703, .F. ) ;
#77785=CARTESIAN_POINT ( 'NONE',  ( -33.98325472291460159, 111.1250000000000000, -3.175000000000234746 ) ) ;
#77818=CARTESIAN_POINT ( 'NONE',  ( -77.39114642429849766, 120.6499999999999915, -71.77848634863219957 ) ) ;
#77844=VERTEX_POINT ( 'NONE', #15814 ) ;
#77864=LINE ( 'NONE', #69702, #12814 ) ;
#77873=ORIENTED_EDGE ( 'NONE', *, *, #25032, .T. ) ;
#77896=VECTOR ( 'NONE', #78021, 1000.000000000000000 ) ;
#77918=CARTESIAN_POINT ( 'NONE',  ( -130.4363378768870234, 71.14122173980734942, -5.641126054320938721 ) ) ;
#77927=DIRECTION ( 'NONE',  ( 0.9659258262890688673, 0.000000000000000000, -0.2588190451025189631 ) ) ;
#77928=CARTESIAN_POINT ( 'NONE',  ( -72.96458098368751166, 127.0000000000000000, 72.96458098368620426 ) ) ;
#77929=DIRECTION ( 'NONE',  ( -0.9659258262890675351, 0.000000000000000000, -0.2588190451025234595 ) ) ;
#77954=PLANE ( 'NONE',  #68517 ) ;
#77970=VERTEX_POINT ( 'NONE', #45275 ) ;
#77978=CARTESIAN_POINT ( 'NONE',  ( 99.33304294513213506, 89.94765885072628464, 84.72230615113687691 ) ) ;
#77979=CARTESIAN_POINT ( 'NONE',  ( 4.481506956522084195, 70.65969245518890318, -130.4796279538066983 ) ) ;
#77992=EDGE_CURVE ( 'NONE', #19337, #9633, #37596, .T. ) ;
#77993=EDGE_CURVE ( 'NONE', #81147, #65492, #72114, .T. ) ;
#78012=ORIENTED_EDGE ( 'NONE', *, *, #83933, .T. ) ;
#78021=DIRECTION ( 'NONE',  ( 0.000000000000000000, -1.000000000000000000, 0.000000000000000000 ) ) ;
#78072=PLANE ( 'NONE',  #51083 ) ;
#78074=CYLINDRICAL_SURFACE ( 'NONE', #86711, 12.70000000000000107 ) ;
#78080=ORIENTED_EDGE ( 'NONE', *, *, #43934, .F. ) ;
#78091=DIRECTION ( 'NONE',  ( 0.000000000000000000, 0.000000000000000000, -1.000000000000000000 ) ) ;
#78094=CARTESIAN_POINT ( 'NONE',  ( -74.36911441044735227, 83.38952084682851762, 92.32962665258540369 ) ) ;
#78103=CARTESIAN_POINT ( 'NONE',  ( 91.50401754987822756, 76.93600387762165838, -75.38287938184973314 ) ) ;
#78122=AXIS2_PLACEMENT_3D ( 'NONE', #63165, #64521, #44499 ) ;
#78128=ORIENTED_EDGE ( 'NONE', *, *, #82554, .T. ) ;
#78131=ORIENTED_EDGE ( 'NONE', *, *, #69822, .T. ) ;
#78156=LINE ( 'NONE', #79039, #59187 ) ;
#78172=DIRECTION ( 'NONE',  ( 0.000000000000000000, 1.000000000000000000, 0.000000000000000000 ) ) ;
#78193=DIRECTION ( 'NONE',  ( 0.000000000000000000, 0.000000000000000000, 1.000000000000000000 ) ) ;
#78196=DIRECTION ( 'NONE',  ( -0.7071067811865439090, 0.000000000000000000, -0.7071067811865512365 ) ) ;
#78200=EDGE_LOOP ( 'NONE', ( #55938, #7993 ) ) ;
#78214=CARTESIAN_POINT ( 'NONE',  ( -92.89936586971981569, 95.23006786499111342, 91.73195104381176179 ) ) ;
#78220=CARTESIAN_POINT ( 'NONE',  ( 4.163101094985349692E-14, 120.6499999999999915, -98.60478223830740774 ) ) ;
#78232=DIRECTION ( 'NONE',  ( 0.000000000000000000, 0.000000000000000000, -1.000000000000000000 ) ) ;
#78236=AXIS2_PLACEMENT_3D ( 'NONE', #8167, #45228, #86597 ) ;
#78288=FACE_OUTER_BOUND ( 'NONE', #37982, .T. ) ;
#78289=AXIS2_PLACEMENT_3D ( 'NONE', #48405, #76138, #33461 ) ;
#78298=AXIS2_PLACEMENT_3D ( 'NONE', #2033, #57428, #3809 ) ;
#78301=DIRECTION ( 'NONE',  ( 0.000000000000000000, 1.000000000000000000, 0.000000000000000000 ) ) ;
#78310=CARTESIAN_POINT ( 'NONE',  ( -59.93649209371488951, 82.54999999999999716, -77.89700433585392148 ) ) ;
#78314=CARTESIAN_POINT ( 'NONE',  ( -72.96458098368751166, 127.0000000000000000, 67.92268098368620599 ) ) ;
#78319=CARTESIAN_POINT ( 'NONE',  ( -7.205548786489490269E-13, 127.0000000000000000, 96.04375000000000284 ) ) ;
#78325=EDGE_CURVE ( 'NONE', #61270, #6171, #6286, .T. ) ;
#78329=EDGE_CURVE ( 'NONE', #43857, #74189, #47950, .T. ) ;
#78337=CARTESIAN_POINT ( 'NONE',  ( 0.8390482630167189759, 69.85000000000000853, 130.5560000000000400 ) ) ;
#78378=CARTESIAN_POINT ( 'NONE',  ( -130.4354319819074703, 71.15434825076370373, 5.621545387653513970 ) ) ;
#78395=AXIS2_PLACEMENT_3D ( 'NONE', #77928, #64297, #43377 ) ;
#78406=PLANE ( 'NONE',  #57583 ) ;
#78409=CARTESIAN_POINT ( 'NONE',  ( -7.205548786489490269E-13, 117.4749999999999943, 111.1250000000000000 ) ) ;
#78413=VERTEX_POINT ( 'NONE', #717 ) ;
#78416=ORIENTED_EDGE ( 'NONE', *, *, #22118, .F. ) ;
#78451=CARTESIAN_POINT ( 'NONE',  ( 12.70000000000000107, 82.54999999999999716, -129.9368274816650910 ) ) ;
#78461=CARTESIAN_POINT ( 'NONE',  ( -76.20505178924278766, 120.6499999999999915, -76.20505178924469192 ) ) ;
#78487=DIRECTION ( 'NONE',  ( 0.000000000000000000, 0.000000000000000000, -1.000000000000000000 ) ) ;
#78492=ADVANCED_FACE ( 'NONE', ( #23430 ), #17043, .F. ) ;
#78522=CARTESIAN_POINT ( 'NONE',  ( 129.9368274816649489, 82.54999999999999716, 12.70000000000136176 ) ) ;
#78527=EDGE_CURVE ( 'NONE', #6249, #82562, #58794, .T. ) ;
#78531=AXIS2_PLACEMENT_3D ( 'NONE', #66916, #6479, #81021 ) ;
#78536=ORIENTED_EDGE ( 'NONE', *, *, #48644, .T. ) ;
#78548=DIRECTION ( 'NONE',  ( 0.000000000000000000, -1.000000000000000000, 0.000000000000000000 ) ) ;
#78551=CARTESIAN_POINT ( 'NONE',  ( -74.15067561874160162, 127.0000000000000000, -68.53801554307528932 ) ) ;
#78576=FACE_OUTER_BOUND ( 'NONE', #82812, .T. ) ;
#78581=LINE ( 'NONE', #15891, #54017 ) ;
#78605=DIRECTION ( 'NONE',  ( 0.000000000000000000, 0.000000000000000000, 1.000000000000000000 ) ) ;
#78607=DIRECTION ( 'NONE',  ( 0.2588190451025236261, 0.000000000000000000, -0.9659258262890675351 ) ) ;
#78627=EDGE_CURVE ( 'NONE', #64886, #66793, #71660, .T. ) ;
#78629=DIRECTION ( 'NONE',  ( 0.000000000000000000, 1.000000000000000000, 0.000000000000000000 ) ) ;
#78636=CARTESIAN_POINT ( 'NONE',  ( 100.5986936721446341, 85.85000629251469206, -83.21537498883944295 ) ) ;
#78665=AXIS2_PLACEMENT_3D ( 'NONE', #47028, #67946, #21151 ) ;
#78678=ORIENTED_EDGE ( 'NONE', *, *, #24695, .T. ) ;
#78685=AXIS2_PLACEMENT_3D ( 'NONE', #89351, #5328, #12140 ) ;
#78704=EDGE_CURVE ( 'NONE', #68783, #3990, #13613, .T. ) ;
#78722=EDGE_LOOP ( 'NONE', ( #36794, #27554 ) ) ;
#78731=CARTESIAN_POINT ( 'NONE',  ( 0.000000000000000000, 198.8420489685532004, 0.000000000000000000 ) ) ;
#78772=LINE ( 'NONE', #36962, #46659 ) ;
#78774=AXIS2_PLACEMENT_3D ( 'NONE', #17512, #64770, #3435 ) ;
#78778=ORIENTED_EDGE ( 'NONE', *, *, #12052, .F. ) ;
#78802=CARTESIAN_POINT ( 'NONE',  ( 103.1875000000000000, 117.4749999999999943, -7.143749999999640110 ) ) ;
#78833=EDGE_CURVE ( 'NONE', #73407, #84780, #70359, .T. ) ;
#78848=CARTESIAN_POINT ( 'NONE',  ( -68.53801554307499089, 120.6499999999999915, 74.15067561874188584 ) ) ;
#78859=EDGE_LOOP ( 'NONE', ( #26516, #12192, #34554, #31551 ) ) ;
#78862=CARTESIAN_POINT ( 'NONE',  ( -4.867771054587870516, 94.30191638479371363, -130.4669033451686175 ) ) ;
#78870=VERTEX_POINT ( 'NONE', #43273 ) ;
#78871=VERTEX_POINT ( 'NONE', #30112 ) ;
#78872=EDGE_LOOP ( 'NONE', ( #48797, #3149, #25215, #49712 ) ) ;
#78889=AXIS2_PLACEMENT_3D ( 'NONE', #19995, #6357, #61751 ) ;
#78921=ORIENTED_EDGE ( 'NONE', *, *, #1494, .T. ) ;
#78923=ORIENTED_EDGE ( 'NONE', *, *, #51847, .T. ) ;
#78939=CARTESIAN_POINT ( 'NONE',  ( -103.1875000000000000, 127.0000000000000000, 5.041899999998910253 ) ) ;
#78951=DIRECTION ( 'NONE',  ( 0.000000000000000000, 1.000000000000000000, 0.000000000000000000 ) ) ;
#78960=B_SPLINE_CURVE_WITH_KNOTS ( 'NONE', 3,
 ( #72846, #23820, #32384, #30623, #79239, #58323, #10611, #16998, #66017, #24696, #52363, #80126, #45552, #73283, #73737, #11059, #4255, #59642, #25136, #52796, #39214, #33746, #81915, #81475, #75081 ),
 .UNSPECIFIED., .F., .F.,
 ( 4, 2, 2, 2, 2, 2, 2, 2, 2, 1, 2, 2, 4 ),
 ( 6.610103225985008611E-19, 0.002483982529268030041, 0.003725973793902044844, 0.004967965058536060081, 0.007451947587804091423, 0.008693938852438104492, 0.009935930117072118428, 0.01241991264634014977, 0.01366190391097416197, 0.01490389517560817417, 0.01614588644024218464, 0.01738787770487619858, 0.01987186023414422298 ),
 .UNSPECIFIED. ) ;
#78969=CARTESIAN_POINT ( 'NONE',  ( 90.13186587200897293, 73.86197090048096925, 77.01855645442628884 ) ) ;
#78974=ORIENTED_EDGE ( 'NONE', *, *, #30381, .F. ) ;
#78994=DIRECTION ( 'NONE',  ( 0.000000000000000000, 1.000000000000000000, 0.000000000000000000 ) ) ;
#79002=LINE ( 'NONE', #16770, #13995 ) ;
#79005=DIRECTION ( 'NONE',  ( 0.7071067811865536790, 0.000000000000000000, -0.7071067811865413555 ) ) ;
#79032=ORIENTED_EDGE ( 'NONE', *, *, #83123, .F. ) ;
#79039=CARTESIAN_POINT ( 'NONE',  ( -105.4788588808462038, 120.6499999999999915, -3.968750000001139977 ) ) ;
#79045=ORIENTED_EDGE ( 'NONE', *, *, #10253, .T. ) ;
#79065=ORIENTED_EDGE ( 'NONE', *, *, #50039, .F. ) ;
#79075=CARTESIAN_POINT ( 'NONE',  ( 0.000000000000000000, 101.5999999999999943, -103.1875000000000000 ) ) ;
#79076=VECTOR ( 'NONE', #63776, 1000.000000000000000 ) ;
#79094=VERTEX_POINT ( 'NONE', #4638 ) ;
#79098=DIRECTION ( 'NONE',  ( 0.5000000000000012212, 0.000000000000000000, 0.8660254037844380415 ) ) ;
#79100=CARTESIAN_POINT ( 'NONE',  ( -88.25806911646338904, 93.94653598907717651, 96.20559720633596612 ) ) ;
#79115=CIRCLE ( 'NONE', #45738, 118.5560000000000116 ) ;
#79136=EDGE_CURVE ( 'NONE', #71312, #37218, #6871, .T. ) ;
#79139=VERTEX_POINT ( 'NONE', #76367 ) ;
#79146=DIRECTION ( 'NONE',  ( -0.000000000000000000, 1.000000000000000000, -0.000000000000000000 ) ) ;
#79176=VECTOR ( 'NONE', #86453, 999.9999999999998863 ) ;
#79217=CARTESIAN_POINT ( 'NONE',  ( 118.4716181662679872, 70.66242608954388515, 4.488731742999982011 ) ) ;
#79219=DIRECTION ( 'NONE',  ( 0.000000000000000000, 1.000000000000000000, 0.000000000000000000 ) ) ;
#79223=VERTEX_POINT ( 'NONE', #9571 ) ;
#79228=VECTOR ( 'NONE', #48890, 999.9999999999998863 ) ;
#79237=EDGE_LOOP ( 'NONE', ( #26663, #9023, #15757, #33058 ) ) ;
#79239=CARTESIAN_POINT ( 'NONE',  ( -3.286821707691937711, 70.27560252132435892, 118.5111027017741776 ) ) ;
#79245=VERTEX_POINT ( 'NONE', #85886 ) ;
#79262=CARTESIAN_POINT ( 'NONE',  ( -130.1658077747427171, 74.80151635532865839, -10.09693588310369350 ) ) ;
#79275=B_SPLINE_CURVE_WITH_KNOTS ( 'NONE', 3,
 ( #59368, #52970, #4864, #45719, #66635, #46173, #67531, #33010, #87990, #4426, #32112, #73904, #65736, #32553, #60706, #11688, #60258, #39382, #25748, #88442, #74357, #12127, #39809, #26203, #44846, #89340 ),
 .UNSPECIFIED., .F., .F.,
 ( 4, 2, 2, 2, 2, 2, 2, 2, 2, 2, 2, 2, 4 ),
 ( 0.01986933033599076748, 0.02111058882927464853, 0.02235184732255853304, 0.02483436430912634024, 0.02607562280241026292, 0.02731688129569418561, 0.02979939828226199974, 0.03228191526882981388, 0.03352317376211371575, 0.03476443225539761761, 0.03724694924196542134, 0.03848820773524931627, 0.03972946622853321813 ),
 .UNSPECIFIED. ) ;
#79307=CARTESIAN_POINT ( 'NONE',  ( -0.8293186434173683841, 95.24999999999997158, -130.5560000000000116 ) ) ;
#79324=CARTESIAN_POINT ( 'NONE',  ( 1.665555919329872792, 69.93248702128259708, -130.5479027315182066 ) ) ;
#79339=DIRECTION ( 'NONE',  ( 0.000000000000000000, 1.000000000000000000, 0.000000000000000000 ) ) ;
#79374=DIRECTION ( 'NONE',  ( 0.000000000000000000, -1.000000000000000000, 0.000000000000000000 ) ) ;
#79380=CARTESIAN_POINT ( 'NONE',  ( 31.75000000000000000, 124.5870000000000033, 3.174999999999999822 ) ) ;
#79400=CARTESIAN_POINT ( 'NONE',  ( 83.90387289223293976, 76.93632333215535368, 100.0252357601330004 ) ) ;
#79403=CARTESIAN_POINT ( 'NONE',  ( 100.8082743238007595, 80.89704698943972971, -82.96136257730026387 ) ) ;
#79419=CARTESIAN_POINT ( 'NONE',  ( 75.10852726169315474, 77.68452076096552616, 91.72954497613159219 ) ) ;
#79438=LINE ( 'NONE', #78551, #33582 ) ;
#79446=CARTESIAN_POINT ( 'NONE',  ( 72.96458098368701428, 127.0000000000000000, -80.10833098368678407 ) ) ;
#79448=ADVANCED_FACE ( 'NONE', ( #67654 ), #5435, .F. ) ;
#79470=ORIENTED_EDGE ( 'NONE', *, *, #19225, .T. ) ;
#79477=DIRECTION ( 'NONE',  ( 0.000000000000000000, 0.000000000000000000, 1.000000000000000000 ) ) ;
#79522=CIRCLE ( 'NONE', #53335, 42.54500000000000171 ) ;
#79537=DIRECTION ( 'NONE',  ( 0.000000000000000000, 1.000000000000000000, 0.000000000000000000 ) ) ;
#79552=CARTESIAN_POINT ( 'NONE',  ( -103.1875000000000000, 117.4749999999999943, -1.080832317973422076E-12 ) ) ;
#79558=DIRECTION ( 'NONE',  ( 0.000000000000000000, -1.000000000000000000, 0.000000000000000000 ) ) ;
#79565=AXIS2_PLACEMENT_3D ( 'NONE', #23275, #51369, #71846 ) ;
#79574=EDGE_CURVE ( 'NONE', #78870, #75109, #70687, .T. ) ;
#79583=CIRCLE ( 'NONE', #62177, 7.143750000000001599 ) ;
#79598=CARTESIAN_POINT ( 'NONE',  ( -8.690912999409459161, 73.28018275885442279, 130.2667388509219677 ) ) ;
#79608=ORIENTED_EDGE ( 'NONE', *, *, #85477, .F. ) ;
#79662=CARTESIAN_POINT ( 'NONE',  ( 118.4231949783269897, 71.15456258041355397, -5.621971333129370585 ) ) ;
#79666=FACE_OUTER_BOUND ( 'NONE', #41075, .T. ) ;
#79670=ORIENTED_EDGE ( 'NONE', *, *, #84789, .T. ) ;
#79700=ORIENTED_EDGE ( 'NONE', *, *, #88459, .T. ) ;
#79701=VERTEX_POINT ( 'NONE', #29797 ) ;
#79715=EDGE_LOOP ( 'NONE', ( #56061, #22968 ) ) ;
#79739=CIRCLE ( 'NONE', #31851, 7.143750000000004263 ) ;
#79752=CARTESIAN_POINT ( 'NONE',  ( -12.69999999999999929, 83.38939070830898004, -129.9368274816650342 ) ) ;
#79783=DIRECTION ( 'NONE',  ( 0.000000000000000000, -1.000000000000000000, 0.000000000000000000 ) ) ;
#79823=ADVANCED_FACE ( 'NONE', ( #20188 ), #52858, .F. ) ;
#79836=VERTEX_POINT ( 'NONE', #11118 ) ;
#79845=DIRECTION ( 'NONE',  ( 1.000000000000000000, 0.000000000000000000, 1.047445008332812253E-14 ) ) ;
#79860=EDGE_CURVE ( 'NONE', #40430, #70137, #27433, .T. ) ;
#79881=CARTESIAN_POINT ( 'NONE',  ( 118.3041687469094256, 92.64232203292141321, -7.754495127084455319 ) ) ;
#79902=DIRECTION ( 'NONE',  ( 0.000000000000000000, 1.000000000000000000, 0.000000000000000000 ) ) ;
#79929=EDGE_CURVE ( 'NONE', #29190, #6159, #54001, .T. ) ;
#79953=ORIENTED_EDGE ( 'NONE', *, *, #62497, .T. ) ;
#79963=MANIFOLD_SOLID_BREP ( 'Stock-BR-Y-104-1', #63386 ) ;
#79989=CARTESIAN_POINT ( 'NONE',  ( 72.96458098368701428, 117.4749999999999943, -72.96458098368670164 ) ) ;
#79998=DIRECTION ( 'NONE',  ( 0.000000000000000000, 1.000000000000000000, 0.000000000000000000 ) ) ;
#80029=EDGE_LOOP ( 'NONE', ( #33915, #49503, #12122, #45582 ) ) ;
#80039=CARTESIAN_POINT ( 'NONE',  ( 4.163336342344339551E-14, 127.0000000000000000, -107.7702177616926065 ) ) ;
#80041=VECTOR ( 'NONE', #44833, 1000.000000000000000 ) ;
#80057=LINE ( 'NONE', #18257, #9377 ) ;
#80071=CARTESIAN_POINT ( 'NONE',  ( -7.205548786489490269E-13, 127.0000000000000000, 103.1875000000000000 ) ) ;
#80081=VERTEX_POINT ( 'NONE', #85852 ) ;
#80092=CARTESIAN_POINT ( 'NONE',  ( -83.52520760052897231, 78.07027470200927155, 100.3415888741740503 ) ) ;
#80106=CARTESIAN_POINT ( 'NONE',  ( 117.9083433361412290, 79.66725693986899159, 12.37555662352282226 ) ) ;
#80119=EDGE_CURVE ( 'NONE', #55858, #65321, #79115, .T. ) ;
#80126=CARTESIAN_POINT ( 'NONE',  ( -8.383266637423213652, 73.00087262779534569, 118.2596760195012848 ) ) ;
#80139=FACE_OUTER_BOUND ( 'NONE', #1201, .T. ) ;
#80189=EDGE_LOOP ( 'NONE', ( #27000, #15801, #52930, #28855 ) ) ;
#80201=CARTESIAN_POINT ( 'NONE',  ( -74.36911441044735227, 81.71068249639867531, 92.32962665258538948 ) ) ;
#80213=CARTESIAN_POINT ( 'NONE',  ( 0.000000000000000000, 117.4749999999999943, -103.1875000000000000 ) ) ;
#80220=CARTESIAN_POINT ( 'NONE',  ( 11.89044713366393324, 87.03112570152838146, 130.0135071244502285 ) ) ;
#80231=EDGE_LOOP ( 'NONE', ( #52516, #48139, #88976, #54062, #50362, #3726 ) ) ;
#80233=FACE_BOUND ( 'NONE', #17033, .T. ) ;
#80238=ORIENTED_EDGE ( 'NONE', *, *, #1213, .F. ) ;
#80242=ORIENTED_EDGE ( 'NONE', *, *, #70020, .T. ) ;
#80256=DIRECTION ( 'NONE',  ( 0.000000000000000000, 0.000000000000000000, 1.000000000000000000 ) ) ;
#80266=ADVANCED_FACE ( 'NONE', ( #56997 ), #36578, .F. ) ;
#80269=ORIENTED_EDGE ( 'NONE', *, *, #63736, .T. ) ;
#80296=EDGE_LOOP ( 'NONE', ( #6489, #66705, #51082, #1691 ) ) ;
#80298=AXIS2_PLACEMENT_3D ( 'NONE', #76893, #75556, #26951 ) ;
#80299=VERTEX_POINT ( 'NONE', #7516 ) ;
#80313=ORIENTED_EDGE ( 'NONE', *, *, #8150, .F. ) ;
#80319=CARTESIAN_POINT ( 'NONE',  ( 118.0058645681208702, 88.18374315479978520, -11.41243735079784472 ) ) ;
#80326=CARTESIAN_POINT ( 'NONE',  ( -71.77848634863029531, 120.6499999999999915, -77.39114642430038771 ) ) ;
#80343=ADVANCED_FACE ( 'NONE', ( #45470 ), #18237, .F. ) ;
#80346=ORIENTED_EDGE ( 'NONE', *, *, #4797, .F. ) ;
#80349=CARTESIAN_POINT ( 'NONE',  ( -118.5214325610856605, 70.17658267799285454, 2.892017926150298734 ) ) ;
#80357=EDGE_LOOP ( 'NONE', ( #6710, #65599, #1945, #45897 ) ) ;
#80363=ORIENTED_EDGE ( 'NONE', *, *, #4650, .T. ) ;
#80379=DIRECTION ( 'NONE',  ( 0.000000000000000000, 1.000000000000000000, 0.000000000000000000 ) ) ;
#80392=DIRECTION ( 'NONE',  ( 0.000000000000000000, 1.000000000000000000, 0.000000000000000000 ) ) ;
#80408=CARTESIAN_POINT ( 'NONE',  ( -11.41378189430731993, 76.91903266065129685, -118.0057337156638653 ) ) ;
#80409=EDGE_CURVE ( 'NONE', #69770, #61270, #86842, .T. ) ;
#80432=CARTESIAN_POINT ( 'NONE',  ( -72.96458098368600531, 117.4749999999999943, -72.96458098368781009 ) ) ;
#80446=CARTESIAN_POINT ( 'NONE',  ( -71.77848634863029531, 127.0000000000000000, -77.39114642430038771 ) ) ;
#80457=EDGE_CURVE ( 'NONE', #70447, #59781, #7379, .T. ) ;
#80475=LINE ( 'NONE', #18236, #88968 ) ;
#80489=CARTESIAN_POINT ( 'NONE',  ( 2.684158038187649039E-15, 69.84999999999999432, -130.5560000000000116 ) ) ;
#80496=VECTOR ( 'NONE', #34829, 1000.000000000000000 ) ;
#80497=( NAMED_UNIT ( * ) SI_UNIT ( $, .STERADIAN. ) SOLID_ANGLE_UNIT ( ) );
#80512=FACE_OUTER_BOUND ( 'NONE', #45538, .T. ) ;
#80544=CARTESIAN_POINT ( 'NONE',  ( 118.3861417219090555, 71.54629894495526798, -6.354613972968428115 ) ) ;
#80554=PLANE ( 'NONE',  #1165 ) ;
#80617=DIRECTION ( 'NONE',  ( 0.000000000000000000, 1.000000000000000000, 0.000000000000000000 ) ) ;
#80618=CARTESIAN_POINT ( 'NONE',  ( -11.41184330286787052, 88.18497404666861428, -118.0059224074909707 ) ) ;
#80629=DIRECTION ( 'NONE',  ( 0.000000000000000000, 1.000000000000000000, 0.000000000000000000 ) ) ;
#80645=DIRECTION ( 'NONE',  ( 0.000000000000000000, 1.000000000000000000, 0.000000000000000000 ) ) ;
#80659=CARTESIAN_POINT ( 'NONE',  ( 92.32962665258456525, 83.38952084682853183, 74.36911441044827598 ) ) ;
#80663=ORIENTED_EDGE ( 'NONE', *, *, #1946, .T. ) ;
#80677=ADVANCED_FACE ( 'NONE', ( #44483 ), #37694, .T. ) ;
#80696=CARTESIAN_POINT ( 'NONE',  ( -3.968749999999949818, 120.6499999999999915, -105.4788588808462038 ) ) ;
#80706=AXIS2_PLACEMENT_3D ( 'NONE', #20764, #26073, #45583 ) ;
#80717=CARTESIAN_POINT ( 'NONE',  ( 0.000000000000000000, 92.07499999999998863, 88.90000000000000568 ) ) ;
#80727=EDGE_LOOP ( 'NONE', ( #28867, #7346, #52271, #20588 ) ) ;
#80733=CARTESIAN_POINT ( 'NONE',  ( 100.4321520267700265, 78.46444036551646661, -83.41622542100857629 ) ) ;
#80738=ORIENTED_EDGE ( 'NONE', *, *, #63709, .F. ) ;
#80757=CARTESIAN_POINT ( 'NONE',  ( -7.205548786489490269E-13, 127.0000000000000000, 103.1875000000000000 ) ) ;
#80803=CARTESIAN_POINT ( 'NONE',  ( -77.39114642429849766, 120.6499999999999915, -71.77848634863219957 ) ) ;
#80815=EDGE_CURVE ( 'NONE', #41588, #77431, #39465, .T. ) ;
#80821=DIRECTION ( 'NONE',  ( 0.000000000000000000, 1.000000000000000000, 0.000000000000000000 ) ) ;
#80826=LINE ( 'NONE', #59893, #14210 ) ;
#80850=AXIS2_PLACEMENT_3D ( 'NONE', #25018, #79558, #85487 ) ;
#80858=CARTESIAN_POINT ( 'NONE',  ( 98.05663017059093534, 92.12504059357191011, -86.19814306825418271 ) ) ;
#80889=CARTESIAN_POINT ( 'NONE',  ( -82.96293804092792357, 84.21449860606323057, 100.8069756963044341 ) ) ;
#80904=CARTESIAN_POINT ( 'NONE',  ( 0.000000000000000000, 101.5999999999999943, 0.000000000000000000 ) ) ;
#80925=EDGE_CURVE ( 'NONE', #81025, #36469, #51809, .T. ) ;
#80927=( LENGTH_UNIT ( ) NAMED_UNIT ( * ) SI_UNIT ( .MILLI., .METRE. ) );
#80937=CARTESIAN_POINT ( 'NONE',  ( -103.1875000000000000, 127.0000000000000000, 7.143749999998919797 ) ) ;
#80960=CARTESIAN_POINT ( 'NONE',  ( 98.60478223830740774, 120.6499999999999915, 3.859079674607175002E-13 ) ) ;
#80975=ADVANCED_FACE ( 'NONE', ( #20818 ), #68072, .F. ) ;
#80992=CARTESIAN_POINT ( 'NONE',  ( -3.968749999999949818, 120.6499999999999915, -105.4788588808462038 ) ) ;
#81002=CARTESIAN_POINT ( 'NONE',  ( 0.000000000000000000, 127.0000000000000000, -103.1875000000000000 ) ) ;
#81013=CARTESIAN_POINT ( 'NONE',  ( -100.6520717229718542, 79.66695435136416847, -83.15068351451320439 ) ) ;
#81016=DIRECTION ( 'NONE',  ( 0.000000000000000000, 1.000000000000000000, 0.000000000000000000 ) ) ;
#81021=DIRECTION ( 'NONE',  ( 0.000000000000000000, 0.000000000000000000, -1.000000000000000000 ) ) ;
#81025=VERTEX_POINT ( 'NONE', #77134 ) ;
#81026=ORIENTED_EDGE ( 'NONE', *, *, #20593, .T. ) ;
#81041=EDGE_LOOP ( 'NONE', ( #23868, #3183, #4095, #58990 ) ) ;
#81055=EDGE_LOOP ( 'NONE', ( #59295, #32788 ) ) ;
#81070=CARTESIAN_POINT ( 'NONE',  ( -7.205548786489490269E-13, 127.0000000000000000, 103.1875000000000000 ) ) ;
#81087=VECTOR ( 'NONE', #6010, 1000.000000000000000 ) ;
#81089=VERTEX_POINT ( 'NONE', #22179 ) ;
#81090=VERTEX_POINT ( 'NONE', #14911 ) ;
#81091=EDGE_CURVE ( 'NONE', #83626, #14127, #43476, .T. ) ;
#81104=CARTESIAN_POINT ( 'NONE',  ( -74.89042153202872498, 78.46643079253875896, 91.90737012895671398 ) ) ;
#81109=ORIENTED_EDGE ( 'NONE', *, *, #64976, .F. ) ;
#81111=VERTEX_POINT ( 'NONE', #57564 ) ;
#81120=CARTESIAN_POINT ( 'NONE',  ( 89.13693605261661901, 92.64232203292139900, 78.17042387453797403 ) ) ;
#81142=DIRECTION ( 'NONE',  ( 0.000000000000000000, 1.000000000000000000, 0.000000000000000000 ) ) ;
#81147=VERTEX_POINT ( 'NONE', #79380 ) ;
#81188=FACE_OUTER_BOUND ( 'NONE', #3680, .T. ) ;
#81194=CARTESIAN_POINT ( 'NONE',  ( 100.8594679592218171, 82.54999999999999716, -82.89895571708191824 ) ) ;
#81206=EDGE_CURVE ( 'NONE', #5947, #14550, #87966, .T. ) ;
#81220=B_SPLINE_CURVE_WITH_KNOTS ( 'NONE', 3,
 ( #13590, #69006, #34473, #76263, #21304, #9919, #44407, #65324, #37625, #17622, #1764, #45302, #78969, #43966, #3101, #52103, #58928, #72145, #30362, #29917, #9033, #23561, #86668, #24440, #37171, #23120, #57606, #44865, #51669, #73020, #64880, #17180, #51224, #50792, #10790, #23998, #31233, #30799, #58492, #2664, #86221, #79419, #84893, #71261, #72594, #10357, #58058, #63989 ),
 .UNSPECIFIED., .F., .F.,
 ( 4, 2, 2, 2, 2, 2, 2, 2, 2, 1, 2, 2, 2, 2, 2, 2, 2, 2, 2, 2, 2, 1, 2, 2, 4 ),
 ( 0.05960646776571133093, 0.06208927922045071046, 0.06333068494782040370, 0.06457209067519009693, 0.06705490212992951116, 0.06829630785729923215, 0.06953771358466893926, 0.07202052503940842287, 0.07326193076677815774, 0.07450333649414789261, 0.07574474222151762748, 0.07698614794888736235, 0.07946895940362684596, 0.08195177085836631570, 0.08319317658573605057, 0.08443458231310579931, 0.08691739376784528293, 0.08815879949521501779, 0.08940020522258475266, 0.09188301667732420852, 0.09312442240469395727, 0.09436582813206367826, 0.09560723385943342700, 0.09684863958680314799, 0.09933145104154265936 ),
 .UNSPECIFIED. ) ;
#81222=CARTESIAN_POINT ( 'NONE',  ( 117.8759966127888674, 83.38015080693121206, 12.67975824297127296 ) ) ;
#81269=AXIS2_PLACEMENT_3D ( 'NONE', #8344, #55552, #7442 ) ;
#81273=CYLINDRICAL_SURFACE ( 'NONE', #35887, 7.143750000000004263 ) ;
#81301=AXIS2_PLACEMENT_3D ( 'NONE', #35787, #88980, #55760 ) ;
#81302=CARTESIAN_POINT ( 'NONE',  ( -130.4016766882983234, 93.55256755804781221, -6.356666657630320572 ) ) ;
#81315=CARTESIAN_POINT ( 'NONE',  ( 85.31607583734475497, 90.93081950567957961, -98.82361644294707048 ) ) ;
#81354=ORIENTED_EDGE ( 'NONE', *, *, #45351, .T. ) ;
#81359=DIRECTION ( 'NONE',  ( -0.000000000000000000, -1.000000000000000000, -0.000000000000000000 ) ) ;
#81363=CARTESIAN_POINT ( 'NONE',  ( 92.32962665258612844, 82.54999999999999716, -74.36911441044637172 ) ) ;
#81377=ORIENTED_EDGE ( 'NONE', *, *, #37597, .T. ) ;
#81378=SURFACE_SIDE_STYLE ('',( #54059 ) ) ;
#81397=CONICAL_SURFACE ( 'NONE', #55212, 190.5000000000000000, 0.7853981633974300713 ) ;
#81404=B_SPLINE_CURVE_WITH_KNOTS ( 'NONE', 3,
 ( #77420, #55594, #8385, #56511, #56051, #49698, #69716, #35169, #84702, #42875, #70609, #71515, #50595, #14306, #83796, #76521, #50140, #84254, #41982, #71070, #21572, #36084, #2015, #78337, #63796 ),
 .UNSPECIFIED., .F., .F.,
 ( 4, 2, 2, 2, 2, 2, 2, 2, 2, 1, 2, 2, 4 ),
 ( 0.05959919981814688211, 0.06208050401323544909, 0.06332115611077974993, 0.06456180820832406464, 0.06704311240341262468, 0.06828376450095689776, 0.06952441659850118472, 0.07200572079358977251, 0.07324637289113407335, 0.07448702498867838806, 0.07572767708622268890, 0.07696832918376700361, 0.07944963337885561916 ),
 .UNSPECIFIED. ) ;
#81409=EDGE_CURVE ( 'NONE', #72980, #26828, #50192, .T. ) ;
#81463=CARTESIAN_POINT ( 'NONE',  ( -86.19613171056677459, 73.00415124681445889, -98.05713019660817054 ) ) ;
#81472=DIRECTION ( 'NONE',  ( 0.000000000000000000, 0.000000000000000000, 1.000000000000000000 ) ) ;
#81475=CARTESIAN_POINT ( 'NONE',  ( -12.70000000000000284, 81.72078997525719046, 117.8738102209307641 ) ) ;
#81488=DIRECTION ( 'NONE',  ( 6.982966722218760189E-15, 0.000000000000000000, -1.000000000000000000 ) ) ;
#81512=DIRECTION ( 'NONE',  ( 0.000000000000000000, 0.000000000000000000, 1.000000000000000000 ) ) ;
#81518=CARTESIAN_POINT ( 'NONE',  ( 0.000000000000000000, 92.07499999999998863, 0.000000000000000000 ) ) ;
#81521=DIRECTION ( 'NONE',  ( -3.406823656978775284E-15, 0.000000000000000000, -1.000000000000000000 ) ) ;
#81526=CARTESIAN_POINT ( 'NONE',  ( -2.883928177975681351, 94.92528396209723951, -118.5216277020858797 ) ) ;
#81558=VERTEX_POINT ( 'NONE', #44265 ) ;
#81566=CARTESIAN_POINT ( 'NONE',  ( 89.55756476669434107, 92.11680164986010766, 77.68727430815062007 ) ) ;
#81578=ADVANCED_FACE ( 'NONE', ( #73317 ), #66958, .T. ) ;
#81579=DIRECTION ( 'NONE',  ( 0.000000000000000000, 1.000000000000000000, 0.000000000000000000 ) ) ;
#81596=ORIENTED_EDGE ( 'NONE', *, *, #77993, .T. ) ;
#81613=EDGE_CURVE ( 'NONE', #66251, #2544, #16650, .T. ) ;
#81632=DIRECTION ( 'NONE',  ( -0.9659258262890686453, 0.000000000000000000, 0.2588190451025194072 ) ) ;
#81668=CARTESIAN_POINT ( 'NONE',  ( 118.3048154812336179, 92.64969027323469675, 7.744053933099116271 ) ) ;
#81718=CARTESIAN_POINT ( 'NONE',  ( 0.000000000000000000, 95.25000000000000000, 0.000000000000000000 ) ) ;
#81741=UNCERTAINTY_MEASURE_WITH_UNIT (LENGTH_MEASURE( 1.000000000000000082E-05 ), #80927, 'distance_accuracy_value', 'NONE');
#81743=CARTESIAN_POINT ( 'NONE',  ( -129.9388103550934090, 83.38002811471484677, -12.67976361810899988 ) ) ;
#81747=SHAPE_DEFINITION_REPRESENTATION ( #48474, #42769 ) ;
#81753=FACE_BOUND ( 'NONE', #4126, .T. ) ;
#81757=CARTESIAN_POINT ( 'NONE',  ( -7.760001168987765929, 72.46196594926868784, -118.3038028359265894 ) ) ;
#81760=EDGE_LOOP ( 'NONE', ( #39166, #30455, #87737, #73999 ) ) ;
#81772=ORIENTED_EDGE ( 'NONE', *, *, #65783, .T. ) ;
#81775=VECTOR ( 'NONE', #27972, 1000.000000000000000 ) ;
#81811=CARTESIAN_POINT ( 'NONE',  ( -103.1875000000000000, 127.0000000000000000, 7.937499999998919087 ) ) ;
#81812=EDGE_CURVE ( 'NONE', #37208, #27150, #43266, .T. ) ;
#81818=ORIENTED_EDGE ( 'NONE', *, *, #18381, .T. ) ;
#81836=ORIENTED_EDGE ( 'NONE', *, *, #65969, .F. ) ;
#81877=FACE_OUTER_BOUND ( 'NONE', #24764, .T. ) ;
#81894=DIRECTION ( 'NONE',  ( -1.047445008332813989E-14, 0.000000000000000000, 1.000000000000000000 ) ) ;
#81897=FACE_OUTER_BOUND ( 'NONE', #78872, .T. ) ;
#81902=CARTESIAN_POINT ( 'NONE',  ( -98.82395782888141866, 74.16976894168007561, -85.31568053864921808 ) ) ;
#81915=CARTESIAN_POINT ( 'NONE',  ( -12.61957378781718297, 80.89607376620493540, 117.8825615626982994 ) ) ;
#81929=CARTESIAN_POINT ( 'NONE',  ( 12.27452259663393086, 85.83635631587367243, 117.9189384461415813 ) ) ;
#81943=EDGE_CURVE ( 'NONE', #84780, #11327, #25701, .T. ) ;
#81944=LINE ( 'NONE', #47824, #11514 ) ;
#81961=DIRECTION ( 'NONE',  ( 0.000000000000000000, 1.000000000000000000, 0.000000000000000000 ) ) ;
#81966=CARTESIAN_POINT ( 'NONE',  ( -10.33011338239548493, 89.94938708489701185, -118.1053235025621291 ) ) ;
#82004=CARTESIAN_POINT ( 'NONE',  ( 12.61959663417972521, 80.89626266586573422, -129.9447639770759508 ) ) ;
#82008=CARTESIAN_POINT ( 'NONE',  ( 87.71185091857864791, 93.94641470820116069, 79.76397050720474624 ) ) ;
#82014=VECTOR ( 'NONE', #56087, 1000.000000000000000 ) ;
#82017=CARTESIAN_POINT ( 'NONE',  ( -82.89895571708225930, 82.54999999999999716, -100.8594679592215471 ) ) ;
#82109=VERTEX_POINT ( 'NONE', #7881 ) ;
#82123=EDGE_CURVE ( 'NONE', #72752, #19831, #52975, .T. ) ;
#82130=AXIS2_PLACEMENT_3D ( 'NONE', #63669, #36420, #75952 ) ;
#82136=EDGE_LOOP ( 'NONE', ( #41117, #2743, #18789, #36111, #66462, #50943 ) ) ;
#82150=CARTESIAN_POINT ( 'NONE',  ( -118.1261869548601453, 74.80137413886471620, -10.09682577435429529 ) ) ;
#82167=CARTESIAN_POINT ( 'NONE',  ( 72.96458098368650269, 127.0000000000000000, 72.96458098368729850 ) ) ;
#82189=AXIS2_PLACEMENT_3D ( 'NONE', #59636, #59196, #81472 ) ;
#82190=CARTESIAN_POINT ( 'NONE',  ( -129.9449521816638935, 84.21449860606323057, 12.61764002986459765 ) ) ;
#82194=ORIENTED_EDGE ( 'NONE', *, *, #72361, .F. ) ;
#82197=PRODUCT_CONTEXT ( 'NONE', #12135, 'mechanical' ) ;
#82198=CIRCLE ( 'NONE', #18294, 34.13125000000000142 ) ;
#82204=CARTESIAN_POINT ( 'NONE',  ( 84.72230615113649321, 89.94765885072622780, -99.33304294513241928 ) ) ;
#82265=LINE ( 'NONE', #7293, #85279 ) ;
#82270=CARTESIAN_POINT ( 'NONE',  ( 130.4016766882982949, 93.55256755804781221, 6.356666657631230066 ) ) ;
#82273=LINE ( 'NONE', #54954, #89732 ) ;
#82276=ORIENTED_EDGE ( 'NONE', *, *, #41293, .T. ) ;
#82277=VECTOR ( 'NONE', #25270, 1000.000000000000000 ) ;
#82297=CIRCLE ( 'NONE', #41607, 25.39999999999999858 ) ;
#82302=SURFACE_STYLE_FILL_AREA ( #34114 ) ;
#82303=DIRECTION ( 'NONE',  ( 0.000000000000000000, 1.000000000000000000, 0.000000000000000000 ) ) ;
#82310=CARTESIAN_POINT ( 'NONE',  ( 1.669011862100898913, 69.93236506402145380, 118.5470928879096562 ) ) ;
#82311=ADVANCED_FACE ( 'NONE', ( #78288 ), #72351, .F. ) ;
#82333=CARTESIAN_POINT ( 'NONE',  ( -91.73035097708734042, 69.84937019662268654, 92.90380151375066475 ) ) ;
#82353=CARTESIAN_POINT ( 'NONE',  ( -96.70122665881181945, 71.54617234588346264, -87.71474477836304118 ) ) ;
#82365=DIRECTION ( 'NONE',  ( 0.000000000000000000, 0.000000000000000000, 1.000000000000000000 ) ) ;
#82374=ORIENTED_EDGE ( 'NONE', *, *, #65756, .T. ) ;
#82377=CARTESIAN_POINT ( 'NONE',  ( 11.89031456967465594, 87.03148351030577601, 117.9583453772440151 ) ) ;
#82406=DIRECTION ( 'NONE',  ( -0.7071067811865460184, 0.000000000000000000, -0.7071067811865489050 ) ) ;
#82409=CARTESIAN_POINT ( 'NONE',  ( 9.572570118836559061, 90.93799233918605296, -118.1704038715884337 ) ) ;
#82424=VECTOR ( 'NONE', #57755, 1000.000000000000000 ) ;
#82442=CARTESIAN_POINT ( 'NONE',  ( -79.21825297796402765, 71.54629894495528220, 88.20503424218303223 ) ) ;
#82445=ORIENTED_EDGE ( 'NONE', *, *, #4315, .T. ) ;
#82455=B_SPLINE_CURVE_WITH_KNOTS ( 'NONE', 3,
 ( #84384, #8055, #56636, #27153, #55278, #28954, #22153, #41209, #40772, #34858, #14884, #28487, #48911, #83037, #76650, #49372, #48455, #55717, #21698, #68496, #62564, #63007, #62114, #82591, #41653, #789 ),
 .UNSPECIFIED., .F., .F.,
 ( 4, 2, 2, 2, 2, 2, 2, 2, 2, 2, 2, 2, 4 ),
 ( 0.01987186023414422298, 0.02111327400948154187, 0.02235468778481886076, 0.02483751533549349855, 0.02607892911083080009, 0.02732034288616810164, 0.02980317043684273595, 0.03228599798751737027, 0.03352741176285468222, 0.03476882553819198723, 0.03725165308886659726, 0.03849306686420389534, 0.03973448063954120035 ),
 .UNSPECIFIED. ) ;
#82457=EDGE_CURVE ( 'NONE', #27929, #27593, #47221, .T. ) ;
#82458=AXIS2_PLACEMENT_3D ( 'NONE', #86368, #71845, #44555 ) ;
#82461=ADVANCED_FACE ( 'NONE', ( #74571 ), #66861, .F. ) ;
#82463=EDGE_LOOP ( 'NONE', ( #27287, #15766, #11274, #83573 ) ) ;
#82468=CARTESIAN_POINT ( 'NONE',  ( -92.90667244829720062, 95.24968527363475346, -91.72735010416646162 ) ) ;
#82477=ORIENTED_EDGE ( 'NONE', *, *, #28024, .F. ) ;
#82503=CARTESIAN_POINT ( 'NONE',  ( -130.0566129357925433, 76.91670260214422683, 11.41267162807883118 ) ) ;
#82518=DIRECTION ( 'NONE',  ( 0.000000000000000000, -1.000000000000000000, 0.000000000000000000 ) ) ;
#82522=ORIENTED_EDGE ( 'NONE', *, *, #74813, .F. ) ;
#82524=AXIS2_PLACEMENT_3D ( 'NONE', #49710, #7941, #85609 ) ;
#82534=DIRECTION ( 'NONE',  ( -0.2588190451025281225, 0.000000000000000000, 0.9659258262890663138 ) ) ;
#82554=EDGE_CURVE ( 'NONE', #34288, #40430, #7334, .T. ) ;
#82562=VERTEX_POINT ( 'NONE', #55895 ) ;
#82566=DIRECTION ( 'NONE',  ( -0.2588190451025166317, 0.000000000000000000, -0.9659258262890694224 ) ) ;
#82591=CARTESIAN_POINT ( 'NONE',  ( -0.8301440424157360276, 95.22976080284065858, 118.5538265829301281 ) ) ;
#82592=CIRCLE ( 'NONE', #50666, 5.041900000000001825 ) ;
#82598=DIRECTION ( 'NONE',  ( -0.2588190451025219607, 0.000000000000000000, -0.9659258262890678681 ) ) ;
#82602=DIRECTION ( 'NONE',  ( -0.7071067811865460184, 0.000000000000000000, 0.7071067811865489050 ) ) ;
#82630=ORIENTED_EDGE ( 'NONE', *, *, #43328, .F. ) ;
#82642=DIRECTION ( 'NONE',  ( 0.000000000000000000, -1.000000000000000000, 0.000000000000000000 ) ) ;
#82644=AXIS2_PLACEMENT_3D ( 'NONE', #3002, #9821, #66103 ) ;
#82650=EDGE_CURVE ( 'NONE', #53265, #83626, #66104, .T. ) ;
#82654=CARTESIAN_POINT ( 'NONE',  ( 96.70275196374477389, 93.55256755804781221, -87.71306776503814717 ) ) ;
#82672=DIRECTION ( 'NONE',  ( -0.8660254037844379305, 0.000000000000000000, 0.5000000000000011102 ) ) ;
#82673=EDGE_LOOP ( 'NONE', ( #81818, #23266, #62334, #51413, #38891, #39921 ) ) ;
#82680=CARTESIAN_POINT ( 'NONE',  ( -118.4577320646418599, 94.30044247306076954, 4.871303722669348524 ) ) ;
#82682=CARTESIAN_POINT ( 'NONE',  ( 89.55259891852614373, 73.00424585431356661, -77.69145367648771128 ) ) ;
#82685=DIRECTION ( 'NONE',  ( 0.000000000000000000, 0.000000000000000000, -1.000000000000000000 ) ) ;
#82695=CARTESIAN_POINT ( 'NONE',  ( -12.70000000000000107, 82.54999999999999716, -129.9368274816650910 ) ) ;
#82708=ORIENTED_EDGE ( 'NONE', *, *, #7479, .F. ) ;
#82714=CARTESIAN_POINT ( 'NONE',  ( -72.96458098368751166, 127.0000000000000000, 72.96458098368620426 ) ) ;
#82720=CARTESIAN_POINT ( 'NONE',  ( 130.4018701889609133, 93.55484823631827851, -6.352633250517150110 ) ) ;
#82737=EDGE_LOOP ( 'NONE', ( #87280, #23534, #30190, #75534 ) ) ;
#82739=CARTESIAN_POINT ( 'NONE',  ( -78.17938156622513191, 72.47328848629021536, -89.12695577293565918 ) ) ;
#82754=CARTESIAN_POINT ( 'NONE',  ( 87.71474477836335382, 71.54617234588344843, -96.70122665881150681 ) ) ;
#82758=EDGE_CURVE ( 'NONE', #77844, #63421, #71369, .T. ) ;
#82759=AXIS2_PLACEMENT_3D ( 'NONE', #33502, #10815, #59404 ) ;
#82773=AXIS2_PLACEMENT_3D ( 'NONE', #5046, #32745, #4150 ) ;
#82782=CARTESIAN_POINT ( 'NONE',  ( -100.2530235599234203, 77.68489675156570229, 83.63178471058918717 ) ) ;
#82812=EDGE_LOOP ( 'NONE', ( #69571, #10528, #49155, #68996 ) ) ;
#82816=VECTOR ( 'NONE', #71612, 1000.000000000000000 ) ;
#82827=CARTESIAN_POINT ( 'NONE',  ( 0.8293608286808564767, 95.25000000000000000, 118.5560000000000258 ) ) ;
#82842=ORIENTED_EDGE ( 'NONE', *, *, #55309, .T. ) ;
#82857=CARTESIAN_POINT ( 'NONE',  ( 12.70000000000000284, 82.96441223327236969, -117.8738102209307783 ) ) ;
#82864=DIRECTION ( 'NONE',  ( 0.000000000000000000, 0.000000000000000000, 1.000000000000000000 ) ) ;
#82873=CARTESIAN_POINT ( 'NONE',  ( 77.89700433585413464, 82.54999999999999716, -59.93649209371462661 ) ) ;
#82874=DIRECTION ( 'NONE',  ( 1.000000000000000000, 0.000000000000000000, 6.878358445406130340E-15 ) ) ;
#82879=ORIENTED_EDGE ( 'NONE', *, *, #8465, .T. ) ;
#82892=ORIENTED_EDGE ( 'NONE', *, *, #6009, .T. ) ;
#82909=DIRECTION ( 'NONE',  ( 0.000000000000000000, -1.000000000000000000, 0.000000000000000000 ) ) ;
#82918=VECTOR ( 'NONE', #36620, 1000.000000000000000 ) ;
#82923=ADVANCED_FACE ( 'NONE', ( #31790 ), #52650, .F. ) ;
#82925=EDGE_CURVE ( 'NONE', #16856, #4380, #86424, .T. ) ;
#82947=CARTESIAN_POINT ( 'NONE',  ( 129.9368274816649489, 81.72130195885949888, 12.70000000000135643 ) ) ;
#82982=FACE_BOUND ( 'NONE', #7728, .T. ) ;
#82989=VERTEX_POINT ( 'NONE', #52207 ) ;
#83000=VERTEX_POINT ( 'NONE', #4985 ) ;
#83009=CARTESIAN_POINT ( 'NONE',  ( -71.77848634863190114, 127.0000000000000000, 77.39114642429879609 ) ) ;
#83033=EDGE_CURVE ( 'NONE', #33210, #29629, #19758, .T. ) ;
#83037=CARTESIAN_POINT ( 'NONE',  ( -8.387180980836955513, 92.12328101316225570, 118.2604483546762424 ) ) ;
#83043=LINE ( 'NONE', #28044, #16453 ) ;
#83052=CARTESIAN_POINT ( 'NONE',  ( 7.400192735666117905, 72.22046014531929359, -118.3253218772466511 ) ) ;
#83067=DIRECTION ( 'NONE',  ( 0.000000000000000000, 0.000000000000000000, 1.000000000000000000 ) ) ;
#83087=CARTESIAN_POINT ( 'NONE',  ( 100.4327019155579137, 78.46683822717001533, 83.41556370846579682 ) ) ;
#83109=AXIS2_PLACEMENT_3D ( 'NONE', #17068, #24328, #45192 ) ;
#83123=EDGE_CURVE ( 'NONE', #3990, #68783, #74869, .T. ) ;
#83126=CARTESIAN_POINT ( 'NONE',  ( 78.16952835488746132, 72.45860812971083931, -89.13771950014273671 ) ) ;
#83144=EDGE_CURVE ( 'NONE', #24254, #28103, #86114, .T. ) ;
#83156=FACE_OUTER_BOUND ( 'NONE', #49124, .T. ) ;
#83164=ORIENTED_EDGE ( 'NONE', *, *, #42865, .F. ) ;
#83197=CARTESIAN_POINT ( 'NONE',  ( 69.72411017813010403, 120.6499999999999915, -69.72411017812979139 ) ) ;
#83199=CARTESIAN_POINT ( 'NONE',  ( 9.554550254943340093, 74.17292945273928240, 118.1706666865833455 ) ) ;
#83217=CARTESIAN_POINT ( 'NONE',  ( -72.96458098368751166, 127.0000000000000000, 72.96458098368620426 ) ) ;
#83219=CARTESIAN_POINT ( 'NONE',  ( -94.33955404248663967, 70.17666187254641841, 90.25011051337732226 ) ) ;
#83225=DIRECTION ( 'NONE',  ( 0.000000000000000000, 1.000000000000000000, 0.000000000000000000 ) ) ;
#83232=CARTESIAN_POINT ( 'NONE',  ( -3.968749999999949818, 120.6499999999999915, -105.4788588808462038 ) ) ;
#83243=CARTESIAN_POINT ( 'NONE',  ( -86.13037352894129128, 94.82191660594813243, -81.46927207886268718 ) ) ;
#83252=EDGE_CURVE ( 'NONE', #24268, #70447, #29723, .T. ) ;
#83266=ORIENTED_EDGE ( 'NONE', *, *, #50284, .T. ) ;
#83291=LINE ( 'NONE', #1519, #15209 ) ;
#83294=CARTESIAN_POINT ( 'NONE',  ( 6.359675246477851651, 93.55082578214791056, -118.3858732848555206 ) ) ;
#83308=CARTESIAN_POINT ( 'NONE',  ( 129.9368274816649489, 82.54999999999999716, 12.70000000000136176 ) ) ;
#83315=VERTEX_POINT ( 'NONE', #18845 ) ;
#83332=FACE_OUTER_BOUND ( 'NONE', #16903, .T. ) ;
#83340=VERTEX_POINT ( 'NONE', #46966 ) ;
#83373=AXIS2_PLACEMENT_3D ( 'NONE', #30657, #11092, #58354 ) ;
#83380=DIRECTION ( 'NONE',  ( -0.5000000000000012212, 0.000000000000000000, -0.8660254037844380415 ) ) ;
#83382=CARTESIAN_POINT ( 'NONE',  ( 130.5477899301573359, 69.93364840292898066, 1.674143004590020523 ) ) ;
#83383=ORIENTED_EDGE ( 'NONE', *, *, #87016, .T. ) ;
#83395=DIRECTION ( 'NONE',  ( 0.000000000000000000, 0.000000000000000000, 1.000000000000000000 ) ) ;
#83401=DIRECTION ( 'NONE',  ( 0.000000000000000000, 1.000000000000000000, 0.000000000000000000 ) ) ;
#83402=CARTESIAN_POINT ( 'NONE',  ( 74.15067561874209900, 120.6499999999999915, 68.53801554307469246 ) ) ;
#83416=CARTESIAN_POINT ( 'NONE',  ( 103.1875000000000000, 127.0000000000000000, -7.937499999999639400 ) ) ;
#83440=CARTESIAN_POINT ( 'NONE',  ( 84.90178614994185580, 90.29814575435200652, 99.18048580889484356 ) ) ;
#83448=LINE ( 'NONE', #68020, #11291 ) ;
#83462=FACE_OUTER_BOUND ( 'NONE', #55284, .T. ) ;
#83469=DIRECTION ( 'NONE',  ( 0.000000000000000000, 1.000000000000000000, 0.000000000000000000 ) ) ;
#83480=CARTESIAN_POINT ( 'NONE',  ( 71.77848634863140376, 120.6499999999999915, -77.39114642429929347 ) ) ;
#83509=DIRECTION ( 'NONE',  ( 0.000000000000000000, 1.000000000000000000, 0.000000000000000000 ) ) ;
#83515=CARTESIAN_POINT ( 'NONE',  ( 100.5877059554732824, 79.26455342200333121, 83.22858459372999107 ) ) ;
#83524=ORIENTED_EDGE ( 'NONE', *, *, #61620, .T. ) ;
#83541=ORIENTED_EDGE ( 'NONE', *, *, #87422, .F. ) ;
#83545=AXIS2_PLACEMENT_3D ( 'NONE', #20105, #19645, #19206 ) ;
#83560=CARTESIAN_POINT ( 'NONE',  ( -87.71311422381535294, 93.94553785444269067, 79.76258624986857626 ) ) ;
#83563=CARTESIAN_POINT ( 'NONE',  ( -117.8738102209307925, 82.54999999999999716, 12.69999999999959073 ) ) ;
#83566=CARTESIAN_POINT ( 'NONE',  ( 82.65143893653623763, 69.93120980984942037, -84.99964240976891006 ) ) ;
#83573=ORIENTED_EDGE ( 'NONE', *, *, #37807, .F. ) ;
#83585=CARTESIAN_POINT ( 'NONE',  ( 75.37293521528361850, 88.18374315479975678, -91.51255889651554298 ) ) ;
#83603=VERTEX_POINT ( 'NONE', #52315 ) ;
#83608=EDGE_LOOP ( 'NONE', ( #19305, #22419 ) ) ;
#83609=VECTOR ( 'NONE', #72829, 1000.000000000000000 ) ;
#83623=CARTESIAN_POINT ( 'NONE',  ( -74.62294912200651709, 79.66725693986896317, -92.12462914090781396 ) ) ;
#83626=VERTEX_POINT ( 'NONE', #57829 ) ;
#83637=CARTESIAN_POINT ( 'NONE',  ( 84.72210942531978617, 75.15271101351807204, -99.33321048326455127 ) ) ;
#83673=FACE_OUTER_BOUND ( 'NONE', #26028, .T. ) ;
#83684=VERTEX_POINT ( 'NONE', #87775 ) ;
#83686=CARTESIAN_POINT ( 'NONE',  ( -84.90151352399661278, 74.80151635532862997, -99.18073718829371899 ) ) ;
#83687=CARTESIAN_POINT ( 'NONE',  ( -92.32962665258507684, 82.54999999999999716, -74.36911441044765070 ) ) ;
#83723=CARTESIAN_POINT ( 'NONE',  ( 72.96458098368650269, 117.4749999999999943, 72.96458098368729850 ) ) ;
#83742=CARTESIAN_POINT ( 'NONE',  ( 12.05172457139580899, 86.64129263485732224, -117.9422889837464794 ) ) ;
#83746=CARTESIAN_POINT ( 'NONE',  ( 0.000000000000000000, 95.25000000000000000, 0.000000000000000000 ) ) ;
#83766=VERTEX_POINT ( 'NONE', #68677 ) ;
#83776=CARTESIAN_POINT ( 'NONE',  ( -80.31601416995057718, 70.80054593973557076, 87.20837843453702476 ) ) ;
#83796=CARTESIAN_POINT ( 'NONE',  ( 7.759765182912740755, 72.46180059790658845, 130.3270382739332831 ) ) ;
#83801=ADVANCED_FACE ( 'NONE', ( #520 ), #34138, .F. ) ;
#83804=AXIS2_PLACEMENT_3D ( 'NONE', #8815, #17397, #31018 ) ;
#83808=ORIENTED_EDGE ( 'NONE', *, *, #35019, .F. ) ;
#83835=LINE ( 'NONE', #21610, #68959 ) ;
#83838=CARTESIAN_POINT ( 'NONE',  ( 129.9681501387582898, 79.66749569656610674, 12.37561169055549826 ) ) ;
#83903=CARTESIAN_POINT ( 'NONE',  ( 96.94208673522926745, 93.33885111288432768, 87.44839512528898240 ) ) ;
#83922=DIRECTION ( 'NONE',  ( -0.8660254037844387076, 0.000000000000000000, 0.4999999999999998890 ) ) ;
#83933=EDGE_CURVE ( 'NONE', #83315, #31262, #85902, .T. ) ;
#83943=CARTESIAN_POINT ( 'NONE',  ( 74.15067561874269586, 127.0000000000000000, -68.53801554307419508 ) ) ;
#83973=CARTESIAN_POINT ( 'NONE',  ( -3.968749999999949818, 127.0000000000000000, -105.4788588808462038 ) ) ;
#83976=CARTESIAN_POINT ( 'NONE',  ( 100.6520717229712574, 79.66695435136416847, 83.15068351451385809 ) ) ;
#83984=EDGE_CURVE ( 'NONE', #49178, #6765, #2330, .T. ) ;
#83985=EDGE_LOOP ( 'NONE', ( #24109, #15192, #740, #20794 ) ) ;
#83997=CIRCLE ( 'NONE', #28814, 34.13125000000000142 ) ;
#84011=CARTESIAN_POINT ( 'NONE',  ( -74.89049941105085395, 86.63388195152283799, 91.90730674524705535 ) ) ;
#84034=CARTESIAN_POINT ( 'NONE',  ( 88.20661029664630348, 93.55239623846826191, -79.21650378603804654 ) ) ;
#84042=LINE ( 'NONE', #3475, #9540 ) ;
#84056=AXIS2_PLACEMENT_3D ( 'NONE', #64086, #78629, #23653 ) ;
#84065=CARTESIAN_POINT ( 'NONE',  ( 2.684158038187649039E-15, 69.84999999999999432, -130.5560000000000116 ) ) ;
#84082=DIRECTION ( 'NONE',  ( 1.000000000000000000, 0.000000000000000000, 1.047445008332812253E-14 ) ) ;
#84090=CARTESIAN_POINT ( 'NONE',  ( 83.89393544538361880, 76.91670260214422683, -100.0338904447224024 ) ) ;
#84103=DIRECTION ( 'NONE',  ( -0.5000000000000003331, 0.000000000000000000, -0.8660254037844383745 ) ) ;
#84128=DIRECTION ( 'NONE',  ( 0.000000000000000000, -1.000000000000000000, 0.000000000000000000 ) ) ;
#84141=CARTESIAN_POINT ( 'NONE',  ( -74.87617104506240651, 86.64222086580517157, -91.91945768840214726 ) ) ;
#84168=LINE ( 'NONE', #71432, #76415 ) ;
#84169=EDGE_LOOP ( 'NONE', ( #15800, #1488 ) ) ;
#84180=ORIENTED_EDGE ( 'NONE', *, *, #2442, .F. ) ;
#84220=CARTESIAN_POINT ( 'NONE',  ( 72.96458098368701428, 127.0000000000000000, -80.10833098368678407 ) ) ;
#84243=CARTESIAN_POINT ( 'NONE',  ( -103.1875000000000000, 101.5999999999999943, -5.041900000001080073 ) ) ;
#84250=ORIENTED_EDGE ( 'NONE', *, *, #43562, .F. ) ;
#84254=CARTESIAN_POINT ( 'NONE',  ( 5.627553765716396761, 71.15732062108085643, 130.4351721735936280 ) ) ;
#84255=CARTESIAN_POINT ( 'NONE',  ( -98.06216817836258315, 92.11674985319542941, -86.19179098795304128 ) ) ;
#84261=DIRECTION ( 'NONE',  ( -0.2588190451025206285, 0.000000000000000000, 0.9659258262890683122 ) ) ;
#84286=EDGE_CURVE ( 'NONE', #55335, #40086, #52216, .T. ) ;
#84294=CARTESIAN_POINT ( 'NONE',  ( 0.000000000000000000, 111.1250000000000000, 0.000000000000000000 ) ) ;
#84298=CARTESIAN_POINT ( 'NONE',  ( 130.5480269016124453, 69.93117631934794076, -1.660224752217818622 ) ) ;
#84311=CARTESIAN_POINT ( 'NONE',  ( -68.53801554307499089, 120.6499999999999915, 74.15067561874188584 ) ) ;
#84315=DIRECTION ( 'NONE',  ( 1.000000000000000000, 0.000000000000000000, 0.000000000000000000 ) ) ;
#84320=VECTOR ( 'NONE', #28930, 1000.000000000000114 ) ;
#84328=ADVANCED_FACE ( 'NONE', ( #62644 ), #34482, .F. ) ;
#84335=VECTOR ( 'NONE', #44948, 1000.000000000000000 ) ;
#84341=ORIENTED_EDGE ( 'NONE', *, *, #27308, .T. ) ;
#84358=CARTESIAN_POINT ( 'NONE',  ( 87.71306776503782032, 93.55256755804781221, 96.70275196374507232 ) ) ;
#84380=EDGE_LOOP ( 'NONE', ( #47961, #54274, #44531, #16950 ) ) ;
#84384=CARTESIAN_POINT ( 'NONE',  ( -12.70000000000000107, 82.54999999999999716, 117.8738102209307641 ) ) ;
#84392=CIRCLE ( 'NONE', #29201, 188.9759999999999991 ) ;
#84393=DIRECTION ( 'NONE',  ( -0.7071067811865490160, 0.000000000000000000, -0.7071067811865461294 ) ) ;
#84407=ORIENTED_EDGE ( 'NONE', *, *, #2352, .F. ) ;
#84408=CARTESIAN_POINT ( 'NONE',  ( 103.1875000000000000, 117.4749999999999943, 3.602774393244745134E-13 ) ) ;
#84423=PLANE ( 'NONE',  #86242 ) ;
#84471=CARTESIAN_POINT ( 'NONE',  ( -77.01901799881224520, 91.23868085022589014, 90.13147184857939465 ) ) ;
#84478=CARTESIAN_POINT ( 'NONE',  ( 86.12934247706293434, 70.27763793881260312, -81.47036787067791863 ) ) ;
#84480=CARTESIAN_POINT ( 'NONE',  ( -71.77848634863190114, 120.6499999999999915, 77.39114642429879609 ) ) ;
#84491=ADVANCED_FACE ( 'NONE', ( #65335 ), #15411, .F. ) ;
#84497=CARTESIAN_POINT ( 'NONE',  ( 74.36911441044796334, 82.54999999999999716, -92.32962665258483526 ) ) ;
#84521=ORIENTED_EDGE ( 'NONE', *, *, #3964, .F. ) ;
#84522=VECTOR ( 'NONE', #51951, 1000.000000000000000 ) ;
#84524=DIRECTION ( 'NONE',  ( -3.576143065239989638E-15, 0.000000000000000000, 1.000000000000000000 ) ) ;
#84532=ORIENTED_EDGE ( 'NONE', *, *, #25582, .T. ) ;
#84543=ORIENTED_EDGE ( 'NONE', *, *, #64093, .F. ) ;
#84547=CARTESIAN_POINT ( 'NONE',  ( 91.13743891206681269, 69.93117631934792655, -93.48535127324109339 ) ) ;
#84552=VECTOR ( 'NONE', #66650, 1000.000000000000000 ) ;
#84561=ORIENTED_EDGE ( 'NONE', *, *, #61559, .F. ) ;
#84562=EDGE_CURVE ( 'NONE', #15841, #23774, #55901, .T. ) ;
#84593=CARTESIAN_POINT ( 'NONE',  ( -90.65736737572414938, 90.28416741362501341, -76.39920031718057203 ) ) ;
#84597=CARTESIAN_POINT ( 'NONE',  ( 9.720633968232110273E-16, 127.0000000000000000, -111.1250000000000000 ) ) ;
#84627=CARTESIAN_POINT ( 'NONE',  ( -6.364581335559162056, 71.52860519235655090, 130.4026037055029690 ) ) ;
#84676=EDGE_CURVE ( 'NONE', #79139, #81090, #11196, .T. ) ;
#84699=VERTEX_POINT ( 'NONE', #21217 ) ;
#84702=CARTESIAN_POINT ( 'NONE',  ( 11.02410282832817856, 76.19023921641802133, 130.0905510769329965 ) ) ;
#84703=CARTESIAN_POINT ( 'NONE',  ( -100.0339087179664830, 88.18319050751490806, -83.89391322244402716 ) ) ;
#84705=DIRECTION ( 'NONE',  ( 0.7071067811865490160, 0.000000000000000000, -0.7071067811865461294 ) ) ;
#84710=B_SPLINE_CURVE_WITH_KNOTS ( 'NONE', 3,
 ( #52496, #74768, #18450, #67952, #61132, #12097, #46138, #5282, #60673, #88412, #19361, #12547, #40233, #62922, #42466, #63379, #49288, #55634, #13442, #68852, #76565, #14346, #84298, #68409, #22068, #83382, #20707, #42025, #28866, #35666, #48828, #7076, #6623, #75673, #35211, #69753, #34319, #62025, #27510, #89759, #55186, #28402, #49738, #41570, #83838, #253, #82947, #77461 ),
 .UNSPECIFIED., .F., .F.,
 ( 4, 2, 2, 2, 2, 2, 2, 2, 2, 1, 2, 2, 2, 2, 2, 2, 2, 2, 2, 2, 2, 1, 2, 2, 4 ),
 ( 0.05959919981814688905, 0.06208168506169057382, 0.06332292768346242662, 0.06456417030523425860, 0.06704665554877799194, 0.06828789817054985167, 0.06952914079232172528, 0.07201162603586544475, 0.07325286865763730448, 0.07449411127940915034, 0.07573535390118101007, 0.07697659652295286981, 0.07945908176649658927, 0.08194156701004030874, 0.08318280963181216847, 0.08442405225358402820, 0.08690653749712774767, 0.08814778011889960740, 0.08938902274067146714, 0.09187150798421522824, 0.09311275060598708797, 0.09435399322775894770, 0.09559523584953080744, 0.09683647847130266717, 0.09931896371484640051 ),
 .UNSPECIFIED. ) ;
#84713=ORIENTED_EDGE ( 'NONE', *, *, #82758, .T. ) ;
#84716=DIRECTION ( 'NONE',  ( 0.000000000000000000, 1.000000000000000000, 0.000000000000000000 ) ) ;
#84720=EDGE_CURVE ( 'NONE', #88514, #59215, #75730, .T. ) ;
#84722=EDGE_CURVE ( 'NONE', #47173, #79701, #50215, .T. ) ;
#84731=CIRCLE ( 'NONE', #76006, 7.143750000000001599 ) ;
#84780=VERTEX_POINT ( 'NONE', #26672 ) ;
#84784=DIRECTION ( 'NONE',  ( 6.982966722218758611E-15, 0.000000000000000000, -1.000000000000000000 ) ) ;
#84788=CARTESIAN_POINT ( 'NONE',  ( 98.60478223830740774, 120.6499999999999915, 3.859079674607175002E-13 ) ) ;
#84789=EDGE_CURVE ( 'NONE', #65340, #61102, #54806, .T. ) ;
#84814=EDGE_CURVE ( 'NONE', #2062, #24255, #86484, .T. ) ;
#84830=ORIENTED_EDGE ( 'NONE', *, *, #44521, .F. ) ;
#84849=PLANE ( 'NONE',  #34457 ) ;
#84854=CARTESIAN_POINT ( 'NONE',  ( -72.96458098368600531, 127.0000000000000000, -65.02708098368781009 ) ) ;
#84856=CARTESIAN_POINT ( 'NONE',  ( -72.96458098368751166, 127.0000000000000000, 80.90208098368620426 ) ) ;
#84870=CARTESIAN_POINT ( 'NONE',  ( 72.96458098368650269, 127.0000000000000000, 72.96458098368729850 ) ) ;
#84872=ORIENTED_EDGE ( 'NONE', *, *, #32821, .T. ) ;
#84873=CARTESIAN_POINT ( 'NONE',  ( -69.72411017812909506, 120.6499999999999915, -69.72411017813089984 ) ) ;
#84890=PLANE ( 'NONE',  #44031 ) ;
#84893=CARTESIAN_POINT ( 'NONE',  ( 74.89107914305698444, 78.46407912418317210, 91.90683392111155570 ) ) ;
#84903=CARTESIAN_POINT ( 'NONE',  ( -3.968749999999949818, 127.0000000000000000, -105.4788588808462038 ) ) ;
#84914=DIRECTION ( 'NONE',  ( 1.000000000000000000, 0.000000000000000000, 6.878358445406130340E-15 ) ) ;
#84918=CARTESIAN_POINT ( 'NONE',  ( -103.1875000000000000, 127.0000000000000000, -1.080832317973422076E-12 ) ) ;
#84930=AXIS2_PLACEMENT_3D ( 'NONE', #22664, #15839, #43519 ) ;
#84940=CARTESIAN_POINT ( 'NONE',  ( 81.76533775135496285, 94.92435932957492639, -85.84941893669241608 ) ) ;
#84975=CARTESIAN_POINT ( 'NONE',  ( -72.96458098368600531, 127.0000000000000000, -72.96458098368781009 ) ) ;
#84976=EDGE_LOOP ( 'NONE', ( #20249, #80242, #4700, #16616 ) ) ;
#84981=ORIENTED_EDGE ( 'NONE', *, *, #45461, .F. ) ;
#84986=VERTEX_POINT ( 'NONE', #52389 ) ;
#84994=ORIENTED_EDGE ( 'NONE', *, *, #69483, .F. ) ;
#84995=EDGE_CURVE ( 'NONE', #27158, #28006, #24108, .T. ) ;
#84999=EDGE_CURVE ( 'NONE', #9193, #9719, #37007, .T. ) ;
#85009=CARTESIAN_POINT ( 'NONE',  ( -107.7702177616926065, 120.6499999999999915, -1.170464777364108012E-12 ) ) ;
#85013=EDGE_LOOP ( 'NONE', ( #27686, #13202, #547, #72254 ) ) ;
#85027=CARTESIAN_POINT ( 'NONE',  ( -100.7545871043104881, 84.62817240485476589, 83.02643542998036708 ) ) ;
#85037=CARTESIAN_POINT ( 'NONE',  ( -85.30119219530070040, 74.16222525595220816, -98.83784439188644910 ) ) ;
#85038=CARTESIAN_POINT ( 'NONE',  ( -89.13693605261713060, 92.64232203292144163, -78.17042387453736296 ) ) ;
#85097=CARTESIAN_POINT ( 'NONE',  ( -12.53577546185475811, 84.62767492864716701, 129.9527996235914600 ) ) ;
#85099=EDGE_CURVE ( 'NONE', #24268, #51571, #46915, .T. ) ;
#85124=PLANE ( 'NONE',  #70126 ) ;
#85126=ADVANCED_FACE ( 'NONE', ( #58765, #80139 ), #40113, .T. ) ;
#85149=CARTESIAN_POINT ( 'NONE',  ( -100.4326241145870284, 86.63355734047006251, -83.41565754067492833 ) ) ;
#85163=ORIENTED_EDGE ( 'NONE', *, *, #81943, .T. ) ;
#85191=CARTESIAN_POINT ( 'NONE',  ( -130.0912141755840992, 76.20343663217360586, -11.00834544827219652 ) ) ;
#85192=ADVANCED_FACE ( 'NONE', ( #25598 ), #51940, .F. ) ;
#85210=CARTESIAN_POINT ( 'NONE',  ( 97.46299999999996544, 82.54999999999999716, 1.020870737183004530E-12 ) ) ;
#85228=DIRECTION ( 'NONE',  ( -0.7071067811865510144, 0.000000000000000000, 0.7071067811865441310 ) ) ;
#85232=ORIENTED_EDGE ( 'NONE', *, *, #56542, .F. ) ;
#85254=AXIS2_PLACEMENT_3D ( 'NONE', #26144, #32051, #87036 ) ;
#85264=CARTESIAN_POINT ( 'NONE',  ( 103.1875000000000000, 117.4749999999999943, 7.143750000000359535 ) ) ;
#85265=VECTOR ( 'NONE', #5583, 999.9999999999998863 ) ;
#85273=LINE ( 'NONE', #15322, #42357 ) ;
#85279=VECTOR ( 'NONE', #20023, 1000.000000000000000 ) ;
#85286=EDGE_CURVE ( 'NONE', #68811, #68997, #19722, .T. ) ;
#85302=CARTESIAN_POINT ( 'NONE',  ( -98.14560000000000173, 117.4749999999999943, -1.080832317973422076E-12 ) ) ;
#85305=CARTESIAN_POINT ( 'NONE',  ( 67.35192090801830034, 120.6499999999999915, 78.57724105935551506 ) ) ;
#85316=FACE_BOUND ( 'NONE', #9091, .T. ) ;
#85334=EDGE_CURVE ( 'NONE', #36762, #81089, #55065, .T. ) ;
#85342=FACE_OUTER_BOUND ( 'NONE', #65922, .T. ) ;
#85345=CARTESIAN_POINT ( 'NONE',  ( 3.968749999999215294, 127.0000000000000000, 105.4788588808464027 ) ) ;
#85363=DIRECTION ( 'NONE',  ( 0.000000000000000000, -1.000000000000000000, 0.000000000000000000 ) ) ;
#85366=DIRECTION ( 'NONE',  ( 0.000000000000000000, 0.000000000000000000, 1.000000000000000000 ) ) ;
#85400=EDGE_CURVE ( 'NONE', #76254, #1241, #2831, .T. ) ;
#85448=CARTESIAN_POINT ( 'NONE',  ( 76.20505178924389611, 120.6499999999999915, -76.20505178924359768 ) ) ;
#85455=DIRECTION ( 'NONE',  ( 0.000000000000000000, 0.000000000000000000, 1.000000000000000000 ) ) ;
#85477=EDGE_CURVE ( 'NONE', #2816, #7755, #84168, .T. ) ;
#85480=CARTESIAN_POINT ( 'NONE',  ( -98.05663017059038111, 92.12504059357192432, 86.19814306825486483 ) ) ;
#85487=DIRECTION ( 'NONE',  ( 0.000000000000000000, 0.000000000000000000, -1.000000000000000000 ) ) ;
#85523=EDGE_LOOP ( 'NONE', ( #42917, #60092, #49411, #15177 ) ) ;
#85560=EDGE_CURVE ( 'NONE', #57775, #77970, #39120, .T. ) ;
#85561=ORIENTED_EDGE ( 'NONE', *, *, #14742, .F. ) ;
#85593=ORIENTED_EDGE ( 'NONE', *, *, #56491, .T. ) ;
#85609=DIRECTION ( 'NONE',  ( 0.000000000000000000, -1.000000000000000000, 0.000000000000000000 ) ) ;
#85635=CARTESIAN_POINT ( 'NONE',  ( 3.968749999999229949, 127.0000000000000000, 100.8961411191535973 ) ) ;
#85637=CARTESIAN_POINT ( 'NONE',  ( -130.5559380315088163, 69.85063703626890685, -0.8489233174136696647 ) ) ;
#85680=DIRECTION ( 'NONE',  ( -0.2588190451025119132, 0.000000000000000000, -0.9659258262890706437 ) ) ;
#85698=CARTESIAN_POINT ( 'NONE',  ( 75.69222284415393176, 88.91144712388911842, 91.24829632406283508 ) ) ;
#85737=DIRECTION ( 'NONE',  ( 0.000000000000000000, -1.000000000000000000, 0.000000000000000000 ) ) ;
#85743=FACE_BOUND ( 'NONE', #78722, .T. ) ;
#85746=ORIENTED_EDGE ( 'NONE', *, *, #2124, .T. ) ;
#85749=ORIENTED_EDGE ( 'NONE', *, *, #23023, .F. ) ;
#85760=CARTESIAN_POINT ( 'NONE',  ( 3.968749999999215294, 127.0000000000000000, 105.4788588808464027 ) ) ;
#85761=CARTESIAN_POINT ( 'NONE',  ( -7.205548786489490269E-13, 117.4749999999999943, 103.1875000000000000 ) ) ;
#85765=CARTESIAN_POINT ( 'NONE',  ( 33.98325472291465132, 104.3431970271542042, -3.174999999999999822 ) ) ;
#85770=ORIENTED_EDGE ( 'NONE', *, *, #62549, .F. ) ;
#85782=DIRECTION ( 'NONE',  ( -0.7071067811865510144, 0.000000000000000000, 0.7071067811865441310 ) ) ;
#85784=DIRECTION ( 'NONE',  ( 0.000000000000000000, -1.000000000000000000, 0.000000000000000000 ) ) ;
#85791=ORIENTED_EDGE ( 'NONE', *, *, #34876, .T. ) ;
#85852=CARTESIAN_POINT ( 'NONE',  ( 74.15067561874269586, 120.6499999999999915, -68.53801554307419508 ) ) ;
#85886=CARTESIAN_POINT ( 'NONE',  ( -77.39114642429849766, 127.0000000000000000, -71.77848634863219957 ) ) ;
#85893=CIRCLE ( 'NONE', #74270, 5.041900000000001825 ) ;
#85902=LINE ( 'NONE', #71376, #71825 ) ;
#85921=CARTESIAN_POINT ( 'NONE',  ( -100.8465607796065200, 83.38002811471483255, 82.91466710319213007 ) ) ;
#85924=DIRECTION ( 'NONE',  ( 0.000000000000000000, 0.000000000000000000, 1.000000000000000000 ) ) ;
#85931=ORIENTED_EDGE ( 'NONE', *, *, #24068, .T. ) ;
#85954=ORIENTED_EDGE ( 'NONE', *, *, #6920, .T. ) ;
#85967=CARTESIAN_POINT ( 'NONE',  ( -9.569027000640168978, 74.15895453169299856, 130.2061718688152610 ) ) ;
#85974=LINE ( 'NONE', #44597, #88144 ) ;
#86008=EDGE_LOOP ( 'NONE', ( #59028, #84994, #13093, #69911 ) ) ;
#86036=ORIENTED_EDGE ( 'NONE', *, *, #60049, .T. ) ;
#86055=ORIENTED_EDGE ( 'NONE', *, *, #8787, .T. ) ;
#86064=VERTEX_POINT ( 'NONE', #18120 ) ;
#86074=CARTESIAN_POINT ( 'NONE',  ( -130.4924045281959479, 70.52074417248462623, 4.093845692693608207 ) ) ;
#86084=DIRECTION ( 'NONE',  ( 0.000000000000000000, 1.000000000000000000, 0.000000000000000000 ) ) ;
#86101=DIRECTION ( 'NONE',  ( 0.9659258262890695335, 0.000000000000000000, -0.2588190451025166317 ) ) ;
#86102=DIRECTION ( 'NONE',  ( 0.000000000000000000, 1.000000000000000000, 0.000000000000000000 ) ) ;
#86114=LINE ( 'NONE', #3876, #60388 ) ;
#86118=PLANE ( 'NONE',  #10594 ) ;
#86159=ORIENTED_EDGE ( 'NONE', *, *, #82650, .T. ) ;
#86171=CARTESIAN_POINT ( 'NONE',  ( 12.70000000000000107, 82.54999999999999716, -117.8738102209307641 ) ) ;
#86186=FACE_BOUND ( 'NONE', #10920, .T. ) ;
#86199=EDGE_LOOP ( 'NONE', ( #49678, #6122 ) ) ;
#86221=CARTESIAN_POINT ( 'NONE',  ( 75.38287938184939208, 76.93600387762164416, 91.50401754987846914 ) ) ;
#86233=ADVANCED_FACE ( 'NONE', ( #5856 ), #81273, .T. ) ;
#86235=EDGE_LOOP ( 'NONE', ( #53276, #78080, #52004, #69934 ) ) ;
#86241=CARTESIAN_POINT ( 'NONE',  ( 74.15067561874209900, 120.6499999999999915, 68.53801554307469246 ) ) ;
#86242=AXIS2_PLACEMENT_3D ( 'NONE', #85765, #44386, #9440 ) ;
#86267=CIRCLE ( 'NONE', #47075, 9.525000000000000355 ) ;
#86276=DIRECTION ( 'NONE',  ( 0.000000000000000000, 1.000000000000000000, 0.000000000000000000 ) ) ;
#86311=CARTESIAN_POINT ( 'NONE',  ( 0.000000000000000000, 95.25000000000000000, 0.000000000000000000 ) ) ;
#86320=DIRECTION ( 'NONE',  ( 7.067626426349370916E-15, 0.000000000000000000, -1.000000000000000000 ) ) ;
#86328=LINE ( 'NONE', #30025, #43661 ) ;
#86349=EDGE_CURVE ( 'NONE', #70164, #38056, #71661, .T. ) ;
#86351=ORIENTED_EDGE ( 'NONE', *, *, #89114, .F. ) ;
#86368=CARTESIAN_POINT ( 'NONE',  ( -7.205548786489490269E-13, 127.0000000000000000, 103.1875000000000000 ) ) ;
#86380=FACE_BOUND ( 'NONE', #14531, .T. ) ;
#86399=ADVANCED_FACE ( 'NONE', ( #70306 ), #8992, .F. ) ;
#86419=EDGE_LOOP ( 'NONE', ( #73308, #47770, #45460, #16141, #78678, #38996, #54741, #87588, #36404, #69927 ) ) ;
#86420=APPLICATION_CONTEXT ( 'automotive_design' ) ;
#86424=CIRCLE ( 'NONE', #54538, 7.143750000000004263 ) ;
#86444=ORIENTED_EDGE ( 'NONE', *, *, #25582, .F. ) ;
#86446=ORIENTED_EDGE ( 'NONE', *, *, #84562, .T. ) ;
#86452=DIRECTION ( 'NONE',  ( -0.5000000000000003331, 0.000000000000000000, -0.8660254037844383745 ) ) ;
#86453=DIRECTION ( 'NONE',  ( -0.7071067811865439090, 0.000000000000000000, -0.7071067811865512365 ) ) ;
#86456=EDGE_CURVE ( 'NONE', #52485, #23727, #36235, .T. ) ;
#86459=ADVANCED_FACE ( 'NONE', ( #57105 ), #84849, .F. ) ;
#86461=ORIENTED_EDGE ( 'NONE', *, *, #61260, .T. ) ;
#86463=VECTOR ( 'NONE', #9714, 1000.000000000000000 ) ;
#86473=CARTESIAN_POINT ( 'NONE',  ( 117.9083666784913476, 79.66685870724428753, -12.37533002637958113 ) ) ;
#86484=CIRCLE ( 'NONE', #80706, 88.90000000000000568 ) ;
#86485=EDGE_CURVE ( 'NONE', #52873, #15453, #30123, .T. ) ;
#86501=ORIENTED_EDGE ( 'NONE', *, *, #59967, .F. ) ;
#86516=CARTESIAN_POINT ( 'NONE',  ( -130.4023353925299773, 71.53177522571070313, -6.370020420675912121 ) ) ;
#86560=CARTESIAN_POINT ( 'NONE',  ( -11.02183147610883829, 88.91382474694674443, -130.0907465706570179 ) ) ;
#86577=DIRECTION ( 'NONE',  ( -0.2588190451025166317, 0.000000000000000000, -0.9659258262890694224 ) ) ;
#86578=CARTESIAN_POINT ( 'NONE',  ( 77.69357874334650660, 92.12496802699139664, 89.55214429302449730 ) ) ;
#86582=CARTESIAN_POINT ( 'NONE',  ( 9.331435647859348646E-23, 95.25000000000000000, 130.5560000000000116 ) ) ;
#86597=DIRECTION ( 'NONE',  ( 0.000000000000000000, 0.000000000000000000, -1.000000000000000000 ) ) ;
#86599=CARTESIAN_POINT ( 'NONE',  ( -7.205548786489490269E-13, 117.4749999999999943, 96.04375000000000284 ) ) ;
#86603=EDGE_LOOP ( 'NONE', ( #8365, #82374, #14066, #45800 ) ) ;
#86624=DIRECTION ( 'NONE',  ( 0.000000000000000000, 1.000000000000000000, 0.000000000000000000 ) ) ;
#86643=DIRECTION ( 'NONE',  ( 0.000000000000000000, 0.000000000000000000, -1.000000000000000000 ) ) ;
#86652=CARTESIAN_POINT ( 'NONE',  ( 100.8594679592218597, 81.72130195885952730, -82.89895571708196087 ) ) ;
#86666=VECTOR ( 'NONE', #41972, 1000.000000000000000 ) ;
#86668=CARTESIAN_POINT ( 'NONE',  ( 84.99964240976864005, 69.93120980984940616, 82.65143893653650764 ) ) ;
#86676=CARTESIAN_POINT ( 'NONE',  ( 8.748570571408901218E-16, 127.0000000000000000, -96.04375000000000284 ) ) ;
#86681=CARTESIAN_POINT ( 'NONE',  ( 118.5215310810514922, 94.92435932957491218, -2.887881501068293666 ) ) ;
#86711=AXIS2_PLACEMENT_3D ( 'NONE', #69452, #34470, #63984 ) ;
#86714=CARTESIAN_POINT ( 'NONE',  ( -117.9582931081850745, 78.06989712577872353, 11.89083204515657677 ) ) ;
#86715=ORIENTED_EDGE ( 'NONE', *, *, #8731, .T. ) ;
#86740=CARTESIAN_POINT ( 'NONE',  ( 31.75000000000000000, 104.3431970271542042, -3.174999999999999822 ) ) ;
#86774=DIRECTION ( 'NONE',  ( 0.000000000000000000, 1.000000000000000000, 0.000000000000000000 ) ) ;
#86818=DIRECTION ( 'NONE',  ( 0.9659258262890693114, 0.000000000000000000, 0.2588190451025170757 ) ) ;
#86827=ADVANCED_FACE ( 'NONE', ( #75231 ), #46599, .F. ) ;
#86842=LINE ( 'NONE', #80937, #13811 ) ;
#86878=CARTESIAN_POINT ( 'NONE',  ( 0.000000000000000000, 125.7300000000000040, 0.000000000000000000 ) ) ;
#86901=AXIS2_PLACEMENT_3D ( 'NONE', #39986, #73618, #38207 ) ;
#86909=CARTESIAN_POINT ( 'NONE',  ( 118.4860207371917085, 70.52018178143197247, 4.092354625463673123 ) ) ;
#86949=ORIENTED_EDGE ( 'NONE', *, *, #84814, .F. ) ;
#87016=EDGE_CURVE ( 'NONE', #43994, #12205, #11438, .T. ) ;
#87017=CARTESIAN_POINT ( 'NONE',  ( 10.09455232642977052, 74.79837219561763106, -130.1659940687516723 ) ) ;
#87027=CIRCLE ( 'NONE', #17379, 5.041900000000001825 ) ;
#87036=DIRECTION ( 'NONE',  ( 0.000000000000000000, 0.000000000000000000, -1.000000000000000000 ) ) ;
#87044=FACE_OUTER_BOUND ( 'NONE', #42631, .T. ) ;
#87050=ORIENTED_EDGE ( 'NONE', *, *, #37597, .F. ) ;
#87062=FACE_OUTER_BOUND ( 'NONE', #24970, .T. ) ;
#87083=DIRECTION ( 'NONE',  ( 0.000000000000000000, 1.000000000000000000, 0.000000000000000000 ) ) ;
#87092=EDGE_LOOP ( 'NONE', ( #52713, #21339, #51583, #59749, #44131, #33757 ) ) ;
#87093=CARTESIAN_POINT ( 'NONE',  ( 0.000000000000000000, 124.9679999999999893, -25.39999999999999858 ) ) ;
#87121=ADVANCED_FACE ( 'NONE', ( #6411 ), #7760, .T. ) ;
#87129=CARTESIAN_POINT ( 'NONE',  ( 72.96458098368701428, 117.4749999999999943, -80.10833098368678407 ) ) ;
#87158=DIRECTION ( 'NONE',  ( -3.406823656978775284E-15, 0.000000000000000000, -1.000000000000000000 ) ) ;
#87175=CARTESIAN_POINT ( 'NONE',  ( 3.110602869834275287E-15, 198.8420489685532004, 25.39999999999999858 ) ) ;
#87197=DIRECTION ( 'NONE',  ( 0.000000000000000000, -1.000000000000000000, 0.000000000000000000 ) ) ;
#87201=ORIENTED_EDGE ( 'NONE', *, *, #56377, .T. ) ;
#87214=EDGE_LOOP ( 'NONE', ( #27805, #29359, #6580, #50168 ) ) ;
#87236=CARTESIAN_POINT ( 'NONE',  ( 6.802569982901797644E-16, 69.84999999999999432, 118.5560000000000116 ) ) ;
#87238=DIRECTION ( 'NONE',  ( 0.000000000000000000, 1.000000000000000000, 0.000000000000000000 ) ) ;
#87244=FACE_OUTER_BOUND ( 'NONE', #7936, .T. ) ;
#87245=PLANE ( 'NONE',  #53288 ) ;
#87260=CARTESIAN_POINT ( 'NONE',  ( 72.96458098368701428, 117.4749999999999943, -65.82083098368670449 ) ) ;
#87280=ORIENTED_EDGE ( 'NONE', *, *, #22128, .F. ) ;
#87286=DIRECTION ( 'NONE',  ( 0.000000000000000000, -1.000000000000000000, 0.000000000000000000 ) ) ;
#87287=B_SPLINE_CURVE_WITH_KNOTS ( 'NONE', 3,
 ( #59482, #65425, #3208, #24981, #52648, #78636, #16392, #44065, #71800, #2766, #46743, #26756, #54438, #80858, #25421, #19503, #82654, #54889, #33134, #25874, #4983, #47186, #20412, #48083, #60829, #19059, #53546, #40830, #47639, #13585, #88562, #13150, #74925, #74475, #41272, #19960, #75816, #81315, #74024, #82204, #5439, #69002, #53090, #26320, #67660, #68557, #53994, #18609, #39938 ),
 .UNSPECIFIED., .F., .F.,
 ( 4, 2, 2, 2, 2, 2, 2, 2, 2, 2, 2, 2, 2, 2, 2, 1, 2, 2, 2, 2, 2, 2, 2, 2, 4 ),
 ( 0.01986933033599077095, 0.02111088875730815148, 0.02235244717862553548, 0.02483556402126030002, 0.02607712244257766321, 0.02731868086389502639, 0.02980179770652973542, 0.03228491454916444792, 0.03352647297048180070, 0.03476803139179915347, 0.03725114823443387985, 0.03849270665575126732, 0.03973426507706865479, 0.04221738191970346443, 0.04345894034102086578, 0.04470049876233826713, 0.04594205718365568236, 0.04718361560497308371, 0.04966673244760788641, 0.05090829086892528776, 0.05214984929024267524, 0.05463296613287745018, 0.05587452455419482378, 0.05711608297551219737, 0.05959919981814691681 ),
 .UNSPECIFIED. ) ;
#87294=CARTESIAN_POINT ( 'NONE',  ( -74.15067561874160162, 120.6499999999999915, -68.53801554307528932 ) ) ;
#87302=PLANE ( 'NONE',  #64056 ) ;
#87308=CARTESIAN_POINT ( 'NONE',  ( 72.96458098368701428, 117.4749999999999943, -72.96458098368670164 ) ) ;
#87323=DIRECTION ( 'NONE',  ( 0.000000000000000000, -1.000000000000000000, 0.000000000000000000 ) ) ;
#87351=CARTESIAN_POINT ( 'NONE',  ( 76.20505178924339873, 120.6499999999999915, 76.20505178924419454 ) ) ;
#87355=CARTESIAN_POINT ( 'NONE',  ( 117.8827794761418204, 80.88465057165900873, -12.61751953376081303 ) ) ;
#87358=CARTESIAN_POINT ( 'NONE',  ( 7.937500000000000000, 120.6499999999999915, -103.1875000000000000 ) ) ;
#87373=EDGE_LOOP ( 'NONE', ( #18551, #67611, #56335, #21882, #84872, #81354 ) ) ;
#87378=CARTESIAN_POINT ( 'NONE',  ( 72.96458098368650269, 127.0000000000000000, 65.82083098368730134 ) ) ;
#87388=DIRECTION ( 'NONE',  ( 0.000000000000000000, -1.000000000000000000, 0.000000000000000000 ) ) ;
#87401=ORIENTED_EDGE ( 'NONE', *, *, #30535, .T. ) ;
#87422=EDGE_CURVE ( 'NONE', #7174, #78413, #23012, .T. ) ;
#87424=CARTESIAN_POINT ( 'NONE',  ( -12.70000000000000107, 82.54999999999999716, -117.8738102209307641 ) ) ;
#87434=CARTESIAN_POINT ( 'NONE',  ( -92.32962665258560264, 82.54999999999999716, 74.36911441044701121 ) ) ;
#87451=CARTESIAN_POINT ( 'NONE',  ( -74.62312585591585901, 79.66685870724428753, 92.12448541806632818 ) ) ;
#87465=CARTESIAN_POINT ( 'NONE',  ( 87.20679695024468003, 94.30044237600044710, 80.31773325845628619 ) ) ;
#87485=ORIENTED_EDGE ( 'NONE', *, *, #61859, .F. ) ;
#87495=ORIENTED_EDGE ( 'NONE', *, *, #24426, .F. ) ;
#87510=CARTESIAN_POINT ( 'NONE',  ( -100.8961411191535973, 120.6499999999999915, 3.968749999998880451 ) ) ;
#87529=EDGE_CURVE ( 'NONE', #71312, #12494, #38928, .T. ) ;
#87530=CARTESIAN_POINT ( 'NONE',  ( -103.1875000000000000, 127.0000000000000000, -1.080832317973422076E-12 ) ) ;
#87532=EDGE_CURVE ( 'NONE', #79836, #77844, #39029, .T. ) ;
#87547=ADVANCED_FACE ( 'NONE', ( #40375 ), #6752, .F. ) ;
#87551=CARTESIAN_POINT ( 'NONE',  ( -107.7702177616926065, 120.6499999999999915, -1.170464777364108012E-12 ) ) ;
#87568=CARTESIAN_POINT ( 'NONE',  ( 117.9189176348423871, 85.83559868056555331, -12.27472195321713855 ) ) ;
#87588=ORIENTED_EDGE ( 'NONE', *, *, #85099, .F. ) ;
#87601=CARTESIAN_POINT ( 'NONE',  ( -118.1708971306822917, 74.16967745525862199, 9.551705748361122517 ) ) ;
#87603=ORIENTED_EDGE ( 'NONE', *, *, #69271, .F. ) ;
#87605=DIRECTION ( 'NONE',  ( -0.7071067811865535679, 0.000000000000000000, 0.7071067811865414665 ) ) ;
#87618=AXIS2_PLACEMENT_3D ( 'NONE', #54837, #84393, #82602 ) ;
#87659=CARTESIAN_POINT ( 'NONE',  ( 108.2293999999999983, 117.4749999999999943, 3.602774393244745134E-13 ) ) ;
#87675=DIRECTION ( 'NONE',  ( 0.000000000000000000, 1.000000000000000000, 0.000000000000000000 ) ) ;
#87681=CARTESIAN_POINT ( 'NONE',  ( 0.000000000000000000, 92.07499999999998863, 38.10000000000000142 ) ) ;
#87684=CARTESIAN_POINT ( 'NONE',  ( -117.9171910823874327, 85.85031469618031963, -12.29178224785141005 ) ) ;
#87691=DIRECTION ( 'NONE',  ( 0.000000000000000000, -1.000000000000000000, 0.000000000000000000 ) ) ;
#87706=DIRECTION ( 'NONE',  ( 0.000000000000000000, 0.000000000000000000, 1.000000000000000000 ) ) ;
#87717=CARTESIAN_POINT ( 'NONE',  ( 130.5401660959919354, 95.08644067748866746, 2.073645319395265307 ) ) ;
#87733=ORIENTED_EDGE ( 'NONE', *, *, #15284, .F. ) ;
#87737=ORIENTED_EDGE ( 'NONE', *, *, #44521, .T. ) ;
#87744=DIRECTION ( 'NONE',  ( -6.982966722218760189E-15, 0.000000000000000000, 1.000000000000000000 ) ) ;
#87775=CARTESIAN_POINT ( 'NONE',  ( -33.98325472291460159, 124.5870000000000033, -3.175000000000234746 ) ) ;
#87783=DIRECTION ( 'NONE',  ( 0.000000000000000000, 0.000000000000000000, 1.000000000000000000 ) ) ;
#87798=PLANE ( 'NONE',  #10105 ) ;
#87832=FACE_OUTER_BOUND ( 'NONE', #18006, .T. ) ;
#87834=VERTEX_POINT ( 'NONE', #16265 ) ;
#87847=ADVANCED_FACE ( 'NONE', ( #22192 ), #57122, .F. ) ;
#87863=FACE_OUTER_BOUND ( 'NONE', #60864, .T. ) ;
#87922=ORIENTED_EDGE ( 'NONE', *, *, #30512, .T. ) ;
#87934=ADVANCED_FACE ( 'NONE', ( #24417 ), #72569, .T. ) ;
#87935=DIRECTION ( 'NONE',  ( -0.2588190451025246253, 0.000000000000000000, 0.9659258262890673130 ) ) ;
#87954=VERTEX_POINT ( 'NONE', #4418 ) ;
#87955=PLANE ( 'NONE',  #33655 ) ;
#87966=LINE ( 'NONE', #46603, #48954 ) ;
#87968=CARTESIAN_POINT ( 'NONE',  ( 3.174999999999889688, 104.3431970271541900, 31.75000000000000000 ) ) ;
#87990=CARTESIAN_POINT ( 'NONE',  ( 11.39408073823493872, 88.17482193101727717, -130.0579986637597187 ) ) ;
#87992=CARTESIAN_POINT ( 'NONE',  ( 100.0252357601327589, 76.93632333215536789, -83.90387289223328082 ) ) ;
#88005=AXIS2_PLACEMENT_3D ( 'NONE', #25247, #87935, #81142 ) ;
#88016=DIRECTION ( 'NONE',  ( -0.000000000000000000, 1.000000000000000000, -0.000000000000000000 ) ) ;
#88019=LINE ( 'NONE', #27578, #49113 ) ;
#88056=CARTESIAN_POINT ( 'NONE',  ( -118.5214188546241445, 70.17671898886894155, -2.891923471343901930 ) ) ;
#88073=ORIENTED_EDGE ( 'NONE', *, *, #65643, .T. ) ;
#88144=VECTOR ( 'NONE', #23743, 1000.000000000000000 ) ;
#88145=CARTESIAN_POINT ( 'NONE',  ( -117.8914297010765324, 84.62843115047674303, -12.53565398905618977 ) ) ;
#88169=CARTESIAN_POINT ( 'NONE',  ( 90.32698471909186821, 90.93965867633431799, -76.79137032886062286 ) ) ;
#88178=EDGE_CURVE ( 'NONE', #79094, #40277, #20726, .T. ) ;
#88187=SURFACE_STYLE_USAGE ( .BOTH. , #81378 ) ;
#88204=ORIENTED_EDGE ( 'NONE', *, *, #32975, .F. ) ;
#88213=CARTESIAN_POINT ( 'NONE',  ( -33.98325472291465132, 104.3431970271541900, 3.174999999999764899 ) ) ;
#88222=AXIS2_PLACEMENT_3D ( 'NONE', #80904, #81359, #39984 ) ;
#88225=CARTESIAN_POINT ( 'NONE',  ( 72.96458098368701428, 127.0000000000000000, -72.96458098368670164 ) ) ;
#88252=ORIENTED_EDGE ( 'NONE', *, *, #63417, .T. ) ;
#88264=EDGE_CURVE ( 'NONE', #47173, #18138, #36146, .T. ) ;
#88272=CARTESIAN_POINT ( 'NONE',  ( -99.33321048326486391, 75.15271101351808625, -84.72210942531944511 ) ) ;
#88299=CARTESIAN_POINT ( 'NONE',  ( -31.75000000000000000, 104.3431970271541900, -3.175000000000219647 ) ) ;
#88314=DIRECTION ( 'NONE',  ( 0.000000000000000000, -1.000000000000000000, 0.000000000000000000 ) ) ;
#88316=ORIENTED_EDGE ( 'NONE', *, *, #68053, .F. ) ;
#88355=DIRECTION ( 'NONE',  ( 0.000000000000000000, 1.000000000000000000, 0.000000000000000000 ) ) ;
#88369=CARTESIAN_POINT ( 'NONE',  ( 11.75210537873753402, 77.68270844259760111, -130.0262747911924635 ) ) ;
#88372=CARTESIAN_POINT ( 'NONE',  ( 90.81826664111963510, 89.94786999841838337, 76.20774946062938682 ) ) ;
#88380=CARTESIAN_POINT ( 'NONE',  ( -87.44900557253164664, 93.33921197991992358, -96.94152442043716178 ) ) ;
#88381=LINE ( 'NONE', #53808, #11929 ) ;
#88398=DIRECTION ( 'NONE',  ( 0.000000000000000000, 0.000000000000000000, 1.000000000000000000 ) ) ;
#88406=CYLINDRICAL_SURFACE ( 'NONE', #78665, 12.69999999999999574 ) ;
#88411=ORIENTED_EDGE ( 'NONE', *, *, #18381, .F. ) ;
#88412=CARTESIAN_POINT ( 'NONE',  ( 130.1467648208193850, 75.15271101351808625, -10.33160863867446899 ) ) ;
#88415=CIRCLE ( 'NONE', #23138, 7.937500000000000000 ) ;
#88426=LINE ( 'NONE', #40250, #59979 ) ;
#88442=CARTESIAN_POINT ( 'NONE',  ( 4.090559613967800878, 94.60197653454002875, -130.4941709638409861 ) ) ;
#88459=EDGE_CURVE ( 'NONE', #36469, #81025, #82592, .T. ) ;
#88514=VERTEX_POINT ( 'NONE', #12460 ) ;
#88530=CARTESIAN_POINT ( 'NONE',  ( 72.96458098368650269, 127.0000000000000000, 72.96458098368729850 ) ) ;
#88542=LINE ( 'NONE', #61696, #77297 ) ;
#88550=CARTESIAN_POINT ( 'NONE',  ( -130.0003666679300522, 86.63355734047007672, 12.03281245963826862 ) ) ;
#88562=CARTESIAN_POINT ( 'NONE',  ( 88.80956239834438293, 94.30053025434480674, -95.69832483115219190 ) ) ;
#88583=DIRECTION ( 'NONE',  ( 0.000000000000000000, 1.000000000000000000, 0.000000000000000000 ) ) ;
#88585=DIRECTION ( 'NONE',  ( 0.000000000000000000, 0.000000000000000000, 1.000000000000000000 ) ) ;
#88586=EDGE_LOOP ( 'NONE', ( #33331, #28977, #25898, #32522 ) ) ;
#88591=CARTESIAN_POINT ( 'NONE',  ( -83.89391322244367188, 88.18319050751492227, 100.0339087179667814 ) ) ;
#88596=DIRECTION ( 'NONE',  ( 0.000000000000000000, 1.000000000000000000, 0.000000000000000000 ) ) ;
#88614=CARTESIAN_POINT ( 'NONE',  ( 92.22587532767860807, 84.62843115047675724, -74.49778344313808986 ) ) ;
#88631=CARTESIAN_POINT ( 'NONE',  ( 130.0003666679301944, 86.63355734047007672, -12.03281245963736446 ) ) ;
#88641=CARTESIAN_POINT ( 'NONE',  ( -12.27515439545620701, 79.26608163778621474, -129.9777074703579842 ) ) ;
#88649=ORIENTED_EDGE ( 'NONE', *, *, #88982, .T. ) ;
#88658=ORIENTED_EDGE ( 'NONE', *, *, #48644, .F. ) ;
#88673=EDGE_CURVE ( 'NONE', #35668, #41448, #88415, .T. ) ;
#88681=CARTESIAN_POINT ( 'NONE',  ( 72.96458098368650269, 127.0000000000000000, 78.00648098368728256 ) ) ;
#88683=EDGE_CURVE ( 'NONE', #24180, #14963, #10084, .T. ) ;
#88695=FACE_OUTER_BOUND ( 'NONE', #86419, .T. ) ;
#88720=CYLINDRICAL_SURFACE ( 'NONE', #52807, 12.70000000000000107 ) ;
#88725=AXIS2_PLACEMENT_3D ( 'NONE', #55632, #83380, #76563 ) ;
#88757=ORIENTED_EDGE ( 'NONE', *, *, #26315, .T. ) ;
#88775=CARTESIAN_POINT ( 'NONE',  ( -12.03238568418269594, 86.63481793440480772, -117.9438919316608150 ) ) ;
#88801=AXIS2_PLACEMENT_3D ( 'NONE', #60474, #46391, #66398 ) ;
#88814=DIRECTION ( 'NONE',  ( 0.000000000000000000, 1.000000000000000000, 0.000000000000000000 ) ) ;
#88828=AXIS2_PLACEMENT_3D ( 'NONE', #2589, #43895, #16216 ) ;
#88832=ORIENTED_EDGE ( 'NONE', *, *, #32220, .T. ) ;
#88860=DIRECTION ( 'NONE',  ( 0.000000000000000000, 0.000000000000000000, -1.000000000000000000 ) ) ;
#88870=FACE_OUTER_BOUND ( 'NONE', #13266, .T. ) ;
#88888=DIRECTION ( 'NONE',  ( 0.000000000000000000, 1.000000000000000000, 0.000000000000000000 ) ) ;
#88901=EDGE_CURVE ( 'NONE', #5885, #40068, #79739, .T. ) ;
#88968=VECTOR ( 'NONE', #73644, 1000.000000000000000 ) ;
#88976=ORIENTED_EDGE ( 'NONE', *, *, #84286, .F. ) ;
#88980=DIRECTION ( 'NONE',  ( 0.000000000000000000, -1.000000000000000000, 0.000000000000000000 ) ) ;
#88982=EDGE_CURVE ( 'NONE', #8076, #36762, #29968, .T. ) ;
#88988=CARTESIAN_POINT ( 'NONE',  ( -130.2064250969985153, 90.93081950567959382, 9.551273559374726219 ) ) ;
#89020=CARTESIAN_POINT ( 'NONE',  ( 4.163101094985349692E-14, 120.6499999999999915, -107.7702177616926065 ) ) ;
#89021=ORIENTED_EDGE ( 'NONE', *, *, #10243, .F. ) ;
#89026=CARTESIAN_POINT ( 'NONE',  ( -118.5538584119706798, 95.23005795263748041, -0.8256312046391705017 ) ) ;
#89048=AXIS2_PLACEMENT_3D ( 'NONE', #31819, #87691, #33171 ) ;
#89068=CARTESIAN_POINT ( 'NONE',  ( 130.3837941446096522, 93.33921197991989516, 6.712224447895777324 ) ) ;
#89078=CARTESIAN_POINT ( 'NONE',  ( -9.275599959524004845, 73.86527412294591954, -130.2264118494045420 ) ) ;
#89084=ORIENTED_EDGE ( 'NONE', *, *, #76985, .F. ) ;
#89087=CARTESIAN_POINT ( 'NONE',  ( -81.47036787067818864, 70.27763793881258891, -86.12934247706263591 ) ) ;
#89090=DIRECTION ( 'NONE',  ( 0.000000000000000000, -1.000000000000000000, 0.000000000000000000 ) ) ;
#89106=ADVANCED_FACE ( 'NONE', ( #31737 ), #58543, .F. ) ;
#89111=CARTESIAN_POINT ( 'NONE',  ( 2.899925867002088431, 70.17843955035350234, 118.5212385615275252 ) ) ;
#89114=EDGE_CURVE ( 'NONE', #65321, #55858, #75376, .T. ) ;
#89132=PLANE ( 'NONE',  #55883 ) ;
#89135=CARTESIAN_POINT ( 'NONE',  ( -98.05713019660782948, 73.00415124681447310, 86.19613171056714407 ) ) ;
#89142=FACE_OUTER_BOUND ( 'NONE', #62546, .T. ) ;
#89152=CARTESIAN_POINT ( 'NONE',  ( -90.25011051337695278, 70.17666187254640420, -94.33955404248699494 ) ) ;
#89157=DIRECTION ( 'NONE',  ( -0.7071067811865414665, 0.000000000000000000, -0.7071067811865534569 ) ) ;
#89158=ORIENTED_EDGE ( 'NONE', *, *, #34842, .T. ) ;
#89187=ADVANCED_FACE ( 'NONE', ( #34307 ), #47476, .F. ) ;
#89211=CARTESIAN_POINT ( 'NONE',  ( 77.39114642429899504, 127.0000000000000000, 71.77848634863160271 ) ) ;
#89244=CARTESIAN_POINT ( 'NONE',  ( -74.36911441044730964, 82.54999999999999716, 92.32962665258534685 ) ) ;
#89250=B_SPLINE_CURVE_WITH_KNOTS ( 'NONE', 3,
 ( #3345, #24675, #87355, #86473, #3787, #59619, #52778, #10592, #44205, #65117, #2902, #60063, #10157, #30600, #25115, #38296, #80544, #79662, #37866, #23800, #52339, #65564, #37414, #58300, #16974, #51903, #11040, #51467, #86909, #79217, #44658, #18298, #65995, #72389, #38741, #4682, #4230, #59178, #45532, #31925, #58729, #24236, #17418, #45100, #80106, #66443, #31474, #32361 ),
 .UNSPECIFIED., .F., .F.,
 ( 4, 2, 2, 2, 2, 2, 2, 2, 2, 1, 2, 2, 2, 2, 2, 2, 2, 2, 2, 2, 2, 1, 2, 2, 4 ),
 ( 0.05960646776571126848, 0.06208927922045068964, 0.06333068494782040370, 0.06457209067519011081, 0.06705490212992956667, 0.06829630785729930154, 0.06953771358466903640, 0.07202052503940852002, 0.07326193076677825489, 0.07450333649414798975, 0.07574474222151772462, 0.07698614794888745949, 0.07946895940362692923, 0.08195177085836638509, 0.08319317658573611995, 0.08443458231310585482, 0.08691739376784532456, 0.08815879949521507331, 0.08940020522258480817, 0.09188301667732426403, 0.09312442240469397114, 0.09436582813206367826, 0.09560723385943339925, 0.09684863958680312024, 0.09933145104154257610 ),
 .UNSPECIFIED. ) ;
#89260=CARTESIAN_POINT ( 'NONE',  ( 90.31319802837550981, 90.93089219781631982, 76.80574412431096221 ) ) ;
#89265=ORIENTED_EDGE ( 'NONE', *, *, #25365, .F. ) ;
#89268=CARTESIAN_POINT ( 'NONE',  ( -83.21537498883982664, 85.85000629251470627, -100.5986936721443499 ) ) ;
#89290=VERTEX_POINT ( 'NONE', #76550 ) ;
#89306=CARTESIAN_POINT ( 'NONE',  ( -129.9777455398983079, 79.26455342200334542, 12.27475243033008212 ) ) ;
#89327=AXIS2_PLACEMENT_3D ( 'NONE', #6995, #61946, #13809 ) ;
#89340=CARTESIAN_POINT ( 'NONE',  ( 1.598849865763559337E-14, 95.25000000000000000, -130.5560000000000116 ) ) ;
#89346=VERTEX_POINT ( 'NONE', #57692 ) ;
#89351=CARTESIAN_POINT ( 'NONE',  ( -72.96458098368600531, 117.4749999999999943, -72.96458098368781009 ) ) ;
#89383=CARTESIAN_POINT ( 'NONE',  ( 33.98325472291465132, 111.1250000000000000, 3.174999999999999822 ) ) ;
#89393=LINE ( 'NONE', #75309, #22299 ) ;
#89399=CARTESIAN_POINT ( 'NONE',  ( -118.0439878494276655, 76.20320268897033600, -11.00820894928435578 ) ) ;
#89408=CARTESIAN_POINT ( 'NONE',  ( 10.79070278320184073, 75.83992121942911524, -118.0641357957730264 ) ) ;
#89439=CARTESIAN_POINT ( 'NONE',  ( 93.48535127324078076, 69.93117631934792655, 91.13743891206708270 ) ) ;
#89451=VERTEX_POINT ( 'NONE', #1850 ) ;
#89475=CIRCLE ( 'NONE', #50289, 7.937500000000000000 ) ;
#89478=AXIS2_PLACEMENT_3D ( 'NONE', #1751, #37608, #70793 ) ;
#89480=CARTESIAN_POINT ( 'NONE',  ( -118.3662777621132136, 93.33860577356858812, 6.713439888430002611 ) ) ;
#89483=CARTESIAN_POINT ( 'NONE',  ( 77.01855645442600462, 73.86197090048096925, -90.13186587200921451 ) ) ;
#89509=ORIENTED_EDGE ( 'NONE', *, *, #62194, .F. ) ;
#89522=CARTESIAN_POINT ( 'NONE',  ( 129.9681618895520216, 85.43248893795416166, -12.37548408773362674 ) ) ;
#89552=CARTESIAN_POINT ( 'NONE',  ( 89.37727808479104397, 70.52074417248462623, -95.16685018565999599 ) ) ;
#89559=CARTESIAN_POINT ( 'NONE',  ( 12.70000000000000107, 82.54999999999999716, 117.8738102209307641 ) ) ;
#89588=VERTEX_POINT ( 'NONE', #60809 ) ;
#89591=DIRECTION ( 'NONE',  ( 0.000000000000000000, 0.000000000000000000, 1.000000000000000000 ) ) ;
#89626=EDGE_CURVE ( 'NONE', #12205, #24335, #10879, .T. ) ;
#89646=EDGE_LOOP ( 'NONE', ( #82477, #73366, #50591, #71482 ) ) ;
#89655=CARTESIAN_POINT ( 'NONE',  ( 103.1875000000000000, 101.5999999999999943, 3.602774393244745134E-13 ) ) ;
#89656=CARTESIAN_POINT ( 'NONE',  ( 0.000000000000000000, 0.000000000000000000, 0.000000000000000000 ) ) ;
#89664=CARTESIAN_POINT ( 'NONE',  ( 12.59756045763256260, 84.21337188079040459, -117.8848095194957750 ) ) ;
#89696=EDGE_CURVE ( 'NONE', #73407, #35831, #7206, .T. ) ;
#89697=CARTESIAN_POINT ( 'NONE',  ( -92.32962665258561685, 81.72118090664557144, 74.36911441044701121 ) ) ;
#89700=ORIENTED_EDGE ( 'NONE', *, *, #37965, .F. ) ;
#89703=EDGE_CURVE ( 'NONE', #4701, #64147, #72592, .T. ) ;
#89704=VECTOR ( 'NONE', #11236, 1000.000000000000000 ) ;
#89723=CARTESIAN_POINT ( 'NONE',  ( -94.61838531165716404, 94.82199753261676278, -89.95770503246875194 ) ) ;
#89729=ORIENTED_EDGE ( 'NONE', *, *, #86349, .F. ) ;
#89732=VECTOR ( 'NONE', #32, 1000.000000000000227 ) ;
#89759=CARTESIAN_POINT ( 'NONE',  ( 130.0912141755840423, 76.20343663217360586, 11.00834544827310779 ) ) ;
#89761=CIRCLE ( 'NONE', #11414, 34.13125000000000142 ) ;
#89770=LINE ( 'NONE', #27081, #33362 ) ;
#89785=LINE ( 'NONE', #13029, #66912 ) ;
#89791=DIRECTION ( 'NONE',  ( 0.4999999999999995004, 0.000000000000000000, 0.8660254037844390407 ) ) ;
#89794=LINE ( 'NONE', #27547, #26867 ) ;
#89818=EDGE_CURVE ( 'NONE', #47880, #80299, #51962, .T. ) ;
#89839=ORIENTED_EDGE ( 'NONE', *, *, #58078, .T. ) ;
#89844=ORIENTED_EDGE ( 'NONE', *, *, #20254, .T. ) ;
#89862=CARTESIAN_POINT ( 'NONE',  ( 4.481911866145203760, 70.65984535152513502, -118.4718773200152384 ) ) ;
#89867=DIRECTION ( 'NONE',  ( 0.000000000000000000, 0.000000000000000000, 1.000000000000000000 ) ) ;
#89898=CARTESIAN_POINT ( 'NONE',  ( 86.93292302958541029, 72.22361908171428979, 97.40459591070944612 ) ) ;
#89906=ORIENTED_EDGE ( 'NONE', *, *, #85099, .T. ) ;
#89914=( GEOMETRIC_REPRESENTATION_CONTEXT ( 3 ) GLOBAL_UNCERTAINTY_ASSIGNED_CONTEXT ( ( #8778 ) ) GLOBAL_UNIT_ASSIGNED_CONTEXT ( ( #5078, #12346, #80497 ) ) REPRESENTATION_CONTEXT ( 'NONE', 'WORKASPACE' ) );
#89920=ORIENTED_EDGE ( 'NONE', *, *, #1168, .F. ) ;
ENDSEC;
END-ISO-10303-21;
